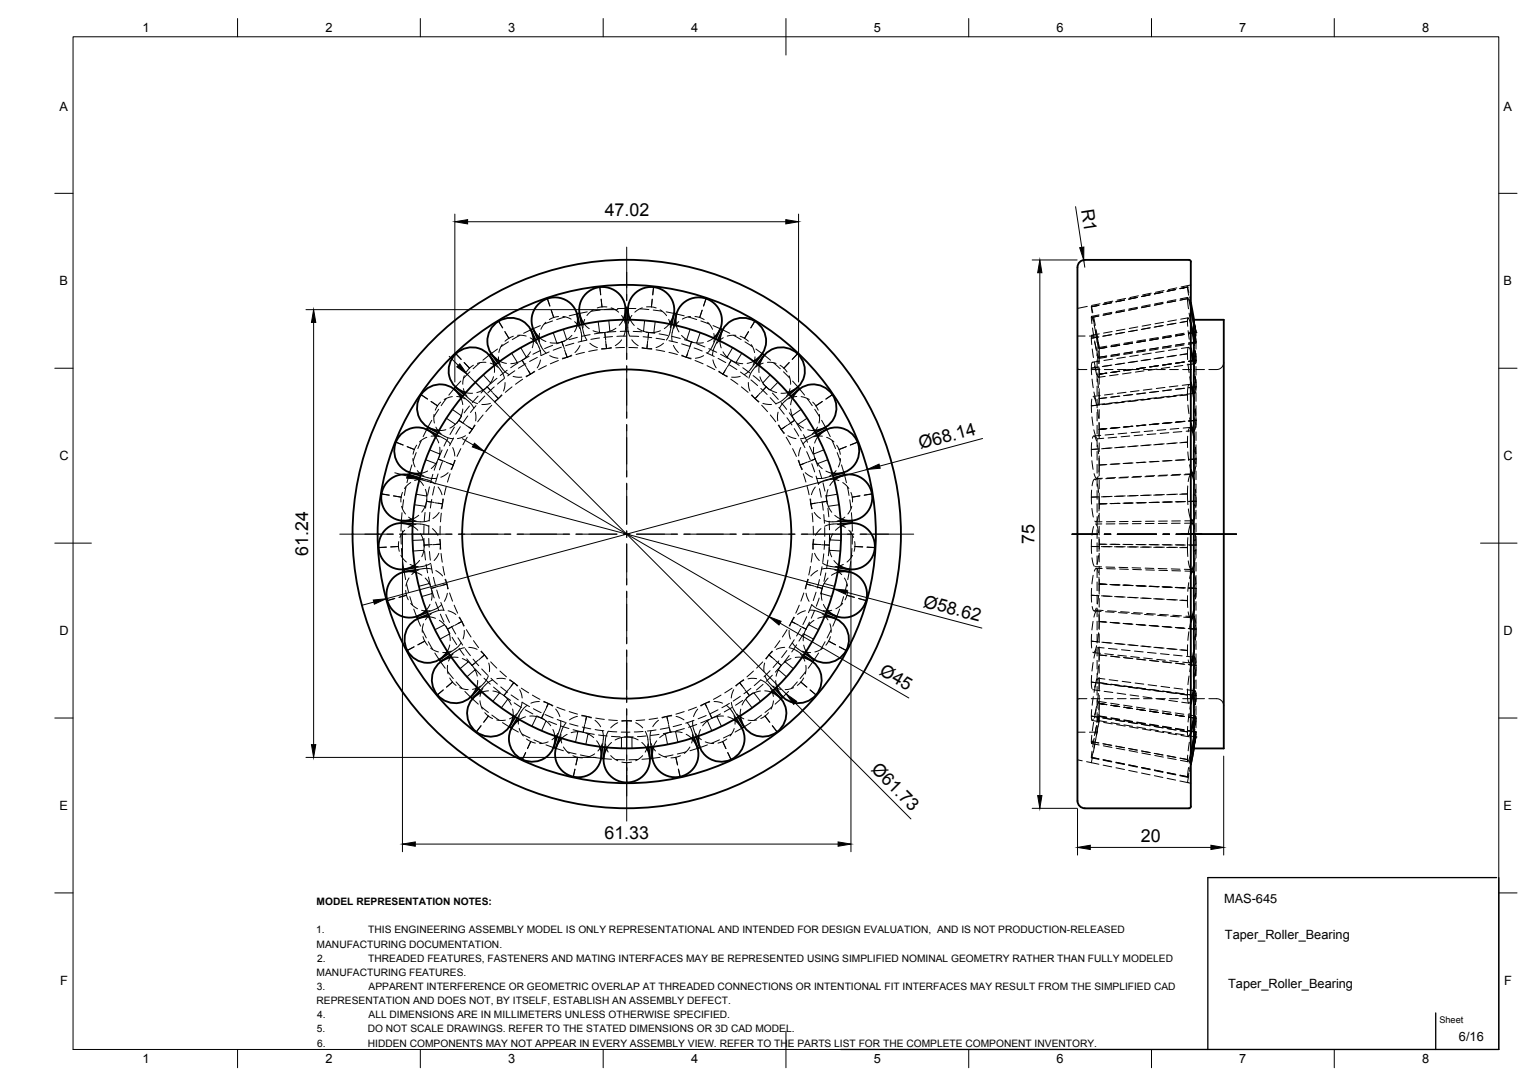
ISO-10303-21;
HEADER;
FILE_DESCRIPTION((''),'2;1');
FILE_NAME('Taper_Roller_Bearing.step','2026-10-09T10:54:55-07:00',(''),(''),'','','');
FILE_SCHEMA (('AUTOMOTIVE_DESIGN { 1 0 10303 214 3 1 1 }'));
ENDSEC;
DATA;
#10=MECHANICAL_DESIGN_GEOMETRIC_PRESENTATION_REPRESENTATION('',(#606),#63824);
#79=TOROIDAL_SURFACE('',#17489,23.5,1.) ;
#80=TOROIDAL_SURFACE('',#17493,36.5,1.) ;
#81=TOROIDAL_SURFACE('',#17497,37.25,0.25) ;
#82=TOROIDAL_SURFACE('',#17503,22.75,0.249999999999998) ;
#99=ELLIPSE('',#17336,29.1332609148258,28.6226076794831) ;
#100=ELLIPSE('',#17338,29.1332609148259,28.622607679483) ;
#101=ELLIPSE('',#17340,29.133260914826,28.6226076794829) ;
#102=ELLIPSE('',#17342,29.1332609148258,28.622607679483) ;
#103=ELLIPSE('',#17344,29.1332609148258,28.6226076794831) ;
#104=ELLIPSE('',#17346,29.1332609148257,28.6226076794832) ;
#105=ELLIPSE('',#17348,29.133260914826,28.6226076794829) ;
#106=ELLIPSE('',#17350,29.1332609148257,28.6226076794832) ;
#107=ELLIPSE('',#17353,29.1332609148258,28.622607679483) ;
#108=ELLIPSE('',#17355,29.1332609148257,28.6226076794832) ;
#109=ELLIPSE('',#17357,29.1332609148255,28.6226076794833) ;
#110=ELLIPSE('',#17359,29.1332609148258,28.6226076794831) ;
#111=ELLIPSE('',#17362,29.1332609148257,28.6226076794832) ;
#112=ELLIPSE('',#17364,29.1332609148257,28.6226076794831) ;
#113=ELLIPSE('',#17366,29.1332609148259,28.622607679483) ;
#114=ELLIPSE('',#17368,29.1332609148258,28.6226076794831) ;
#115=ELLIPSE('',#17370,29.1332609148257,28.6226076794831) ;
#116=ELLIPSE('',#17372,29.1332609148258,28.6226076794831) ;
#117=ELLIPSE('',#17374,29.1332609148258,28.6226076794831) ;
#118=ELLIPSE('',#17376,29.1332609148258,28.6226076794831) ;
#119=ELLIPSE('',#17378,29.1332609148259,28.622607679483) ;
#120=ELLIPSE('',#17380,29.1332609148258,28.622607679483) ;
#121=ELLIPSE('',#17382,29.1332609148258,28.6226076794831) ;
#122=ELLIPSE('',#17384,29.1332609148258,28.622607679483) ;
#123=ELLIPSE('',#17386,29.1332609148258,28.6226076794831) ;
#124=ELLIPSE('',#17388,29.1332609148258,28.6226076794831) ;
#125=ELLIPSE('',#17390,29.1332609148258,28.6226076794831) ;
#126=ELLIPSE('',#17392,29.1332609148258,28.6226076794831) ;
#127=ELLIPSE('',#17393,29.1332609148257,28.6226076794832) ;
#128=ELLIPSE('',#17395,29.8160190680257,29.3077933083081) ;
#129=ELLIPSE('',#17396,29.8160190680257,29.3077933083081) ;
#130=ELLIPSE('',#17397,29.8160190680257,29.3077933083081) ;
#131=ELLIPSE('',#17398,29.8160190680257,29.3077933083081) ;
#132=ELLIPSE('',#17399,29.8160190680257,29.3077933083081) ;
#133=ELLIPSE('',#17400,29.8160190680257,29.3077933083081) ;
#134=ELLIPSE('',#17401,29.8160190680257,29.3077933083081) ;
#135=ELLIPSE('',#17402,29.8160190680257,29.3077933083081) ;
#136=ELLIPSE('',#17403,29.8160190680257,29.3077933083081) ;
#137=ELLIPSE('',#17404,29.8160190680257,29.3077933083081) ;
#138=ELLIPSE('',#17405,29.8160190680257,29.3077933083081) ;
#139=ELLIPSE('',#17406,29.8160190680257,29.3077933083081) ;
#140=ELLIPSE('',#17407,29.8160190680257,29.3077933083081) ;
#141=ELLIPSE('',#17408,29.8160190680257,29.3077933083081) ;
#142=ELLIPSE('',#17409,29.8160190680257,29.3077933083081) ;
#143=ELLIPSE('',#17410,29.8160190680257,29.3077933083081) ;
#144=ELLIPSE('',#17411,29.8160190680257,29.3077933083081) ;
#145=ELLIPSE('',#17412,29.8160190680257,29.3077933083081) ;
#146=ELLIPSE('',#17413,29.8160190680257,29.3077933083081) ;
#147=ELLIPSE('',#17414,29.8160190680257,29.3077933083081) ;
#148=ELLIPSE('',#17415,29.8160190680257,29.3077933083081) ;
#149=ELLIPSE('',#17416,29.8160190680257,29.3077933083081) ;
#150=ELLIPSE('',#17417,29.8160190680257,29.3077933083081) ;
#151=ELLIPSE('',#17418,29.8160190680257,29.3077933083081) ;
#152=ELLIPSE('',#17419,29.8160190680257,29.3077933083081) ;
#153=ELLIPSE('',#17420,29.8160190680257,29.3077933083081) ;
#154=ELLIPSE('',#17421,29.8160190680257,29.3077933083082) ;
#155=ELLIPSE('',#17422,29.8160190680257,29.3077933083082) ;
#156=ELLIPSE('',#17423,29.8160190680257,29.3077933083082) ;
#157=ELLIPSE('',#17424,29.8160190680257,29.3077933083082) ;
#158=ELLIPSE('',#17425,29.8160190680257,29.3077933083081) ;
#159=ELLIPSE('',#17426,29.8160190680257,29.3077933083081) ;
#160=ELLIPSE('',#17427,29.8160190680257,29.3077933083081) ;
#161=ELLIPSE('',#17428,29.8160190680257,29.3077933083081) ;
#162=ELLIPSE('',#17429,29.8160190680257,29.3077933083081) ;
#163=ELLIPSE('',#17430,29.8160190680257,29.3077933083081) ;
#164=ELLIPSE('',#17431,29.8160190680257,29.3077933083081) ;
#165=ELLIPSE('',#17432,29.8160190680257,29.3077933083081) ;
#166=ELLIPSE('',#17433,29.8160190680257,29.3077933083081) ;
#167=ELLIPSE('',#17434,29.8160190680257,29.3077933083081) ;
#168=ELLIPSE('',#17435,29.8160190680257,29.3077933083082) ;
#169=ELLIPSE('',#17436,29.8160190680257,29.3077933083082) ;
#170=ELLIPSE('',#17437,29.8160190680257,29.3077933083081) ;
#171=ELLIPSE('',#17438,29.8160190680257,29.3077933083081) ;
#172=ELLIPSE('',#17439,29.8160190680257,29.3077933083081) ;
#173=ELLIPSE('',#17440,29.8160190680257,29.3077933083081) ;
#174=ELLIPSE('',#17441,29.8160190680257,29.3077933083081) ;
#175=ELLIPSE('',#17442,29.8160190680257,29.3077933083081) ;
#176=ELLIPSE('',#17443,29.8160190680257,29.3077933083081) ;
#177=ELLIPSE('',#17444,29.8160190680257,29.3077933083081) ;
#178=ELLIPSE('',#17445,29.8160190680257,29.3077933083081) ;
#179=ELLIPSE('',#17446,29.8160190680257,29.3077933083081) ;
#180=ELLIPSE('',#17447,29.8160190680257,29.3077933083081) ;
#181=ELLIPSE('',#17448,29.8160190680257,29.3077933083081) ;
#182=ELLIPSE('',#17449,29.8160190680257,29.3077933083082) ;
#183=ELLIPSE('',#17450,29.8160190680257,29.3077933083082) ;
#184=ELLIPSE('',#17451,29.8160190680257,29.3077933083081) ;
#185=ELLIPSE('',#17452,29.8160190680257,29.3077933083081) ;
#186=ELLIPSE('',#17457,35.9515371622909,35.3123204328217) ;
#187=ELLIPSE('',#17458,35.9515371622912,35.3123204328215) ;
#188=ELLIPSE('',#17459,35.9515371622912,35.3123204328215) ;
#189=ELLIPSE('',#17460,35.9515371622913,35.3123204328214) ;
#190=ELLIPSE('',#17461,35.951537162291,35.3123204328217) ;
#191=ELLIPSE('',#17462,35.9515371622911,35.3123204328216) ;
#192=ELLIPSE('',#17463,35.9515371622911,35.3123204328216) ;
#193=ELLIPSE('',#17464,35.9515371622911,35.3123204328216) ;
#194=ELLIPSE('',#17465,35.9515371622913,35.3123204328214) ;
#195=ELLIPSE('',#17466,35.951537162291,35.3123204328217) ;
#196=ELLIPSE('',#17467,35.9515371622912,35.3123204328215) ;
#197=ELLIPSE('',#17468,35.9515371622911,35.3123204328216) ;
#198=ELLIPSE('',#17469,35.951537162291,35.3123204328217) ;
#199=ELLIPSE('',#17470,35.9515371622913,35.3123204328214) ;
#200=ELLIPSE('',#17471,35.951537162291,35.3123204328217) ;
#201=ELLIPSE('',#17472,35.951537162291,35.3123204328217) ;
#202=ELLIPSE('',#17473,35.9515371622912,35.3123204328215) ;
#203=ELLIPSE('',#17474,35.9515371622911,35.3123204328216) ;
#204=ELLIPSE('',#17475,35.9515371622911,35.3123204328216) ;
#205=ELLIPSE('',#17476,35.951537162291,35.3123204328217) ;
#206=ELLIPSE('',#17477,35.9515371622911,35.3123204328215) ;
#207=ELLIPSE('',#17478,35.9515371622911,35.3123204328216) ;
#208=ELLIPSE('',#17479,35.9515371622913,35.3123204328214) ;
#209=ELLIPSE('',#17480,35.9515371622912,35.3123204328215) ;
#210=ELLIPSE('',#17481,35.951537162291,35.3123204328217) ;
#211=ELLIPSE('',#17482,35.9515371622911,35.3123204328216) ;
#212=ELLIPSE('',#17483,35.9515371622913,35.3123204328214) ;
#213=ELLIPSE('',#17484,35.9515371622912,35.3123204328215) ;
#214=ELLIPSE('',#17485,35.9515371622911,35.3123204328216) ;
#333=B_SPLINE_CURVE_WITH_KNOTS('',3,(#53886,#53887,#53888,#53889,#53890,
#53891,#53892,#53893,#53894,#53895,#53896,#53897,#53898,#53899,#53900,#53901,
#53902,#53903,#53904,#53905,#53906,#53907,#53908,#53909,#53910,#53911,#53912,
#53913,#53914,#53915,#53916,#53917,#53918,#53919,#53920,#53921,#53922,#53923,
#53924,#53925),.UNSPECIFIED.,.F.,.F.,(4,3,3,3,3,3,3,3,3,3,3,3,3,4),(1.39920553665769,
1.60174184009255,1.6712576734102,1.86788901812265,2.06612241242195,2.22834356454693,
2.4268269574145,2.62368336398366,2.78544130230508,2.98797174735918,3.19010175291755,
3.34253904006323,3.55341784507492,3.76429664997047),.UNSPECIFIED.) ;
#334=B_SPLINE_CURVE_WITH_KNOTS('',2,(#53927,#53928,#53929),
 .UNSPECIFIED.,.F.,.F.,(3,3),(0.,1.505093859451),.UNSPECIFIED.) ;
#335=B_SPLINE_CURVE_WITH_KNOTS('',2,(#53933,#53934,#53935),
 .UNSPECIFIED.,.F.,.F.,(3,3),(0.0815875964935672,1.58668145590164),
 .UNSPECIFIED.) ;
#336=B_SPLINE_CURVE_WITH_KNOTS('',3,(#53937,#53938,#53939,#53940,#53941,
#53942,#53943,#53944,#53945,#53946,#53947,#53948,#53949,#53950,#53951,#53952,
#53953,#53954,#53955,#53956,#53957,#53958,#53959,#53960,#53961,#53962,#53963,
#53964,#53965,#53966,#53967,#53968,#53969,#53970,#53971,#53972,#53973,#53974,
#53975,#53976),.UNSPECIFIED.,.F.,.F.,(4,3,3,3,3,3,3,3,3,3,3,3,3,4),(5.14917238118853,
5.36005118608411,5.57092999109581,5.77298643029957,5.97546031432194,6.12802772885396,
6.32462027006988,6.52281590231075,6.68512546661211,6.88364627198794,7.08054113574276,
7.24221135774884,7.44474766118475,7.51426349450141),.UNSPECIFIED.) ;
#337=B_SPLINE_CURVE_WITH_KNOTS('',3,(#53980,#53981,#53982,#53983,#53984,
#53985,#53986,#53987,#53988,#53989,#53990,#53991,#53992,#53993,#53994,#53995,
#53996,#53997,#53998,#53999,#54000,#54001,#54002,#54003,#54004,#54005,#54006,
#54007,#54008,#54009,#54010,#54011,#54012,#54013,#54014,#54015,#54016,#54017,
#54018,#54019),.UNSPECIFIED.,.F.,.F.,(4,3,3,3,3,3,3,3,3,3,3,3,3,4),(1.3992055473476,
1.60174185079187,1.6712576734102,1.86788901812146,2.06612241241944,2.22834356454693,
2.42682695741341,2.62368336398125,2.78544130230507,2.98797174735946,3.19010175291812,
3.34253904006322,3.55341784507436,3.76429664996946),.UNSPECIFIED.) ;
#338=B_SPLINE_CURVE_WITH_KNOTS('',2,(#54021,#54022,#54023),
 .UNSPECIFIED.,.F.,.F.,(3,3),(0.,1.50509385964352),.UNSPECIFIED.) ;
#339=B_SPLINE_CURVE_WITH_KNOTS('',2,(#54027,#54028,#54029),
 .UNSPECIFIED.,.F.,.F.,(3,3),(0.0815875959280614,1.58668145590161),
 .UNSPECIFIED.) ;
#340=B_SPLINE_CURVE_WITH_KNOTS('',3,(#54031,#54032,#54033,#54034,#54035,
#54036,#54037,#54038,#54039,#54040,#54041,#54042,#54043,#54044,#54045,#54046,
#54047,#54048,#54049,#54050,#54051,#54052,#54053,#54054,#54055,#54056,#54057,
#54058,#54059,#54060,#54061,#54062,#54063,#54064,#54065,#54066,#54067,#54068,
#54069,#54070),.UNSPECIFIED.,.F.,.F.,(4,3,3,3,3,3,3,3,3,3,3,3,3,4),(5.14917238118934,
5.36005118608456,5.57092999109581,5.77298643030027,5.97546031432337,6.12802772885396,
6.32462027007005,6.52281590231107,6.6851254666121,6.88364627198753,7.08054113574224,
7.24221135774884,7.44474766119323,7.51426348381142),.UNSPECIFIED.) ;
#341=B_SPLINE_CURVE_WITH_KNOTS('',3,(#54074,#54075,#54076,#54077,#54078,
#54079,#54080,#54081,#54082,#54083,#54084,#54085,#54086,#54087,#54088,#54089,
#54090,#54091,#54092,#54093,#54094,#54095,#54096,#54097,#54098,#54099,#54100,
#54101,#54102,#54103,#54104,#54105,#54106,#54107,#54108,#54109,#54110,#54111,
#54112,#54113),.UNSPECIFIED.,.F.,.F.,(4,3,3,3,3,3,3,3,3,3,3,3,3,4),(1.39920580594633,
1.60174210962102,1.6712576734102,1.86788901812167,2.06612241242011,2.22834356454693,
2.42682695741379,2.62368336398277,2.78544130230507,2.9879717473613,3.19010175292116,
3.34253904006322,3.55341784507367,3.76429664996785),.UNSPECIFIED.) ;
#342=B_SPLINE_CURVE_WITH_KNOTS('',2,(#54115,#54116,#54117),
 .UNSPECIFIED.,.F.,.F.,(3,3),(0.,1.50509385929303),.UNSPECIFIED.) ;
#343=B_SPLINE_CURVE_WITH_KNOTS('',2,(#54121,#54122,#54123),
 .UNSPECIFIED.,.F.,.F.,(3,3),(0.0815875965016897,1.5866814559016),
 .UNSPECIFIED.) ;
#344=B_SPLINE_CURVE_WITH_KNOTS('',3,(#54125,#54126,#54127,#54128,#54129,
#54130,#54131,#54132,#54133,#54134,#54135,#54136,#54137,#54138,#54139,#54140,
#54141,#54142,#54143,#54144,#54145,#54146,#54147,#54148,#54149,#54150,#54151,
#54152,#54153,#54154,#54155,#54156,#54157,#54158,#54159,#54160,#54161,#54162,
#54163,#54164),.UNSPECIFIED.,.F.,.F.,(4,3,3,3,3,3,3,3,3,3,3,3,3,4),(5.14917238119121,
5.36005118608542,5.57092999109581,5.77298643029801,5.97546031431876,6.12802772885396,
6.32462027007008,6.52281590231108,6.6851254666121,6.8836462719899,7.08054113574684,
7.24221135774884,7.44474766142535,7.51426322521267),.UNSPECIFIED.) ;
#345=B_SPLINE_CURVE_WITH_KNOTS('',3,(#54168,#54169,#54170,#54171,#54172,
#54173,#54174,#54175,#54176,#54177,#54178,#54179,#54180,#54181,#54182,#54183,
#54184,#54185,#54186,#54187,#54188,#54189,#54190,#54191,#54192,#54193,#54194,
#54195,#54196,#54197,#54198,#54199,#54200,#54201,#54202,#54203,#54204,#54205,
#54206,#54207),.UNSPECIFIED.,.F.,.F.,(4,3,3,3,3,3,3,3,3,3,3,3,3,4),(1.39920578163106,
1.60174208528522,1.67125767341019,1.86788901812004,2.06612241241701,2.22834356454693,
2.42682695741272,2.62368336398046,2.78544130230507,2.98797174735873,3.19010175291722,
3.34253904006322,3.55341784507366,3.76429664996792),.UNSPECIFIED.) ;
#346=B_SPLINE_CURVE_WITH_KNOTS('',2,(#54209,#54210,#54211),
 .UNSPECIFIED.,.F.,.F.,(3,3),(0.,1.50509385916676),.UNSPECIFIED.) ;
#347=B_SPLINE_CURVE_WITH_KNOTS('',2,(#54215,#54216,#54217),
 .UNSPECIFIED.,.F.,.F.,(3,3),(0.0815875966396183,1.58668145590158),
 .UNSPECIFIED.) ;
#348=B_SPLINE_CURVE_WITH_KNOTS('',3,(#54219,#54220,#54221,#54222,#54223,
#54224,#54225,#54226,#54227,#54228,#54229,#54230,#54231,#54232,#54233,#54234,
#54235,#54236,#54237,#54238,#54239,#54240,#54241,#54242,#54243,#54244,#54245,
#54246,#54247,#54248,#54249,#54250,#54251,#54252,#54253,#54254,#54255,#54256,
#54257,#54258),.UNSPECIFIED.,.F.,.F.,(4,3,3,3,3,3,3,3,3,3,3,3,3,4),(5.14917238119099,
5.36005118608529,5.57092999109581,5.77298643030054,5.97546031432383,6.12802772885395,
6.32462027006874,6.52281590230857,6.6851254666121,6.883646271988,7.08054113574284,
7.24221135774883,7.44474766140413,7.51426324952797),.UNSPECIFIED.) ;
#349=B_SPLINE_CURVE_WITH_KNOTS('',3,(#54262,#54263,#54264,#54265,#54266,
#54267,#54268,#54269,#54270,#54271,#54272,#54273,#54274,#54275,#54276,#54277,
#54278,#54279,#54280,#54281,#54282,#54283,#54284,#54285,#54286,#54287,#54288,
#54289,#54290,#54291,#54292,#54293,#54294,#54295,#54296,#54297,#54298,#54299,
#54300,#54301),.UNSPECIFIED.,.F.,.F.,(4,3,3,3,3,3,3,3,3,3,3,3,3,4),(1.39920580297369,
1.60174210664721,1.6712576734102,1.86788901812216,2.06612241242095,2.22834356454693,
2.42682695741258,2.62368336398087,2.78544130230508,2.98797174735879,3.19010175291683,
3.34253904006322,3.55341784507441,3.76429664996957),.UNSPECIFIED.) ;
#350=B_SPLINE_CURVE_WITH_KNOTS('',2,(#54303,#54304,#54305),
 .UNSPECIFIED.,.F.,.F.,(3,3),(0.,1.50509385957502),.UNSPECIFIED.) ;
#351=B_SPLINE_CURVE_WITH_KNOTS('',2,(#54309,#54310,#54311),
 .UNSPECIFIED.,.F.,.F.,(3,3),(0.0815875964292831,1.58668145590159),
 .UNSPECIFIED.) ;
#352=B_SPLINE_CURVE_WITH_KNOTS('',3,(#54313,#54314,#54315,#54316,#54317,
#54318,#54319,#54320,#54321,#54322,#54323,#54324,#54325,#54326,#54327,#54328,
#54329,#54330,#54331,#54332,#54333,#54334,#54335,#54336,#54337,#54338,#54339,
#54340,#54341,#54342,#54343,#54344,#54345,#54346,#54347,#54348,#54349,#54350,
#54351,#54352),.UNSPECIFIED.,.F.,.F.,(4,3,3,3,3,3,3,3,3,3,3,3,3,4),(5.14917238118972,
5.36005118608478,5.57092999109581,5.77298643029918,5.97546031432131,6.12802772885395,
6.32462027006936,6.52281590230965,6.6851254666121,6.88364627198904,7.08054113574454,
7.24221135774883,7.44474766142377,7.51426322818532),.UNSPECIFIED.) ;
#353=B_SPLINE_CURVE_WITH_KNOTS('',3,(#54356,#54357,#54358,#54359,#54360,
#54361,#54362,#54363,#54364,#54365,#54366,#54367,#54368,#54369,#54370,#54371,
#54372,#54373,#54374,#54375,#54376,#54377,#54378,#54379,#54380,#54381,#54382,
#54383,#54384,#54385,#54386,#54387,#54388,#54389,#54390,#54391,#54392,#54393,
#54394,#54395),.UNSPECIFIED.,.F.,.F.,(4,3,3,3,3,3,3,3,3,3,3,3,3,4),(1.39920556389945,
1.60174186735948,1.67125767341019,1.86788901812192,2.06612241242117,2.22834356454693,
2.426826957414,2.62368336398261,2.78544130230507,2.98797174735794,3.1901017529155,
3.34253904006322,3.55341784507408,3.76429664996891),.UNSPECIFIED.) ;
#354=B_SPLINE_CURVE_WITH_KNOTS('',2,(#54397,#54398,#54399),
 .UNSPECIFIED.,.F.,.F.,(3,3),(0.,1.50509385942592),.UNSPECIFIED.) ;
#355=B_SPLINE_CURVE_WITH_KNOTS('',2,(#54403,#54404,#54405),
 .UNSPECIFIED.,.F.,.F.,(3,3),(0.0815875963862985,1.5866814559016),
 .UNSPECIFIED.) ;
#356=B_SPLINE_CURVE_WITH_KNOTS('',3,(#54407,#54408,#54409,#54410,#54411,
#54412,#54413,#54414,#54415,#54416,#54417,#54418,#54419,#54420,#54421,#54422,
#54423,#54424,#54425,#54426,#54427,#54428,#54429,#54430,#54431,#54432,#54433,
#54434,#54435,#54436,#54437,#54438,#54439,#54440,#54441,#54442,#54443,#54444,
#54445,#54446),.UNSPECIFIED.,.F.,.F.,(4,3,3,3,3,3,3,3,3,3,3,3,3,4),(5.14917238118991,
5.36005118608483,5.57092999109581,5.77298643030024,5.97546031432328,6.12802772885395,
6.32462027006993,6.52281590231083,6.6851254666121,6.88364627199045,7.0805411357475,
7.24221135774883,7.44474766121079,7.51426346725949),.UNSPECIFIED.) ;
#357=B_SPLINE_CURVE_WITH_KNOTS('',3,(#54450,#54451,#54452,#54453,#54454,
#54455,#54456,#54457,#54458,#54459,#54460,#54461,#54462,#54463,#54464,#54465,
#54466,#54467,#54468,#54469,#54470,#54471,#54472,#54473,#54474,#54475,#54476,
#54477,#54478,#54479,#54480,#54481,#54482,#54483,#54484,#54485,#54486,#54487,
#54488,#54489),.UNSPECIFIED.,.F.,.F.,(4,3,3,3,3,3,3,3,3,3,3,3,3,4),(1.39920553665765,
1.60174184009286,1.6712576734102,1.86788901812204,2.06612241242079,2.22834356454693,
2.42682695741453,2.62368336398352,2.78544130230508,2.98797174736053,3.19010175291979,
3.34253904006323,3.55341784507441,3.76429664996951),.UNSPECIFIED.) ;
#358=B_SPLINE_CURVE_WITH_KNOTS('',2,(#54491,#54492,#54493),
 .UNSPECIFIED.,.F.,.F.,(3,3),(0.,1.50509385956687),.UNSPECIFIED.) ;
#359=B_SPLINE_CURVE_WITH_KNOTS('',2,(#54497,#54498,#54499),
 .UNSPECIFIED.,.F.,.F.,(3,3),(0.0815875965308134,1.58668145590159),
 .UNSPECIFIED.) ;
#360=B_SPLINE_CURVE_WITH_KNOTS('',3,(#54501,#54502,#54503,#54504,#54505,
#54506,#54507,#54508,#54509,#54510,#54511,#54512,#54513,#54514,#54515,#54516,
#54517,#54518,#54519,#54520,#54521,#54522,#54523,#54524,#54525,#54526,#54527,
#54528,#54529,#54530,#54531,#54532,#54533,#54534,#54535,#54536,#54537,#54538,
#54539,#54540),.UNSPECIFIED.,.F.,.F.,(4,3,3,3,3,3,3,3,3,3,3,3,3,4),(5.14917238118966,
5.36005118608471,5.57092999109581,5.77298643029994,5.9754603143227,6.12802772885396,
6.32462027006873,6.5228159023084,6.6851254666121,6.88364627198617,7.0805411357391,
7.24221135774884,7.44474766118404,7.51426349450139),.UNSPECIFIED.) ;
#361=B_SPLINE_CURVE_WITH_KNOTS('',3,(#54544,#54545,#54546,#54547,#54548,
#54549,#54550,#54551,#54552,#54553,#54554,#54555,#54556,#54557,#54558,#54559,
#54560,#54561,#54562,#54563,#54564,#54565,#54566,#54567,#54568,#54569,#54570,
#54571,#54572,#54573,#54574,#54575,#54576,#54577,#54578,#54579,#54580,#54581,
#54582,#54583),.UNSPECIFIED.,.F.,.F.,(4,3,3,3,3,3,3,3,3,3,3,3,3,4),(1.39920553665761,
1.60174184009247,1.6712576734102,1.86788901812121,2.06612241241882,2.22834356454693,
2.42682695741519,2.62368336398565,2.78544130230508,2.98797174735976,3.1901017529189,
3.34253904006323,3.55341784507426,3.76429664996931),.UNSPECIFIED.) ;
#362=B_SPLINE_CURVE_WITH_KNOTS('',2,(#54585,#54586,#54587),
 .UNSPECIFIED.,.F.,.F.,(3,3),(0.,1.50509385941839),.UNSPECIFIED.) ;
#363=B_SPLINE_CURVE_WITH_KNOTS('',2,(#54591,#54592,#54593),
 .UNSPECIFIED.,.F.,.F.,(3,3),(0.081587596231324,1.5866814559016),
 .UNSPECIFIED.) ;
#364=B_SPLINE_CURVE_WITH_KNOTS('',3,(#54595,#54596,#54597,#54598,#54599,
#54600,#54601,#54602,#54603,#54604,#54605,#54606,#54607,#54608,#54609,#54610,
#54611,#54612,#54613,#54614,#54615,#54616,#54617,#54618,#54619,#54620,#54621,
#54622,#54623,#54624,#54625,#54626,#54627,#54628,#54629,#54630,#54631,#54632,
#54633,#54634),.UNSPECIFIED.,.F.,.F.,(4,3,3,3,3,3,3,3,3,3,3,3,3,4),(5.14917238118963,
5.36005118608472,5.57092999109581,5.77298643030019,5.97546031432334,6.12802772885396,
6.32462027006835,6.52281590230765,6.68512546661211,6.88364627198795,7.08054113574254,
7.24221135774884,7.4447476611839,7.51426349450141),.UNSPECIFIED.) ;
#365=B_SPLINE_CURVE_WITH_KNOTS('',3,(#54638,#54639,#54640,#54641,#54642,
#54643,#54644,#54645,#54646,#54647,#54648,#54649,#54650,#54651,#54652,#54653,
#54654,#54655,#54656,#54657,#54658,#54659,#54660,#54661,#54662,#54663,#54664,
#54665,#54666,#54667,#54668,#54669,#54670,#54671,#54672,#54673,#54674,#54675,
#54676,#54677),.UNSPECIFIED.,.F.,.F.,(4,3,3,3,3,3,3,3,3,3,3,3,3,4),(1.39920577957092,
1.60174208322376,1.6712576734102,1.86788901812092,2.06612241241852,2.22834356454693,
2.42682695741545,2.62368336398506,2.78544130230508,2.98797174736192,3.19010175292271,
3.34253904006322,3.55341784507434,3.76429664996941),.UNSPECIFIED.) ;
#366=B_SPLINE_CURVE_WITH_KNOTS('',2,(#54679,#54680,#54681),
 .UNSPECIFIED.,.F.,.F.,(3,3),(0.,1.50509385951517),.UNSPECIFIED.) ;
#367=B_SPLINE_CURVE_WITH_KNOTS('',2,(#54685,#54686,#54687),
 .UNSPECIFIED.,.F.,.F.,(3,3),(0.0815875965974276,1.58668145590159),
 .UNSPECIFIED.) ;
#368=B_SPLINE_CURVE_WITH_KNOTS('',3,(#54689,#54690,#54691,#54692,#54693,
#54694,#54695,#54696,#54697,#54698,#54699,#54700,#54701,#54702,#54703,#54704,
#54705,#54706,#54707,#54708,#54709,#54710,#54711,#54712,#54713,#54714,#54715,
#54716,#54717,#54718,#54719,#54720,#54721,#54722,#54723,#54724,#54725,#54726,
#54727,#54728),.UNSPECIFIED.,.F.,.F.,(4,3,3,3,3,3,3,3,3,3,3,3,3,4),(5.14917238118954,
5.36005118608465,5.57092999109581,5.77298643029922,5.9754603143212,6.12802772885395,
6.32462027006964,6.52281590231008,6.6851254666121,6.88364627198796,7.0805411357427,
7.24221135774883,7.44474766140348,7.51426325158808),.UNSPECIFIED.) ;
#369=B_SPLINE_CURVE_WITH_KNOTS('',3,(#54732,#54733,#54734,#54735,#54736,
#54737,#54738,#54739,#54740,#54741,#54742,#54743,#54744,#54745,#54746,#54747,
#54748,#54749,#54750,#54751,#54752,#54753,#54754,#54755,#54756,#54757,#54758,
#54759,#54760,#54761,#54762,#54763,#54764,#54765,#54766,#54767,#54768,#54769,
#54770,#54771),.UNSPECIFIED.,.F.,.F.,(4,3,3,3,3,3,3,3,3,3,3,3,3,4),(1.39920575510034,
1.60174205873101,1.6712576734102,1.86788901812208,2.06612241242132,2.22834356454693,
2.42682695741398,2.623683363982,2.78544130230508,2.98797174735979,3.19010175291888,
3.34253904006322,3.55341784507434,3.76429664996953),.UNSPECIFIED.) ;
#370=B_SPLINE_CURVE_WITH_KNOTS('',2,(#54773,#54774,#54775),
 .UNSPECIFIED.,.F.,.F.,(3,3),(0.,1.50509385978829),.UNSPECIFIED.) ;
#371=B_SPLINE_CURVE_WITH_KNOTS('',2,(#54779,#54780,#54781),
 .UNSPECIFIED.,.F.,.F.,(3,3),(0.0815875962064005,1.58668145590161),
 .UNSPECIFIED.) ;
#372=B_SPLINE_CURVE_WITH_KNOTS('',3,(#54783,#54784,#54785,#54786,#54787,
#54788,#54789,#54790,#54791,#54792,#54793,#54794,#54795,#54796,#54797,#54798,
#54799,#54800,#54801,#54802,#54803,#54804,#54805,#54806,#54807,#54808,#54809,
#54810,#54811,#54812,#54813,#54814,#54815,#54816,#54817,#54818,#54819,#54820,
#54821,#54822),.UNSPECIFIED.,.F.,.F.,(4,3,3,3,3,3,3,3,3,3,3,3,3,4),(5.14917238118977,
5.36005118608484,5.57092999109581,5.77298643029907,5.97546031432088,6.12802772885396,
6.32462027006765,6.52281590230627,6.68512546661211,6.88364627198604,7.08054113573874,
7.24221135774884,7.44474766137677,7.51426327605873),.UNSPECIFIED.) ;
#373=B_SPLINE_CURVE_WITH_KNOTS('',3,(#54826,#54827,#54828,#54829,#54830,
#54831,#54832,#54833,#54834,#54835,#54836,#54837,#54838,#54839,#54840,#54841,
#54842,#54843,#54844,#54845,#54846,#54847,#54848,#54849,#54850,#54851,#54852,
#54853,#54854,#54855,#54856,#54857,#54858,#54859,#54860,#54861,#54862,#54863,
#54864,#54865),.UNSPECIFIED.,.F.,.F.,(4,3,3,3,3,3,3,3,3,3,3,3,3,4),(1.39920578522048,
1.60174208887688,1.6712576734102,1.86788901812355,2.06612241242382,2.22834356454693,
2.42682695741664,2.62368336398744,2.78544130230508,2.98797174736012,3.19010175291939,
3.34253904006323,3.55341784507339,3.76429664996726),.UNSPECIFIED.) ;
#374=B_SPLINE_CURVE_WITH_KNOTS('',2,(#54867,#54868,#54869),
 .UNSPECIFIED.,.F.,.F.,(3,3),(0.,1.50509385946946),.UNSPECIFIED.) ;
#375=B_SPLINE_CURVE_WITH_KNOTS('',2,(#54873,#54874,#54875),
 .UNSPECIFIED.,.F.,.F.,(3,3),(0.0815875967998225,1.58668145590156),
 .UNSPECIFIED.) ;
#376=B_SPLINE_CURVE_WITH_KNOTS('',3,(#54877,#54878,#54879,#54880,#54881,
#54882,#54883,#54884,#54885,#54886,#54887,#54888,#54889,#54890,#54891,#54892,
#54893,#54894,#54895,#54896,#54897,#54898,#54899,#54900,#54901,#54902,#54903,
#54904,#54905,#54906,#54907,#54908,#54909,#54910,#54911,#54912,#54913,#54914,
#54915,#54916),.UNSPECIFIED.,.F.,.F.,(4,3,3,3,3,3,3,3,3,3,3,3,3,4),(5.14917238119203,
5.36005118608581,5.57092999109581,5.77298643029689,5.97546031431666,6.12802772885396,
6.32462027006706,6.52281590230514,6.6851254666121,6.88364627198659,7.08054113574006,
7.24221135774884,7.44474766140431,7.51426324593851),.UNSPECIFIED.) ;
#377=B_SPLINE_CURVE_WITH_KNOTS('',3,(#54920,#54921,#54922,#54923,#54924,
#54925,#54926,#54927,#54928,#54929,#54930,#54931,#54932,#54933,#54934,#54935,
#54936,#54937,#54938,#54939,#54940,#54941,#54942,#54943,#54944,#54945,#54946,
#54947,#54948,#54949,#54950,#54951,#54952,#54953,#54954,#54955,#54956,#54957,
#54958,#54959),.UNSPECIFIED.,.F.,.F.,(4,3,3,3,3,3,3,3,3,3,3,3,3,4),(1.39920579236041,
1.6017420960232,1.6712576734102,1.86788901812226,2.06612241242125,2.22834356454693,
2.42682695741395,2.62368336398385,2.78544130230508,2.98797174735984,3.19010175291892,
3.34253904006322,3.55341784507403,3.76429664996856),.UNSPECIFIED.) ;
#378=B_SPLINE_CURVE_WITH_KNOTS('',2,(#54961,#54962,#54963),
 .UNSPECIFIED.,.F.,.F.,(3,3),(0.,1.50509385922266),.UNSPECIFIED.) ;
#379=B_SPLINE_CURVE_WITH_KNOTS('',2,(#54967,#54968,#54969),
 .UNSPECIFIED.,.F.,.F.,(3,3),(0.0815875968142298,1.58668145590157),
 .UNSPECIFIED.) ;
#380=B_SPLINE_CURVE_WITH_KNOTS('',3,(#54971,#54972,#54973,#54974,#54975,
#54976,#54977,#54978,#54979,#54980,#54981,#54982,#54983,#54984,#54985,#54986,
#54987,#54988,#54989,#54990,#54991,#54992,#54993,#54994,#54995,#54996,#54997,
#54998,#54999,#55000,#55001,#55002,#55003,#55004,#55005,#55006,#55007,#55008,
#55009,#55010),.UNSPECIFIED.,.F.,.F.,(4,3,3,3,3,3,3,3,3,3,3,3,3,4),(5.14917238119063,
5.36005118608513,5.57092999109581,5.77298643030012,5.97546031432292,6.12802772885395,
6.32462027007051,6.52281590231203,6.6851254666121,6.8836462719894,7.08054113574546,
7.24221135774883,7.44474766141017,7.51426323879855),.UNSPECIFIED.) ;
#381=B_SPLINE_CURVE_WITH_KNOTS('',3,(#55014,#55015,#55016,#55017,#55018,
#55019,#55020,#55021,#55022,#55023,#55024,#55025,#55026,#55027,#55028,#55029,
#55030,#55031,#55032,#55033,#55034,#55035,#55036,#55037,#55038,#55039,#55040,
#55041,#55042,#55043,#55044,#55045,#55046,#55047,#55048,#55049,#55050,#55051,
#55052,#55053),.UNSPECIFIED.,.F.,.F.,(4,3,3,3,3,3,3,3,3,3,3,3,3,4),(1.39920565780197,
1.6017419613437,1.6712576734102,1.86788901812192,2.06612241242043,2.22834356454693,
2.42682695741329,2.62368336398141,2.78544130230508,2.98797174735931,3.19010175291749,
3.34253904006323,3.5534178450742,3.76429664996896),.UNSPECIFIED.) ;
#382=B_SPLINE_CURVE_WITH_KNOTS('',2,(#55055,#55056,#55057),
 .UNSPECIFIED.,.F.,.F.,(3,3),(0.,1.50509385918315),.UNSPECIFIED.) ;
#383=B_SPLINE_CURVE_WITH_KNOTS('',2,(#55061,#55062,#55063),
 .UNSPECIFIED.,.F.,.F.,(3,3),(0.0815875963175643,1.58668145590161),
 .UNSPECIFIED.) ;
#384=B_SPLINE_CURVE_WITH_KNOTS('',3,(#55065,#55066,#55067,#55068,#55069,
#55070,#55071,#55072,#55073,#55074,#55075,#55076,#55077,#55078,#55079,#55080,
#55081,#55082,#55083,#55084,#55085,#55086,#55087,#55088,#55089,#55090,#55091,
#55092,#55093,#55094,#55095,#55096,#55097,#55098,#55099,#55100,#55101,#55102,
#55103,#55104),.UNSPECIFIED.,.F.,.F.,(4,3,3,3,3,3,3,3,3,3,3,3,3,4),(5.14917238118996,
5.36005118608481,5.57092999109581,5.77298643029938,5.97546031432158,6.12802772885396,
6.32462027006706,6.52281590230528,6.68512546661211,6.88364627198969,7.08054113574575,
7.24221135774884,7.44474766128961,7.51426337335708),.UNSPECIFIED.) ;
#385=B_SPLINE_CURVE_WITH_KNOTS('',3,(#55108,#55109,#55110,#55111,#55112,
#55113,#55114,#55115,#55116,#55117,#55118,#55119,#55120,#55121,#55122,#55123,
#55124,#55125,#55126,#55127,#55128,#55129,#55130,#55131,#55132,#55133,#55134,
#55135,#55136,#55137,#55138,#55139,#55140,#55141,#55142,#55143,#55144,#55145,
#55146,#55147),.UNSPECIFIED.,.F.,.F.,(4,3,3,3,3,3,3,3,3,3,3,3,3,4),(1.39920626730384,
1.60174256547371,1.6712576734102,1.86788901812253,2.06612241242136,2.22834356454693,
2.42682695741533,2.62368336398524,2.78544130230508,2.9879717473591,3.19010175291799,
3.34253904006322,3.55341784507403,3.76429664996862),.UNSPECIFIED.) ;
#386=B_SPLINE_CURVE_WITH_KNOTS('',2,(#55149,#55150,#55151),
 .UNSPECIFIED.,.F.,.F.,(3,3),(0.,1.50509385974731),.UNSPECIFIED.) ;
#387=B_SPLINE_CURVE_WITH_KNOTS('',2,(#55155,#55156,#55157),
 .UNSPECIFIED.,.F.,.F.,(3,3),(0.081587596220629,1.58668145590162),
 .UNSPECIFIED.) ;
#388=B_SPLINE_CURVE_WITH_KNOTS('',3,(#55159,#55160,#55161,#55162,#55163,
#55164,#55165,#55166,#55167,#55168,#55169,#55170,#55171,#55172,#55173,#55174,
#55175,#55176,#55177,#55178,#55179,#55180,#55181,#55182,#55183,#55184,#55185,
#55186,#55187,#55188,#55189,#55190,#55191,#55192,#55193,#55194,#55195,#55196,
#55197,#55198),.UNSPECIFIED.,.F.,.F.,(4,3,3,3,3,3,3,3,3,3,3,3,3,4),(5.14917238119046,
5.36005118608503,5.57092999109581,5.77298643030045,5.97546031432374,6.12802772885396,
6.32462027006966,6.52281590231019,6.6851254666121,6.88364627198813,7.08054113574297,
7.24221135774884,7.44474766183158,7.51426276518474),.UNSPECIFIED.) ;
#389=B_SPLINE_CURVE_WITH_KNOTS('',3,(#55202,#55203,#55204,#55205,#55206,
#55207,#55208,#55209,#55210,#55211,#55212,#55213,#55214,#55215,#55216,#55217,
#55218,#55219,#55220,#55221,#55222,#55223,#55224,#55225,#55226,#55227,#55228,
#55229,#55230,#55231,#55232,#55233,#55234,#55235,#55236,#55237,#55238,#55239,
#55240,#55241),.UNSPECIFIED.,.F.,.F.,(4,3,3,3,3,3,3,3,3,3,3,3,3,4),(1.39920553665763,
1.60174184009342,1.6712576734102,1.86788901812086,2.06612241241843,2.22834356454693,
2.42682695741443,2.62368336398377,2.78544130230508,2.98797174735924,3.19010175291802,
3.34253904006322,3.55341784507355,3.76429664996775),.UNSPECIFIED.) ;
#390=B_SPLINE_CURVE_WITH_KNOTS('',2,(#55243,#55244,#55245),
 .UNSPECIFIED.,.F.,.F.,(3,3),(0.,1.50509385940246),.UNSPECIFIED.) ;
#391=B_SPLINE_CURVE_WITH_KNOTS('',2,(#55249,#55250,#55251),
 .UNSPECIFIED.,.F.,.F.,(3,3),(0.0815875964990715,1.58668145590159),
 .UNSPECIFIED.) ;
#392=B_SPLINE_CURVE_WITH_KNOTS('',3,(#55253,#55254,#55255,#55256,#55257,
#55258,#55259,#55260,#55261,#55262,#55263,#55264,#55265,#55266,#55267,#55268,
#55269,#55270,#55271,#55272,#55273,#55274,#55275,#55276,#55277,#55278,#55279,
#55280,#55281,#55282,#55283,#55284,#55285,#55286,#55287,#55288,#55289,#55290,
#55291,#55292),.UNSPECIFIED.,.F.,.F.,(4,3,3,3,3,3,3,3,3,3,3,3,3,4),(5.14917238119122,
5.36005118608543,5.57092999109581,5.77298643029924,5.97546031432136,6.12802772885395,
6.32462027006939,6.52281590230979,6.6851254666121,6.88364627198772,7.08054113574227,
7.24221135774883,7.44474766118609,7.5142634945014),.UNSPECIFIED.) ;
#393=B_SPLINE_CURVE_WITH_KNOTS('',3,(#55296,#55297,#55298,#55299,#55300,
#55301,#55302,#55303,#55304,#55305,#55306,#55307,#55308,#55309,#55310,#55311,
#55312,#55313,#55314,#55315,#55316,#55317,#55318,#55319,#55320,#55321,#55322,
#55323,#55324,#55325,#55326,#55327,#55328,#55329,#55330,#55331,#55332,#55333,
#55334,#55335),.UNSPECIFIED.,.F.,.F.,(4,3,3,3,3,3,3,3,3,3,3,3,3,4),(1.39920626597427,
1.60174256547503,1.6712576734102,1.86788901812092,2.06612241241852,2.22834356454693,
2.4268269574154,2.62368336398519,2.78544130230508,2.98797174735909,3.19010175291677,
3.34253904006322,3.55341784507445,3.76429664996961),.UNSPECIFIED.) ;
#394=B_SPLINE_CURVE_WITH_KNOTS('',2,(#55337,#55338,#55339),
 .UNSPECIFIED.,.F.,.F.,(3,3),(0.,1.50509385919341),.UNSPECIFIED.) ;
#395=B_SPLINE_CURVE_WITH_KNOTS('',2,(#55343,#55344,#55345),
 .UNSPECIFIED.,.F.,.F.,(3,3),(0.0815875964645715,1.58668145590163),
 .UNSPECIFIED.) ;
#396=B_SPLINE_CURVE_WITH_KNOTS('',3,(#55347,#55348,#55349,#55350,#55351,
#55352,#55353,#55354,#55355,#55356,#55357,#55358,#55359,#55360,#55361,#55362,
#55363,#55364,#55365,#55366,#55367,#55368,#55369,#55370,#55371,#55372,#55373,
#55374,#55375,#55376,#55377,#55378,#55379,#55380,#55381,#55382,#55383,#55384,
#55385,#55386),.UNSPECIFIED.,.F.,.F.,(4,3,3,3,3,3,3,3,3,3,3,3,3,4),(5.14917238118938,
5.36005118608458,5.57092999109581,5.77298643029965,5.97546031432214,6.12802772885396,
6.32462027006888,6.5228159023088,6.6851254666121,6.88364627198861,7.0805411357444,
7.24221135774884,7.44474766183236,7.51426276385522),.UNSPECIFIED.) ;
#397=B_SPLINE_CURVE_WITH_KNOTS('',3,(#55390,#55391,#55392,#55393,#55394,
#55395,#55396,#55397,#55398,#55399,#55400,#55401,#55402,#55403,#55404,#55405,
#55406,#55407,#55408,#55409,#55410,#55411,#55412,#55413,#55414,#55415,#55416,
#55417,#55418,#55419,#55420,#55421,#55422,#55423,#55424,#55425,#55426,#55427,
#55428,#55429),.UNSPECIFIED.,.F.,.F.,(4,3,3,3,3,3,3,3,3,3,3,3,3,4),(1.39920565780197,
1.60174196134636,1.6712576734102,1.86788901812062,2.06612241241771,2.22834356454693,
2.42682695741333,2.62368336398205,2.78544130230508,2.98797174735987,3.19010175291831,
3.34253904006323,3.55341784507432,3.76429664996955),.UNSPECIFIED.) ;
#398=B_SPLINE_CURVE_WITH_KNOTS('',2,(#55431,#55432,#55433),
 .UNSPECIFIED.,.F.,.F.,(3,3),(0.,1.50509385959389),.UNSPECIFIED.) ;
#399=B_SPLINE_CURVE_WITH_KNOTS('',2,(#55437,#55438,#55439),
 .UNSPECIFIED.,.F.,.F.,(3,3),(0.0815875963589051,1.58668145590161),
 .UNSPECIFIED.) ;
#400=B_SPLINE_CURVE_WITH_KNOTS('',3,(#55441,#55442,#55443,#55444,#55445,
#55446,#55447,#55448,#55449,#55450,#55451,#55452,#55453,#55454,#55455,#55456,
#55457,#55458,#55459,#55460,#55461,#55462,#55463,#55464,#55465,#55466,#55467,
#55468,#55469,#55470,#55471,#55472,#55473,#55474,#55475,#55476,#55477,#55478,
#55479,#55480),.UNSPECIFIED.,.F.,.F.,(4,3,3,3,3,3,3,3,3,3,3,3,3,4),(5.1491723811898,
5.36005118608492,5.57092999109581,5.77298643029963,5.97546031432211,6.12802772885396,
6.32462027007047,6.52281590231188,6.6851254666121,6.88364627198989,7.08054113574668,
7.24221135774884,7.44474766129325,7.51426337335708),.UNSPECIFIED.) ;
#401=B_SPLINE_CURVE_WITH_KNOTS('',3,(#55484,#55485,#55486,#55487,#55488,
#55489,#55490,#55491,#55492,#55493,#55494,#55495,#55496,#55497,#55498,#55499,
#55500,#55501,#55502,#55503,#55504,#55505,#55506,#55507,#55508,#55509,#55510,
#55511,#55512,#55513,#55514,#55515,#55516,#55517,#55518,#55519,#55520,#55521,
#55522,#55523),.UNSPECIFIED.,.F.,.F.,(4,3,3,3,3,3,3,3,3,3,3,3,3,4),(1.39920579236047,
1.60174209602461,1.6712576734102,1.86788901812178,2.06612241242039,2.22834356454693,
2.42682695741637,2.6236833639871,2.78544130230507,2.98797174736062,3.1901017529202,
3.34253904006322,3.55341784507431,3.76429664996928),.UNSPECIFIED.) ;
#402=B_SPLINE_CURVE_WITH_KNOTS('',2,(#55525,#55526,#55527),
 .UNSPECIFIED.,.F.,.F.,(3,3),(0.,1.50509385958745),.UNSPECIFIED.) ;
#403=B_SPLINE_CURVE_WITH_KNOTS('',2,(#55531,#55532,#55533),
 .UNSPECIFIED.,.F.,.F.,(3,3),(0.081587596555011,1.58668145590161),
 .UNSPECIFIED.) ;
#404=B_SPLINE_CURVE_WITH_KNOTS('',3,(#55535,#55536,#55537,#55538,#55539,
#55540,#55541,#55542,#55543,#55544,#55545,#55546,#55547,#55548,#55549,#55550,
#55551,#55552,#55553,#55554,#55555,#55556,#55557,#55558,#55559,#55560,#55561,
#55562,#55563,#55564,#55565,#55566,#55567,#55568,#55569,#55570,#55571,#55572,
#55573,#55574),.UNSPECIFIED.,.F.,.F.,(4,3,3,3,3,3,3,3,3,3,3,3,3,4),(5.14917238118991,
5.36005118608479,5.5709299910958,5.77298643029917,5.9754603143211,6.12802772885395,
6.32462027006938,6.5228159023099,6.68512546661209,6.88364627198928,7.08054113574494,
7.24221135774883,7.44474766141436,7.51426323879859),.UNSPECIFIED.) ;
#405=B_SPLINE_CURVE_WITH_KNOTS('',3,(#55578,#55579,#55580,#55581,#55582,
#55583,#55584,#55585,#55586,#55587,#55588,#55589,#55590,#55591,#55592,#55593,
#55594,#55595,#55596,#55597,#55598,#55599,#55600,#55601,#55602,#55603,#55604,
#55605,#55606,#55607,#55608,#55609,#55610,#55611,#55612,#55613,#55614,#55615,
#55616,#55617),.UNSPECIFIED.,.F.,.F.,(4,3,3,3,3,3,3,3,3,3,3,3,3,4),(1.39920578522049,
1.60174208887845,1.6712576734102,1.86788901812191,2.0661224124205,2.22834356454693,
2.42682695741374,2.62368336398196,2.78544130230508,2.98797174736077,3.19010175292072,
3.34253904006322,3.55341784507369,3.76429664996809),.UNSPECIFIED.) ;
#406=B_SPLINE_CURVE_WITH_KNOTS('',2,(#55619,#55620,#55621),
 .UNSPECIFIED.,.F.,.F.,(3,3),(0.,1.50509385994802),.UNSPECIFIED.) ;
#407=B_SPLINE_CURVE_WITH_KNOTS('',2,(#55625,#55626,#55627),
 .UNSPECIFIED.,.F.,.F.,(3,3),(0.0815875960578148,1.58668145590161),
 .UNSPECIFIED.) ;
#408=B_SPLINE_CURVE_WITH_KNOTS('',3,(#55629,#55630,#55631,#55632,#55633,
#55634,#55635,#55636,#55637,#55638,#55639,#55640,#55641,#55642,#55643,#55644,
#55645,#55646,#55647,#55648,#55649,#55650,#55651,#55652,#55653,#55654,#55655,
#55656,#55657,#55658,#55659,#55660,#55661,#55662,#55663,#55664,#55665,#55666,
#55667,#55668),.UNSPECIFIED.,.F.,.F.,(4,3,3,3,3,3,3,3,3,3,3,3,3,4),(5.14917238119084,
5.36005118608529,5.57092999109581,5.7729864302989,5.97546031432077,6.12802772885396,
6.32462027007018,6.52281590231123,6.6851254666121,6.8836462719878,7.08054113574219,
7.24221135774883,7.44474766140652,7.5142632459385),.UNSPECIFIED.) ;
#409=B_SPLINE_CURVE_WITH_KNOTS('',3,(#55672,#55673,#55674,#55675,#55676,
#55677,#55678,#55679,#55680,#55681,#55682,#55683,#55684,#55685,#55686,#55687,
#55688,#55689,#55690,#55691,#55692,#55693,#55694,#55695,#55696,#55697,#55698,
#55699,#55700,#55701,#55702,#55703,#55704,#55705,#55706,#55707,#55708,#55709,
#55710,#55711),.UNSPECIFIED.,.F.,.F.,(4,3,3,3,3,3,3,3,3,3,3,3,3,4),(1.39920575510034,
1.60174205873404,1.6712576734102,1.86788901812231,2.06612241242113,2.22834356454693,
2.42682695741377,2.62368336398224,2.78544130230507,2.98797174735987,3.1901017529183,
3.34253904006322,3.5534178450742,3.76429664996902),.UNSPECIFIED.) ;
#410=B_SPLINE_CURVE_WITH_KNOTS('',2,(#55713,#55714,#55715),
 .UNSPECIFIED.,.F.,.F.,(3,3),(0.,1.50509385928664),.UNSPECIFIED.) ;
#411=B_SPLINE_CURVE_WITH_KNOTS('',2,(#55719,#55720,#55721),
 .UNSPECIFIED.,.F.,.F.,(3,3),(0.081587596588401,1.58668145590163),
 .UNSPECIFIED.) ;
#412=B_SPLINE_CURVE_WITH_KNOTS('',3,(#55723,#55724,#55725,#55726,#55727,
#55728,#55729,#55730,#55731,#55732,#55733,#55734,#55735,#55736,#55737,#55738,
#55739,#55740,#55741,#55742,#55743,#55744,#55745,#55746,#55747,#55748,#55749,
#55750,#55751,#55752,#55753,#55754,#55755,#55756,#55757,#55758,#55759,#55760,
#55761,#55762),.UNSPECIFIED.,.F.,.F.,(4,3,3,3,3,3,3,3,3,3,3,3,3,4),(5.14917238118993,
5.36005118608476,5.57092999109581,5.77298643029968,5.97546031432223,6.12802772885395,
6.32462027006896,6.52281590230873,6.6851254666121,6.88364627198979,7.08054113574599,
7.24221135774883,7.44474766138134,7.51426327605874),.UNSPECIFIED.) ;
#413=B_SPLINE_CURVE_WITH_KNOTS('',3,(#55766,#55767,#55768,#55769,#55770,
#55771,#55772,#55773,#55774,#55775,#55776,#55777,#55778,#55779,#55780,#55781,
#55782,#55783,#55784,#55785,#55786,#55787,#55788,#55789,#55790,#55791,#55792,
#55793,#55794,#55795,#55796,#55797,#55798,#55799,#55800,#55801,#55802,#55803,
#55804,#55805),.UNSPECIFIED.,.F.,.F.,(4,3,3,3,3,3,3,3,3,3,3,3,3,4),(1.39920577957096,
1.60174208322522,1.6712576734102,1.86788901812319,2.06612241242312,2.22834356454693,
2.42682695741511,2.62368336398486,2.78544130230508,2.98797174736008,3.19010175291886,
3.34253904006322,3.5534178450743,3.76429664996913),.UNSPECIFIED.) ;
#414=B_SPLINE_CURVE_WITH_KNOTS('',2,(#55807,#55808,#55809),
 .UNSPECIFIED.,.F.,.F.,(3,3),(0.,1.50509385929993),.UNSPECIFIED.) ;
#415=B_SPLINE_CURVE_WITH_KNOTS('',2,(#55813,#55814,#55815),
 .UNSPECIFIED.,.F.,.F.,(3,3),(0.0815875966725096,1.58668145590163),
 .UNSPECIFIED.) ;
#416=B_SPLINE_CURVE_WITH_KNOTS('',3,(#55817,#55818,#55819,#55820,#55821,
#55822,#55823,#55824,#55825,#55826,#55827,#55828,#55829,#55830,#55831,#55832,
#55833,#55834,#55835,#55836,#55837,#55838,#55839,#55840,#55841,#55842,#55843,
#55844,#55845,#55846,#55847,#55848,#55849,#55850,#55851,#55852,#55853,#55854,
#55855,#55856),.UNSPECIFIED.,.F.,.F.,(4,3,3,3,3,3,3,3,3,3,3,3,3,4),(5.14917238118991,
5.36005118608476,5.57092999109581,5.77298643029882,5.97546031432058,6.12802772885396,
6.32462027006761,6.52281590230618,6.6851254666121,6.88364627199035,7.08054113574733,
7.24221135774884,7.44474766140251,7.51426325158811),.UNSPECIFIED.) ;
#417=B_SPLINE_CURVE_WITH_KNOTS('',3,(#55860,#55861,#55862,#55863,#55864,
#55865,#55866,#55867,#55868,#55869,#55870,#55871,#55872,#55873,#55874,#55875,
#55876,#55877,#55878,#55879,#55880,#55881,#55882,#55883,#55884,#55885,#55886,
#55887,#55888,#55889,#55890,#55891,#55892,#55893,#55894,#55895,#55896,#55897,
#55898,#55899),.UNSPECIFIED.,.F.,.F.,(4,3,3,3,3,3,3,3,3,3,3,3,3,4),(1.39920553665765,
1.60174184009056,1.6712576734102,1.86788901812072,2.06612241241829,2.22834356454694,
2.42682695741387,2.62368336398203,2.78544130230508,2.98797174735976,3.19010175291811,
3.34253904006323,3.55341784507432,3.76429664996928),.UNSPECIFIED.) ;
#418=B_SPLINE_CURVE_WITH_KNOTS('',2,(#55901,#55902,#55903),
 .UNSPECIFIED.,.F.,.F.,(3,3),(0.,1.5050938596919),.UNSPECIFIED.) ;
#419=B_SPLINE_CURVE_WITH_KNOTS('',2,(#55907,#55908,#55909),
 .UNSPECIFIED.,.F.,.F.,(3,3),(0.0815875961098428,1.58668145590164),
 .UNSPECIFIED.) ;
#420=B_SPLINE_CURVE_WITH_KNOTS('',3,(#55911,#55912,#55913,#55914,#55915,
#55916,#55917,#55918,#55919,#55920,#55921,#55922,#55923,#55924,#55925,#55926,
#55927,#55928,#55929,#55930,#55931,#55932,#55933,#55934,#55935,#55936,#55937,
#55938,#55939,#55940,#55941,#55942,#55943,#55944,#55945,#55946,#55947,#55948,
#55949,#55950),.UNSPECIFIED.,.F.,.F.,(4,3,3,3,3,3,3,3,3,3,3,3,3,4),(5.14917238118964,
5.36005118608463,5.57092999109582,5.77298643029978,5.97546031432238,6.12802772885397,
6.32462027006883,6.52281590230841,6.68512546661211,6.88364627198785,7.0805411357423,
7.24221135774884,7.44474766118272,7.51426349450143),.UNSPECIFIED.) ;
#421=B_SPLINE_CURVE_WITH_KNOTS('',3,(#55954,#55955,#55956,#55957,#55958,
#55959,#55960,#55961,#55962,#55963,#55964,#55965,#55966,#55967,#55968,#55969,
#55970,#55971,#55972,#55973,#55974,#55975,#55976,#55977,#55978,#55979,#55980,
#55981,#55982,#55983,#55984,#55985,#55986,#55987,#55988,#55989,#55990,#55991,
#55992,#55993),.UNSPECIFIED.,.F.,.F.,(4,3,3,3,3,3,3,3,3,3,3,3,3,4),(1.39920553665765,
1.60174184009242,1.6712576734102,1.86788901812178,2.0661224124197,2.22834356454693,
2.42682695741288,2.62368336398156,2.78544130230508,2.98797174735984,3.19010175291886,
3.34253904006323,3.55341784507438,3.76429664996941),.UNSPECIFIED.) ;
#422=B_SPLINE_CURVE_WITH_KNOTS('',2,(#55995,#55996,#55997),
 .UNSPECIFIED.,.F.,.F.,(3,3),(0.,1.50509385942888),.UNSPECIFIED.) ;
#423=B_SPLINE_CURVE_WITH_KNOTS('',2,(#56001,#56002,#56003),
 .UNSPECIFIED.,.F.,.F.,(3,3),(0.0815875966181519,1.58668145590164),
 .UNSPECIFIED.) ;
#424=B_SPLINE_CURVE_WITH_KNOTS('',3,(#56005,#56006,#56007,#56008,#56009,
#56010,#56011,#56012,#56013,#56014,#56015,#56016,#56017,#56018,#56019,#56020,
#56021,#56022,#56023,#56024,#56025,#56026,#56027,#56028,#56029,#56030,#56031,
#56032,#56033,#56034,#56035,#56036,#56037,#56038,#56039,#56040,#56041,#56042,
#56043,#56044),.UNSPECIFIED.,.F.,.F.,(4,3,3,3,3,3,3,3,3,3,3,3,3,4),(5.1491723811896,
5.36005118608465,5.57092999109581,5.77298643029993,5.9754603143227,6.12802772885395,
6.32462027006869,6.52281590230835,6.6851254666121,6.88364627198907,7.08054113574468,
7.24221135774883,7.44474766118646,7.51426349450139),.UNSPECIFIED.) ;
#425=B_SPLINE_CURVE_WITH_KNOTS('',3,(#56048,#56049,#56050,#56051,#56052,
#56053,#56054,#56055,#56056,#56057,#56058,#56059,#56060,#56061,#56062,#56063,
#56064,#56065,#56066,#56067,#56068,#56069,#56070,#56071,#56072,#56073,#56074,
#56075,#56076,#56077,#56078,#56079,#56080,#56081,#56082,#56083,#56084,#56085,
#56086,#56087),.UNSPECIFIED.,.F.,.F.,(4,3,3,3,3,3,3,3,3,3,3,3,3,4),(1.39920556389953,
1.60174186736169,1.6712576734102,1.86788901812329,2.06612241242289,2.22834356454693,
2.42682695741632,2.62368336398626,2.78544130230508,2.98797174736086,3.19010175292064,
3.34253904006322,3.55341784507414,3.76429664996872),.UNSPECIFIED.) ;
#426=B_SPLINE_CURVE_WITH_KNOTS('',2,(#56089,#56090,#56091),
 .UNSPECIFIED.,.F.,.F.,(3,3),(0.,1.50509385902892),.UNSPECIFIED.) ;
#427=B_SPLINE_CURVE_WITH_KNOTS('',2,(#56095,#56096,#56097),
 .UNSPECIFIED.,.F.,.F.,(3,3),(0.0815875968459406,1.58668145590164),
 .UNSPECIFIED.) ;
#428=B_SPLINE_CURVE_WITH_KNOTS('',3,(#56099,#56100,#56101,#56102,#56103,
#56104,#56105,#56106,#56107,#56108,#56109,#56110,#56111,#56112,#56113,#56114,
#56115,#56116,#56117,#56118,#56119,#56120,#56121,#56122,#56123,#56124,#56125,
#56126,#56127,#56128,#56129,#56130,#56131,#56132,#56133,#56134,#56135,#56136,
#56137,#56138),.UNSPECIFIED.,.F.,.F.,(4,3,3,3,3,3,3,3,3,3,3,3,3,4),(5.14917238119049,
5.360051186085,5.57092999109581,5.77298643030171,5.97546031432617,6.12802772885396,
6.32462027007144,6.5228159023139,6.6851254666121,6.88364627198961,7.08054113574615,
7.24221135774884,7.44474766120728,7.51426346725953),.UNSPECIFIED.) ;
#429=B_SPLINE_CURVE_WITH_KNOTS('',3,(#56142,#56143,#56144,#56145,#56146,
#56147,#56148,#56149,#56150,#56151,#56152,#56153,#56154,#56155,#56156,#56157,
#56158,#56159,#56160,#56161,#56162,#56163,#56164,#56165,#56166,#56167,#56168,
#56169,#56170,#56171,#56172,#56173,#56174,#56175,#56176,#56177,#56178,#56179,
#56180,#56181),.UNSPECIFIED.,.F.,.F.,(4,3,3,3,3,3,3,3,3,3,3,3,3,4),(1.39920580297372,
1.60174210665031,1.6712576734102,1.86788901812242,2.06612241242141,2.22834356454693,
2.42682695741471,2.6236833639841,2.78544130230508,2.98797174736084,3.19010175292033,
3.34253904006322,3.55341784507415,3.76429664996889),.UNSPECIFIED.) ;
#430=B_SPLINE_CURVE_WITH_KNOTS('',2,(#56183,#56184,#56185),
 .UNSPECIFIED.,.F.,.F.,(3,3),(0.,1.50509385917405),.UNSPECIFIED.) ;
#431=B_SPLINE_CURVE_WITH_KNOTS('',2,(#56189,#56190,#56191),
 .UNSPECIFIED.,.F.,.F.,(3,3),(0.0815875970104741,1.58668145590163),
 .UNSPECIFIED.) ;
#432=B_SPLINE_CURVE_WITH_KNOTS('',3,(#56193,#56194,#56195,#56196,#56197,
#56198,#56199,#56200,#56201,#56202,#56203,#56204,#56205,#56206,#56207,#56208,
#56209,#56210,#56211,#56212,#56213,#56214,#56215,#56216,#56217,#56218,#56219,
#56220,#56221,#56222,#56223,#56224,#56225,#56226,#56227,#56228,#56229,#56230,
#56231,#56232),.UNSPECIFIED.,.F.,.F.,(4,3,3,3,3,3,3,3,3,3,3,3,3,4),(5.14917238118975,
5.36005118608465,5.57092999109581,5.77298643029957,5.97546031432202,6.12802772885396,
6.32462027006847,6.52281590230783,6.6851254666121,6.88364627198963,7.0805411357456,
7.24221135774883,7.44474766142264,7.51426322818531),.UNSPECIFIED.) ;
#433=B_SPLINE_CURVE_WITH_KNOTS('',3,(#56236,#56237,#56238,#56239,#56240,
#56241,#56242,#56243,#56244,#56245,#56246,#56247,#56248,#56249,#56250,#56251,
#56252,#56253,#56254,#56255,#56256,#56257,#56258,#56259,#56260,#56261,#56262,
#56263,#56264,#56265,#56266,#56267,#56268,#56269,#56270,#56271,#56272,#56273,
#56274,#56275),.UNSPECIFIED.,.F.,.F.,(4,3,3,3,3,3,3,3,3,3,3,3,3,4),(1.39920578163109,
1.60174208528961,1.67125767341019,1.86788901812345,2.06612241242393,2.22834356454692,
2.42682695741443,2.62368336398346,2.78544130230507,2.98797174735876,3.1901017529163,
3.34253904006322,3.55341784507393,3.76429664996861),.UNSPECIFIED.) ;
#434=B_SPLINE_CURVE_WITH_KNOTS('',2,(#56277,#56278,#56279),
 .UNSPECIFIED.,.F.,.F.,(3,3),(0.,1.50509385977447),.UNSPECIFIED.) ;
#435=B_SPLINE_CURVE_WITH_KNOTS('',2,(#56283,#56284,#56285),
 .UNSPECIFIED.,.F.,.F.,(3,3),(0.0815875964822538,1.58668145590165),
 .UNSPECIFIED.) ;
#436=B_SPLINE_CURVE_WITH_KNOTS('',3,(#56287,#56288,#56289,#56290,#56291,
#56292,#56293,#56294,#56295,#56296,#56297,#56298,#56299,#56300,#56301,#56302,
#56303,#56304,#56305,#56306,#56307,#56308,#56309,#56310,#56311,#56312,#56313,
#56314,#56315,#56316,#56317,#56318,#56319,#56320,#56321,#56322,#56323,#56324,
#56325,#56326),.UNSPECIFIED.,.F.,.F.,(4,3,3,3,3,3,3,3,3,3,3,3,3,4),(5.14917238119043,
5.36005118608505,5.5709299910958,5.77298643029934,5.97546031432166,6.12802772885395,
6.32462027006776,6.52281590230651,6.6851254666121,6.88364627199062,7.08054113574748,
7.24221135774883,7.44474766140304,7.51426324952791),.UNSPECIFIED.) ;
#437=B_SPLINE_CURVE_WITH_KNOTS('',3,(#56330,#56331,#56332,#56333,#56334,
#56335,#56336,#56337,#56338,#56339,#56340,#56341,#56342,#56343,#56344,#56345,
#56346,#56347,#56348,#56349,#56350,#56351,#56352,#56353,#56354,#56355,#56356,
#56357,#56358,#56359,#56360,#56361,#56362,#56363,#56364,#56365,#56366,#56367,
#56368,#56369),.UNSPECIFIED.,.F.,.F.,(4,3,3,3,3,3,3,3,3,3,3,3,3,4),(1.39920580594635,
1.60174210962213,1.67125767341019,1.86788901812036,2.06612241241732,2.22834356454693,
2.42682695741494,2.62368336398253,2.78544130230507,2.98797174736146,3.1901017529218,
3.34253904006322,3.55341784507419,3.76429664996922),.UNSPECIFIED.) ;
#438=B_SPLINE_CURVE_WITH_KNOTS('',2,(#56371,#56372,#56373),
 .UNSPECIFIED.,.F.,.F.,(3,3),(0.,1.50509385953119),.UNSPECIFIED.) ;
#439=B_SPLINE_CURVE_WITH_KNOTS('',2,(#56377,#56378,#56379),
 .UNSPECIFIED.,.F.,.F.,(3,3),(0.0815875961704467,1.58668145590162),
 .UNSPECIFIED.) ;
#440=B_SPLINE_CURVE_WITH_KNOTS('',3,(#56381,#56382,#56383,#56384,#56385,
#56386,#56387,#56388,#56389,#56390,#56391,#56392,#56393,#56394,#56395,#56396,
#56397,#56398,#56399,#56400,#56401,#56402,#56403,#56404,#56405,#56406,#56407,
#56408,#56409,#56410,#56411,#56412,#56413,#56414,#56415,#56416,#56417,#56418,
#56419,#56420),.UNSPECIFIED.,.F.,.F.,(4,3,3,3,3,3,3,3,3,3,3,3,3,4),(5.14917238118979,
5.3600511860848,5.57092999109581,5.77298643029889,5.97546031432064,6.12802772885396,
6.32462027006939,6.52281590230972,6.6851254666121,6.88364627198858,7.08054113574403,
7.24221135774883,7.44474766142492,7.51426322521266),.UNSPECIFIED.) ;
#441=B_SPLINE_CURVE_WITH_KNOTS('',3,(#56424,#56425,#56426,#56427,#56428,
#56429,#56430,#56431,#56432,#56433,#56434,#56435,#56436,#56437,#56438,#56439,
#56440,#56441,#56442,#56443,#56444,#56445,#56446,#56447,#56448,#56449,#56450,
#56451,#56452,#56453,#56454,#56455,#56456,#56457,#56458,#56459,#56460,#56461,
#56462,#56463),.UNSPECIFIED.,.F.,.F.,(4,3,3,3,3,3,3,3,3,3,3,3,3,4),(1.39920554734762,
1.60174185079261,1.6712576734102,1.86788901812075,2.06612241241815,2.22834356454693,
2.42682695741446,2.62368336398269,2.78544130230508,2.9879717473577,3.19010175291388,
3.34253904006322,3.5534178450744,3.76429664996949),.UNSPECIFIED.) ;
#442=B_SPLINE_CURVE_WITH_KNOTS('',2,(#56465,#56466,#56467),
 .UNSPECIFIED.,.F.,.F.,(3,3),(0.,1.50509385944905),.UNSPECIFIED.) ;
#443=B_SPLINE_CURVE_WITH_KNOTS('',2,(#56471,#56472,#56473),
 .UNSPECIFIED.,.F.,.F.,(3,3),(0.0815875965531534,1.58668145590162),
 .UNSPECIFIED.) ;
#444=B_SPLINE_CURVE_WITH_KNOTS('',3,(#56475,#56476,#56477,#56478,#56479,
#56480,#56481,#56482,#56483,#56484,#56485,#56486,#56487,#56488,#56489,#56490,
#56491,#56492,#56493,#56494,#56495,#56496,#56497,#56498,#56499,#56500,#56501,
#56502,#56503,#56504,#56505,#56506,#56507,#56508,#56509,#56510,#56511,#56512,
#56513,#56514),.UNSPECIFIED.,.F.,.F.,(4,3,3,3,3,3,3,3,3,3,3,3,3,4),(5.14917238118972,
5.36005118608473,5.57092999109581,5.77298643029944,5.97546031432173,6.12802772885396,
6.32462027006809,6.52281590230707,6.6851254666121,6.88364627198843,7.08054113574374,
7.24221135774884,7.44474766119369,7.51426348381143),.UNSPECIFIED.) ;
#445=B_SPLINE_CURVE_WITH_KNOTS('',3,(#56518,#56519,#56520,#56521,#56522,
#56523,#56524,#56525,#56526,#56527,#56528,#56529,#56530,#56531,#56532,#56533,
#56534,#56535,#56536,#56537,#56538,#56539,#56540,#56541,#56542,#56543,#56544,
#56545,#56546,#56547,#56548,#56549,#56550,#56551,#56552,#56553,#56554,#56555,
#56556,#56557),.UNSPECIFIED.,.F.,.F.,(4,3,3,3,3,3,3,3,3,3,3,3,3,4),(1.39920553665764,
1.60174184009116,1.6712576734102,1.86788901812116,2.06612241241911,2.22834356454693,
2.42682695741597,2.62368336398584,2.78544130230508,2.98797174735932,3.19010175291758,
3.34253904006323,3.55341784507458,3.76429664996967),.UNSPECIFIED.) ;
#446=B_SPLINE_CURVE_WITH_KNOTS('',2,(#56559,#56560,#56561),
 .UNSPECIFIED.,.F.,.F.,(3,3),(0.,1.50509385946355),.UNSPECIFIED.) ;
#447=B_SPLINE_CURVE_WITH_KNOTS('',2,(#56565,#56566,#56567),
 .UNSPECIFIED.,.F.,.F.,(3,3),(0.0815875966540559,1.58668145590163),
 .UNSPECIFIED.) ;
#448=B_SPLINE_CURVE_WITH_KNOTS('',3,(#56569,#56570,#56571,#56572,#56573,
#56574,#56575,#56576,#56577,#56578,#56579,#56580,#56581,#56582,#56583,#56584,
#56585,#56586,#56587,#56588,#56589,#56590,#56591,#56592,#56593,#56594,#56595,
#56596,#56597,#56598,#56599,#56600,#56601,#56602,#56603,#56604,#56605,#56606,
#56607,#56608),.UNSPECIFIED.,.F.,.F.,(4,3,3,3,3,3,3,3,3,3,3,3,3,4),(5.14917238118944,
5.36005118608449,5.57092999109581,5.77298643029889,5.97546031432065,6.12802772885396,
6.32462027006934,6.52281590230941,6.68512546661211,6.88364627198978,7.08054113574635,
7.24221135774884,7.4447476611834,7.51426349450135),.UNSPECIFIED.) ;
#449=B_SPLINE_CURVE_WITH_KNOTS('',3,(#56616,#56617,#56618,#56619,#56620,
#56621,#56622,#56623,#56624,#56625,#56626,#56627,#56628,#56629,#56630,#56631,
#56632,#56633,#56634,#56635,#56636,#56637),.UNSPECIFIED.,.F.,.F.,(4,2,2,
2,2,2,2,2,2,2,4),(5.27191149550306E-6,0.0527078513361115,6.45340679863479,
7.10706620105005,7.54824310354326,7.76072560346531,7.78191476646708,7.79349134258084,
7.79962401028583,7.80184798817142,7.80203371562736),.UNSPECIFIED.) ;
#450=B_SPLINE_CURVE_WITH_KNOTS('',3,(#56640,#56641,#56642,#56643,#56644,
#56645,#56646,#56647,#56648,#56649),.UNSPECIFIED.,.F.,.F.,(4,2,2,2,4),(7.80221259693202,
7.80241711061396,7.80965893536248,8.08890869992909,13.8149316250846),
 .UNSPECIFIED.) ;
#451=B_SPLINE_CURVE_WITH_KNOTS('',3,(#56653,#56654,#56655,#56656,#56657,
#56658,#56659,#56660,#56661,#56662,#56663,#56664,#56665,#56666,#56667,#56668,
#56669,#56670,#56671,#56672,#56673,#56674),.UNSPECIFIED.,.F.,.F.,(4,2,2,
2,2,2,2,2,2,2,4),(5.27191148509523E-6,0.0465537949478901,6.44830136700651,
7.10264046407999,7.54412371933544,7.75697956115347,7.7781894765911,7.78977015010294,
7.79592806966615,7.79819769958458,7.79836756459383),.UNSPECIFIED.) ;
#452=B_SPLINE_CURVE_WITH_KNOTS('',3,(#56677,#56678,#56679,#56680,#56681,
#56682,#56683,#56684,#56685,#56686,#56687,#56688),.UNSPECIFIED.,.F.,.F.,
(4,2,2,2,2,4),(7.79863737329538,7.79879895211581,7.811727333517,8.2183177167418,
17.3378811428621,58.4300224110889),.UNSPECIFIED.) ;
#453=B_SPLINE_CURVE_WITH_KNOTS('',3,(#56692,#56693,#56694,#56695,#56696,
#56697,#56698,#56699,#56700,#56701,#56702,#56703,#56704,#56705,#56706,#56707,
#56708,#56709,#56710,#56711,#56712,#56713),.UNSPECIFIED.,.F.,.F.,(4,2,2,
2,2,2,2,2,2,2,4),(5.27191158905907E-6,0.0396446874731099,6.43885097308755,
7.09357142809069,7.53514148843079,7.74829188309382,7.76951301811614,7.78108926141565,
7.78727446991383,7.78888160161461,7.78890865002446),.UNSPECIFIED.) ;
#454=B_SPLINE_CURVE_WITH_KNOTS('',3,(#56716,#56717,#56718,#56719,#56720,
#56721,#56722,#56723,#56724,#56725),.UNSPECIFIED.,.F.,.F.,(4,2,2,2,4),(7.78895653301216,
7.78900494242095,7.79222894606557,7.8726852687626,8.96203806139483),
 .UNSPECIFIED.) ;
#455=B_SPLINE_CURVE_WITH_KNOTS('',3,(#56729,#56730,#56731,#56732,#56733,
#56734,#56735,#56736,#56737,#56738,#56739,#56740,#56741,#56742,#56743,#56744,
#56745,#56746,#56747,#56748,#56749,#56750),.UNSPECIFIED.,.F.,.F.,(4,2,2,
2,2,2,2,2,2,2,4),(5.27191189062319E-6,0.0355022021223558,6.44121530656163,
7.0969892443639,7.53916678802634,7.75276318216616,7.77401784522417,7.78560516000671,
7.79181523099173,7.79344311532259,7.79346999485175),.UNSPECIFIED.) ;
#456=B_SPLINE_CURVE_WITH_KNOTS('',3,(#56753,#56754,#56755,#56756,#56757,
#56758,#56759,#56760,#56761,#56762,#56763,#56764),.UNSPECIFIED.,.F.,.F.,
(4,2,2,2,2,4),(7.79352661259234,7.79358342104345,7.80166819041049,7.90391945213033,
10.5115157415884,22.7185743110134),.UNSPECIFIED.) ;
#457=B_SPLINE_CURVE_WITH_KNOTS('',3,(#56768,#56769,#56770,#56771,#56772,
#56773,#56774,#56775,#56776,#56777,#56778,#56779,#56780,#56781,#56782,#56783,
#56784,#56785,#56786,#56787,#56788,#56789),.UNSPECIFIED.,.F.,.F.,(4,2,2,
2,2,2,2,2,2,2,4),(5.27191147638787E-6,0.0377827332366595,6.43903319305708,
7.0941366968806,7.5359188939874,7.74924020070412,7.77047347261814,7.78205309254291,
7.78824859694197,7.78986477823942,7.78989191787037),.UNSPECIFIED.) ;
#458=B_SPLINE_CURVE_WITH_KNOTS('',3,(#56792,#56793,#56794,#56795,#56796,
#56797,#56798,#56799,#56800,#56801),.UNSPECIFIED.,.F.,.F.,(4,2,2,2,4),(7.78996291674499,
7.7900243542677,7.79393765773531,7.88810518975087,9.08002513845262),
 .UNSPECIFIED.) ;
#459=B_SPLINE_CURVE_WITH_KNOTS('',3,(#56805,#56806,#56807,#56808,#56809,
#56810,#56811,#56812,#56813,#56814,#56815,#56816,#56817,#56818,#56819,#56820,
#56821,#56822,#56823,#56824,#56825,#56826),.UNSPECIFIED.,.F.,.F.,(4,2,2,
2,2,2,2,2,2,2,4),(5.27191138067076E-6,0.0449461593234226,6.44633404502776,
7.1007856663008,7.54230514096117,7.75523728757385,7.77645054559184,7.78803083691326,
7.79419520281166,7.79647958901679,7.79664367287054),.UNSPECIFIED.) ;
#460=B_SPLINE_CURVE_WITH_KNOTS('',3,(#56829,#56830,#56831,#56832,#56833,
#56834,#56835,#56836,#56837,#56838,#56839,#56840,#56841,#56842,#56843,#56844,
#56845,#56846,#56847,#56848,#56849,#56850,#56851,#56852,#56853,#56854,#56855,
#56856),.UNSPECIFIED.,.F.,.F.,(4,3,3,3,3,3,3,3,3,4),(7.79681765090147,7.79693246333981,
7.80264593101425,7.80335304330589,7.86482173740273,8.71154800799036,9.74463365376269,
10.2896549353898,22.5136531132542,24.4500364531805),.UNSPECIFIED.) ;
#461=B_SPLINE_CURVE_WITH_KNOTS('',3,(#56860,#56861,#56862,#56863,#56864,
#56865,#56866,#56867,#56868,#56869,#56870,#56871,#56872,#56873,#56874,#56875,
#56876,#56877,#56878,#56879,#56880,#56881),.UNSPECIFIED.,.F.,.F.,(4,2,2,
2,2,2,2,2,2,2,4),(5.27191147799299E-6,0.0511073819017907,6.45440150746996,
7.10847604594555,7.54989318912631,7.76255058442115,7.78375285138069,7.79533495417965,
7.80147593136055,7.80371064912123,7.80389282491498),.UNSPECIFIED.) ;
#462=B_SPLINE_CURVE_WITH_KNOTS('',3,(#56884,#56885,#56886,#56887,#56888,
#56889,#56890,#56891,#56892,#56893),.UNSPECIFIED.,.F.,.F.,(4,2,2,2,4),(7.80438554879021,
7.80496076768678,7.83948451539625,8.84807105865867,29.8486833513606),
 .UNSPECIFIED.) ;
#463=B_SPLINE_CURVE_WITH_KNOTS('',3,(#56897,#56898,#56899,#56900,#56901,
#56902,#56903,#56904,#56905,#56906,#56907,#56908,#56909,#56910,#56911,#56912,
#56913,#56914,#56915,#56916,#56917,#56918),.UNSPECIFIED.,.F.,.F.,(4,2,2,
2,2,2,2,2,2,2,4),(5.27191166391327E-6,0.0525380308481434,6.45668644422429,
7.11071566703238,7.55213750314294,7.76474488984048,7.78594601623854,7.79752901314693,
7.80366549802474,7.8058915856127,7.80609162294199),.UNSPECIFIED.) ;
#464=B_SPLINE_CURVE_WITH_KNOTS('',3,(#56921,#56922,#56923,#56924,#56925,
#56926,#56927,#56928,#56929,#56930,#56931,#56932),.UNSPECIFIED.,.F.,.F.,
(4,2,2,2,2,4),(7.80644056341581,7.80682262141797,7.85814957526539,8.49497231289726,
25.6284091705695,104.059811221683),.UNSPECIFIED.) ;
#465=B_SPLINE_CURVE_WITH_KNOTS('',3,(#56938,#56939,#56940,#56941,#56942,
#56943,#56944,#56945,#56946,#56947,#56948,#56949,#56950,#56951,#56952,#56953,
#56954,#56955,#56956,#56957,#56958,#56959),.UNSPECIFIED.,.F.,.F.,(4,2,2,
2,2,2,2,2,2,2,4),(5.27191148216978E-6,0.0414743981847573,6.44013831362117,
7.09463297986845,7.53609600585336,7.74912764611573,7.77034174576342,7.78191720208803,
7.78809369888862,7.78969224195007,7.78972443835406),.UNSPECIFIED.) ;
#466=B_SPLINE_CURVE_WITH_KNOTS('',3,(#56962,#56963,#56964,#56965,#56966,
#56967,#56968,#56969,#56970,#56971),.UNSPECIFIED.,.F.,.F.,(4,2,2,2,4),(7.78977667487699,
7.78981377673323,7.79239024212666,7.85784828520671,8.78134693044458),
 .UNSPECIFIED.) ;
#467=B_SPLINE_CURVE_WITH_KNOTS('',3,(#56975,#56976,#56977,#56978,#56979,
#56980,#56981,#56982,#56983,#56984,#56985,#56986,#56987,#56988,#56989,#56990,
#56991,#56992,#56993,#56994,#56995,#56996),.UNSPECIFIED.,.F.,.F.,(4,2,2,
2,2,2,2,2,2,2,4),(5.27191166871522E-6,0.0356514515568032,6.43942015127324,
7.0949804845643,7.53701786178047,7.75054081785537,7.77178857574933,7.78337224535537,
7.78957964075273,7.79120607196549,7.79123706466225),.UNSPECIFIED.) ;
#468=B_SPLINE_CURVE_WITH_KNOTS('',3,(#56999,#57000,#57001,#57002,#57003,
#57004,#57005,#57006,#57007,#57008,#57009,#57010,#57011,#57012,#57013,#57014),
 .UNSPECIFIED.,.F.,.F.,(4,2,2,2,2,2,2,4),(7.79128432176965,7.79131403753904,
7.79508710279556,7.83622558772195,8.30441129116172,8.8671118434176,9.28957449106967,
15.1690241021115),.UNSPECIFIED.) ;
#469=B_SPLINE_CURVE_WITH_KNOTS('',3,(#57018,#57019,#57020,#57021,#57022,
#57023,#57024,#57025,#57026,#57027,#57028,#57029,#57030,#57031,#57032,#57033,
#57034,#57035,#57036,#57037,#57038,#57039),.UNSPECIFIED.,.F.,.F.,(4,2,2,
2,2,2,2,2,2,2,4),(5.27191151498337E-6,0.0359657639257141,6.43915849273793,
7.09463043773541,7.53661602976181,7.7501023827329,7.77134728693642,7.78293006298598,
7.78913549825155,7.79076040490507,7.79078675221503),.UNSPECIFIED.) ;
#470=B_SPLINE_CURVE_WITH_KNOTS('',3,(#57042,#57043,#57044,#57045,#57046,
#57047,#57048,#57049,#57050,#57051,#57052,#57053),.UNSPECIFIED.,.F.,.F.,
(4,2,2,2,2,4),(7.79083814663995,7.79089463150174,7.79821119965064,7.89001115859904,
10.2475238105046,21.2881958971545),.UNSPECIFIED.) ;
#471=B_SPLINE_CURVE_WITH_KNOTS('',3,(#57057,#57058,#57059,#57060,#57061,
#57062,#57063,#57064,#57065,#57066,#57067,#57068,#57069,#57070,#57071,#57072,
#57073,#57074,#57075,#57076,#57077,#57078),.UNSPECIFIED.,.F.,.F.,(4,2,2,
2,2,2,2,2,2,2,4),(5.2719118637948E-6,0.0432725905166975,6.44833055008626,
7.10331460056981,7.54515147355067,7.75829865105336,7.77952893588274,7.79111596175757,
7.79729100354606,7.79959341946853,7.79979287868427),.UNSPECIFIED.) ;
#472=B_SPLINE_CURVE_WITH_KNOTS('',3,(#57081,#57082,#57083,#57084,#57085,
#57086,#57087,#57088,#57089,#57090),.UNSPECIFIED.,.F.,.F.,(4,2,2,2,4),(7.80028431507407,
7.80069015909249,7.83056852627773,8.69977922056581,21.3113858823424),
 .UNSPECIFIED.) ;
#473=B_SPLINE_CURVE_WITH_KNOTS('',3,(#57096,#57097,#57098,#57099,#57100,
#57101,#57102,#57103,#57104,#57105,#57106,#57107,#57108,#57109,#57110,#57111,
#57112,#57113,#57114,#57115,#57116,#57117),.UNSPECIFIED.,.F.,.F.,(4,2,2,
2,2,2,2,2,2,2,4),(5.27191168534313E-6,0.0523927874971037,6.45501410063101,
7.10890009251696,7.55022187180551,7.7627860844029,7.78398255234983,7.79556279674482,
7.80169848168718,7.80392514223319,7.8041092694236),.UNSPECIFIED.) ;
#474=B_SPLINE_CURVE_WITH_KNOTS('',3,(#57120,#57121,#57122,#57123,#57124,
#57125,#57126,#57127,#57128,#57129,#57130,#57131),.UNSPECIFIED.,.F.,.F.,
(4,2,2,2,2,4),(7.80477126540197,7.80558521468643,7.91497253507506,9.27554144510681,
45.7162452587849,212.471335771752),.UNSPECIFIED.) ;
#475=B_SPLINE_CURVE_WITH_KNOTS('',3,(#57135,#57136,#57137,#57138,#57139,
#57140,#57141,#57142,#57143,#57144,#57145,#57146,#57147,#57148,#57149,#57150,
#57151,#57152,#57153,#57154,#57155,#57156,#57157,#57158,#57159,#57160),
 .UNSPECIFIED.,.F.,.F.,(4,2,2,2,2,2,2,2,2,2,2,2,4),(5.27191148861508E-6,
1.47097891395074,5.75978232176541,6.40361086116478,6.48988083888239,7.03787277637638,
7.49650945099211,7.54247660519179,7.67353711320395,7.75556392091874,7.78274835154569,
7.79406144395684,7.80522308440679),.UNSPECIFIED.) ;
#476=B_SPLINE_CURVE_WITH_KNOTS('',3,(#57163,#57164,#57165,#57166,#57167,
#57168,#57169,#57170,#57171,#57172,#57173,#57174,#57175,#57176,#57177,#57178,
#57179,#57180,#57181,#57182),.UNSPECIFIED.,.F.,.F.,(4,2,2,2,2,2,2,2,2,4),
(7.80522308440679,7.80979087307447,8.2018949531721,9.24780316434757,9.79842768307673,
10.2918952776785,43.49970799473,58.02812605844,60.3284654325973,275.954206920472),
 .UNSPECIFIED.) ;
#477=B_SPLINE_CURVE_WITH_KNOTS('',3,(#57186,#57187,#57188,#57189,#57190,
#57191,#57192,#57193,#57194,#57195,#57196,#57197,#57198,#57199,#57200,#57201,
#57202,#57203,#57204,#57205,#57206,#57207),.UNSPECIFIED.,.F.,.F.,(4,2,2,
2,2,2,2,2,2,2,4),(5.27191187477842E-6,0.0432725252097352,6.44831604470414,
7.1032986187713,7.54513449628265,7.75828119283847,7.77951138720516,7.79109852155536,
7.79727326708117,7.79957524268641,7.79974556459194),.UNSPECIFIED.) ;
#478=B_SPLINE_CURVE_WITH_KNOTS('',3,(#57210,#57211,#57212,#57213,#57214,
#57215,#57216,#57217,#57218,#57219),.UNSPECIFIED.,.F.,.F.,(4,2,2,2,4),(7.79995524677398,
7.80010024939709,7.81075911559854,8.12013970698806,12.6093269820519),
 .UNSPECIFIED.) ;
#479=B_SPLINE_CURVE_WITH_KNOTS('',3,(#57223,#57224,#57225,#57226,#57227,
#57228,#57229,#57230,#57231,#57232,#57233,#57234,#57235,#57236,#57237,#57238,
#57239,#57240,#57241,#57242,#57243,#57244),.UNSPECIFIED.,.F.,.F.,(4,2,2,
2,2,2,2,2,2,2,4),(5.271912279136E-6,0.0359879560292855,6.44510187443905,
7.10117994822179,7.54357425347277,7.75725802200454,7.77852259826938,7.79011608262715,
7.7963274350803,7.79795412309629,7.79798119670788),.UNSPECIFIED.) ;
#480=B_SPLINE_CURVE_WITH_KNOTS('',3,(#57247,#57248,#57249,#57250,#57251,
#57252,#57253,#57254,#57255,#57256,#57257,#57258),.UNSPECIFIED.,.F.,.F.,
(4,2,2,2,2,4),(7.79803620397162,7.79809114082297,7.80515926793939,7.89384206027351,
10.1712995690942,20.8370576609684),.UNSPECIFIED.) ;
#481=B_SPLINE_CURVE_WITH_KNOTS('',3,(#57262,#57263,#57264,#57265,#57266,
#57267,#57268,#57269,#57270,#57271,#57272,#57273,#57274,#57275,#57276,#57277,
#57278,#57279,#57280,#57281,#57282,#57283),.UNSPECIFIED.,.F.,.F.,(4,2,2,
2,2,2,2,2,2,2,4),(5.27191168080902E-6,0.0356505571059927,6.43917854529716,
7.0947142369843,7.5367349984191,7.75024992867144,7.77149687789579,7.78308023607464,
7.78928745150985,7.79091398242415,7.79094393251091),.UNSPECIFIED.) ;
#482=B_SPLINE_CURVE_WITH_KNOTS('',3,(#57286,#57287,#57288,#57289,#57290,
#57291,#57292,#57293,#57294,#57295,#57296,#57297),.UNSPECIFIED.,.F.,.F.,
(4,2,2,2,2,4),(7.79100926174046,7.79108071178542,7.80013022621495,7.91427990087799,
10.8320810124655,24.4930959714559),.UNSPECIFIED.) ;
#483=B_SPLINE_CURVE_WITH_KNOTS('',3,(#57301,#57302,#57303,#57304,#57305,
#57306,#57307,#57308,#57309,#57310,#57311,#57312,#57313,#57314,#57315,#57316,
#57317,#57318,#57319,#57320,#57321,#57322),.UNSPECIFIED.,.F.,.F.,(4,2,2,
2,2,2,2,2,2,2,4),(5.27191187344555E-6,0.0415033517824493,6.44685814573985,
7.10203719509694,7.54395170849138,7.75721624445404,7.77845257041729,7.79004012437634,
7.79622326565104,7.79782372936473,7.79785623932904),.UNSPECIFIED.) ;
#484=B_SPLINE_CURVE_WITH_KNOTS('',3,(#57325,#57326,#57327,#57328,#57329,
#57330,#57331,#57332,#57333,#57334,#57335,#57336,#57337,#57338,#57339,#57340,
#57341,#57342),.UNSPECIFIED.,.F.,.F.,(4,2,2,2,2,2,2,2,4),(7.79793150207117,
7.79814723346125,7.79870043059623,7.80649383530305,7.89256327609095,7.99478803002891,
8.06034762858735,9.28573631573981,9.36839839072109),.UNSPECIFIED.) ;
#485=B_SPLINE_CURVE_WITH_KNOTS('',3,(#57346,#57347,#57348,#57349,#57350,
#57351,#57352,#57353,#57354,#57355,#57356,#57357,#57358,#57359,#57360,#57361,
#57362,#57363,#57364,#57365,#57366,#57367,#57368,#57369,#57370,#57371,#57372,
#57373),.UNSPECIFIED.,.F.,.F.,(4,2,2,2,1,2,2,2,2,2,2,2,2,1,4),(5.27191159103619E-6,
1.04820808125431,4.7657172239378,5.66605146943146,6.11270166153183,6.41832688046243,
6.4954431947857,7.09297306404379,7.38226395613211,7.6384860640954,7.75703692454204,
7.78060543766242,7.79405002558409,7.79920996916132,7.80436991273856),
 .UNSPECIFIED.) ;
#486=B_SPLINE_CURVE_WITH_KNOTS('',3,(#57376,#57377,#57378,#57379,#57380,
#57381,#57382,#57383,#57384,#57385,#57386,#57387,#57388,#57389,#57390,#57391,
#57392,#57393),.UNSPECIFIED.,.F.,.F.,(4,2,2,2,2,2,2,2,4),(7.80436991273856,
7.80474232030115,7.88242710709233,8.75841205662384,8.96393995438549,22.8445100409781,
28.9172594538623,29.9482351239262,120.00842073875),.UNSPECIFIED.) ;
#487=B_SPLINE_CURVE_WITH_KNOTS('',3,(#57397,#57398,#57399,#57400,#57401,
#57402,#57403,#57404,#57405,#57406,#57407,#57408,#57409,#57410,#57411,#57412,
#57413,#57414,#57415,#57416,#57417,#57418),.UNSPECIFIED.,.F.,.F.,(4,2,2,
2,2,2,2,2,2,2,4),(5.2719118122293E-6,0.0525432957185552,6.45765275965806,
7.11178013090022,7.55326821002014,7.76590750214238,7.78711180679313,7.79869646853999,
7.80483393332087,7.80706039962179,7.80724567724711),.UNSPECIFIED.) ;
#488=B_SPLINE_CURVE_WITH_KNOTS('',3,(#57421,#57422,#57423,#57424,#57425,
#57426,#57427,#57428,#57429,#57430,#57431,#57432),.UNSPECIFIED.,.F.,.F.,
(4,2,2,2,2,4),(7.80754124133301,7.80785818194975,7.8504276541488,8.37868320530173,
22.5834113324897,87.6053326518759),.UNSPECIFIED.) ;
#489=B_SPLINE_CURVE_WITH_KNOTS('',3,(#57436,#57437,#57438,#57439,#57440,
#57441,#57442,#57443,#57444,#57445,#57446,#57447,#57448,#57449,#57450,#57451,
#57452,#57453,#57454,#57455,#57456,#57457),.UNSPECIFIED.,.F.,.F.,(4,2,2,
2,2,2,2,2,2,2,4),(5.27191176710306E-6,0.0511111946987736,6.45512057751185,
7.10926817712045,7.55073462661806,7.76341577672905,7.78462040594282,7.79620374455683,
7.80234564099213,7.80458100357878,7.80476406937864),.UNSPECIFIED.) ;
#490=B_SPLINE_CURVE_WITH_KNOTS('',3,(#57460,#57461,#57462,#57463,#57464,
#57465,#57466,#57467,#57468,#57469),.UNSPECIFIED.,.F.,.F.,(4,2,2,2,4),(7.80523453137563,
7.80581761661808,7.84080868875818,8.86305145409338,30.1478164970341),
 .UNSPECIFIED.) ;
#491=B_SPLINE_CURVE_WITH_KNOTS('',3,(#57473,#57474,#57475,#57476,#57477,
#57478,#57479,#57480,#57481,#57482,#57483,#57484,#57485,#57486,#57487,#57488,
#57489,#57490,#57491,#57492,#57493,#57494),.UNSPECIFIED.,.F.,.F.,(4,2,2,
2,2,2,2,2,2,2,4),(5.27191169017701E-6,0.0449566642310049,6.44858512306242,
7.10326581171296,7.54493982518336,7.7579465003635,7.77916725766819,7.7907515857637,
7.79691817502006,7.79920352721897,7.7993673461476),.UNSPECIFIED.) ;
#492=B_SPLINE_CURVE_WITH_KNOTS('',3,(#57497,#57498,#57499,#57500,#57501,
#57502,#57503,#57504,#57505,#57506,#57507,#57508),.UNSPECIFIED.,.F.,.F.,
(4,2,2,2,2,4),(7.79964068154672,7.79984266942381,7.81523993495469,8.180553028938,
16.1414183538315,51.9114717465994),.UNSPECIFIED.) ;
#493=B_SPLINE_CURVE_WITH_KNOTS('',3,(#57512,#57513,#57514,#57515,#57516,
#57517,#57518,#57519,#57520,#57521,#57522,#57523,#57524,#57525,#57526,#57527,
#57528,#57529,#57530,#57531,#57532,#57533),.UNSPECIFIED.,.F.,.F.,(4,2,2,
2,2,2,2,2,2,2,4),(5.27191157823416E-6,0.0377812881750992,6.43866511053677,
7.09373109278456,7.53548798669349,7.74879707503235,7.77002911215379,7.78160814123601,
7.78780327656431,7.78941938430865,7.78944792551213),.UNSPECIFIED.) ;
#494=B_SPLINE_CURVE_WITH_KNOTS('',3,(#57536,#57537,#57538,#57539,#57540,
#57541,#57542,#57543,#57544,#57545),.UNSPECIFIED.,.F.,.F.,(4,2,2,2,4),(7.78950417221257,
7.78954999296874,7.79247137180975,7.86278869254345,8.75285890777793),
 .UNSPECIFIED.) ;
#495=B_SPLINE_CURVE_WITH_KNOTS('',3,(#57549,#57550,#57551,#57552,#57553,
#57554,#57555,#57556,#57557,#57558,#57559,#57560,#57561,#57562,#57563,#57564,
#57565,#57566,#57567,#57568,#57569,#57570),.UNSPECIFIED.,.F.,.F.,(4,2,2,
2,2,2,2,2,2,2,4),(5.27191169046416E-6,0.0354948744565003,6.43922713707928,
7.09479828954679,7.53683909853423,7.7503694420143,7.77161751967803,7.78320124737355,
7.78940924098477,7.79103637023299,7.7910624807489),.UNSPECIFIED.) ;
#496=B_SPLINE_CURVE_WITH_KNOTS('',3,(#57573,#57574,#57575,#57576,#57577,
#57578,#57579,#57580,#57581,#57582,#57583,#57584),.UNSPECIFIED.,.F.,.F.,
(4,2,2,2,2,4),(7.79111289413845,7.79116616933223,7.79788554663789,7.88286765791431,
10.0499826184928,20.1949747619141),.UNSPECIFIED.) ;
#497=B_SPLINE_CURVE_WITH_KNOTS('',3,(#57588,#57589,#57590,#57591,#57592,
#57593,#57594,#57595,#57596,#57597,#57598,#57599,#57600,#57601,#57602,#57603,
#57604,#57605,#57606,#57607,#57608,#57609),.UNSPECIFIED.,.F.,.F.,(4,2,2,
2,2,2,2,2,2,2,4),(5.27191168177523E-6,0.0396625350310654,6.443183559499,
7.09834546596198,7.54021325882577,7.75350737242496,7.77474277060722,7.78632676826843,
7.79251614782254,7.7941243263727,7.79415422696317),.UNSPECIFIED.) ;
#498=B_SPLINE_CURVE_WITH_KNOTS('',3,(#57612,#57613,#57614,#57615,#57616,
#57617,#57618,#57619,#57620,#57621),.UNSPECIFIED.,.F.,.F.,(4,2,2,2,4),(7.794199587327,
7.7942340932038,7.79653236739817,7.85378276088928,8.62896774962984),
 .UNSPECIFIED.) ;
#499=B_SPLINE_CURVE_WITH_KNOTS('',3,(#57625,#57626,#57627,#57628,#57629,
#57630,#57631,#57632,#57633,#57634,#57635,#57636,#57637,#57638,#57639,#57640,
#57641,#57642,#57643,#57644,#57645,#57646),.UNSPECIFIED.,.F.,.F.,(4,2,2,
2,2,2,2,2,2,2,4),(5.2719115819804E-6,0.0465604352314907,6.44967554861822,
7.10415442622451,7.54573199163219,7.75863330383081,7.7798478022043,7.79143103500224,
7.79759014313736,7.79986010495208,7.80003908106863),.UNSPECIFIED.) ;
#500=B_SPLINE_CURVE_WITH_KNOTS('',3,(#57649,#57650,#57651,#57652,#57653,
#57654,#57655,#57656,#57657,#57658,#57659,#57660),.UNSPECIFIED.,.F.,.F.,
(4,2,2,2,2,4),(7.80029559813691,7.80047746006334,7.81505666974208,8.27340780924998,
18.5539386231002,64.8773239617285),.UNSPECIFIED.) ;
#501=B_SPLINE_CURVE_WITH_KNOTS('',3,(#57664,#57665,#57666,#57667,#57668,
#57669,#57670,#57671,#57672,#57673,#57674,#57675,#57676,#57677,#57678,#57679,
#57680,#57681,#57682,#57683,#57684,#57685),.UNSPECIFIED.,.F.,.F.,(4,2,2,
2,2,2,2,2,2,2,4),(5.27191148200324E-6,0.0527129873805481,6.45434578160439,
7.10810055256914,7.54934182256476,7.76185532353388,7.78304756105929,7.79462588360834,
7.8007593731596,7.8029837332684,7.80317840349864),.UNSPECIFIED.) ;
#502=B_SPLINE_CURVE_WITH_KNOTS('',3,(#57688,#57689,#57690,#57691,#57692,
#57693,#57694,#57695,#57696,#57697,#57698,#57699),.UNSPECIFIED.,.F.,.F.,
(4,2,2,2,2,4),(7.80373274627093,7.80444564896149,7.9001288190428,9.08312630466139,
41.1183452310278,187.839302386062),.UNSPECIFIED.) ;
#503=B_SPLINE_CURVE_WITH_KNOTS('',3,(#57702,#57703,#57704,#57705,#57706,
#57707,#57708,#57709,#57710,#57711,#57712,#57713,#57714,#57715,#57716,#57717,
#57718,#57719,#57720,#57721,#57722,#57723,#57724,#57725,#57726,#57727),
 .UNSPECIFIED.,.F.,.F.,(4,2,2,2,2,2,2,2,2,2,2,2,4),(5.27191147116053E-6,
1.14584468705305,5.27595614080581,6.27621750851155,6.42842423170021,6.49296697752034,
7.05675108509317,7.48372044806425,7.72947375032807,7.77323441341815,7.79046163520876,
7.79956239767949,7.80160940374884),.UNSPECIFIED.) ;
#504=B_SPLINE_CURVE_WITH_KNOTS('',3,(#57730,#57731,#57732,#57733,#57734,
#57735,#57736,#57737,#57738,#57739,#57740,#57741,#57742,#57743,#57744,#57745,
#57746,#57747,#57748,#57749),.UNSPECIFIED.,.F.,.F.,(4,2,2,2,2,2,2,2,2,4),
(7.80160940758295,7.8089379799619,7.99849136645798,8.48798714708565,8.85467142169077,
9.05313731358241,24.5851715502772,31.3804365288312,32.5696272011659,133.309321825113),
 .UNSPECIFIED.) ;
#505=B_SPLINE_CURVE_WITH_KNOTS('',3,(#57751,#57752,#57753,#57754,#57755,
#57756,#57757,#57758,#57759,#57760,#57761,#57762,#57763,#57764,#57765,#57766,
#57767,#57768,#57769,#57770,#57771,#57772,#57773,#57774,#57775,#57776,#57777,
#57778),.UNSPECIFIED.,.F.,.F.,(4,2,2,2,2,2,2,2,2,2,2,2,2,4),(5.27191147341303E-6,
1.28771119835054,3.98796378162772,5.31699434995946,5.97631810846778,6.42862113427837,
6.4934258850079,7.14815420783244,7.47423960298919,7.64928235471921,7.73777852432768,
7.78772679076623,7.79646451937251,7.80216111214384),.UNSPECIFIED.) ;
#506=B_SPLINE_CURVE_WITH_KNOTS('',3,(#57781,#57782,#57783,#57784,#57785,
#57786,#57787,#57788,#57789,#57790,#57791,#57792,#57793,#57794,#57795,#57796,
#57797,#57798,#57799,#57800),.UNSPECIFIED.,.F.,.F.,(4,2,2,2,2,2,2,2,2,4),
(7.80216111214384,7.81235512109906,8.05788043165933,8.70649760391101,9.05150172288028,
9.31799764820168,29.9162325081877,38.9279602594316,40.3746267938085,174.103758636969),
 .UNSPECIFIED.) ;
#507=B_SPLINE_CURVE_WITH_KNOTS('',3,(#57987,#57988,#57989,#57990,#57991,
#57992,#57993,#57994,#57995,#57996,#57997,#57998,#57999,#58000,#58001,#58002,
#58003,#58004,#58005,#58006,#58007,#58008,#58009,#58010,#58011,#58012,#58013,
#58014,#58015,#58016,#58017,#58018,#58019,#58020,#58021,#58022,#58023,#58024,
#58025,#58026,#58027,#58028,#58029,#58030,#58031,#58032,#58033,#58034,#58035,
#58036,#58037,#58038,#58039,#58040,#58041,#58042,#58043,#58044,#58045,#58046,
#58047,#58048,#58049,#58050,#58051,#58052,#58053,#58054,#58055,#58056,#58057,
#58058,#58059,#58060,#58061,#58062,#58063,#58064,#58065,#58066,#58067,#58068,
#58069,#58070,#58071,#58072,#58073,#58074,#58075,#58076),.UNSPECIFIED.,
 .F.,.F.,(4,2,2,2,2,2,2,2,2,2,2,2,2,2,2,2,2,2,2,2,2,2,2,2,2,2,2,2,2,2,2,
2,2,2,2,2,2,2,2,2,2,2,2,2,4),(1.42697216485095,1.642313125249,3.28462625049799,
4.92693937574699,6.56925250099599,7.39040906362048,8.21156562624498,9.03272218886948,
9.85387875149398,10.2644570328062,10.6750353141185,11.0856135954307,11.496191876743,
11.9067701580552,12.3173484393675,12.5226375800236,12.7279267206797,12.9332158613358,
13.138505001992,13.3261120329266,13.4199155483939,13.5137190638612,13.6075225793285,
13.6544243370621,13.7013260947958,13.7482278525294,13.7951296102631,13.8185804891299,
13.8420313679967,13.8654822468635,13.877207686297,13.8889331257304,13.9006742956463,
13.9124154655623,13.9182860505203,13.9241566354783,13.9270919279573,13.9300272204363,
13.9329625129153,13.9344301591548,13.9358978053943,13.9366528001863,13.9374077949783,
13.9381627897703,13.9385402871663),.UNSPECIFIED.) ;
#508=B_SPLINE_CURVE_WITH_KNOTS('',3,(#58079,#58080,#58081,#58082,#58083,
#58084,#58085,#58086,#58087,#58088,#58089,#58090,#58091,#58092,#58093,#58094,
#58095,#58096,#58097,#58098,#58099,#58100,#58101,#58102,#58103,#58104,#58105,
#58106,#58107,#58108,#58109,#58110,#58111,#58112,#58113,#58114,#58115,#58116,
#58117,#58118,#58119,#58120,#58121,#58122,#58123,#58124,#58125,#58126,#58127,
#58128,#58129,#58130,#58131,#58132,#58133,#58134,#58135,#58136,#58137,#58138,
#58139,#58140,#58141,#58142,#58143,#58144,#58145,#58146,#58147,#58148,#58149,
#58150,#58151,#58152,#58153,#58154,#58155,#58156,#58157,#58158,#58159,#58160,
#58161,#58162,#58163,#58164,#58165,#58166,#58167,#58168),.UNSPECIFIED.,
 .F.,.F.,(4,2,2,2,2,2,2,2,2,2,2,2,2,2,2,2,2,2,2,2,2,2,2,2,2,2,2,2,2,2,2,
2,2,2,2,2,2,2,2,2,2,2,2,2,4),(13.9397809911914,13.9401584882633,13.9409134824073,
13.9416684765512,13.9424234706951,13.9438911167666,13.9453587628381,13.9482940549812,
13.9512293471242,13.9541646392672,13.9600352235533,13.9659058078393,13.9776469764114,
13.9893881449835,14.0011135844584,14.0128390239333,14.0362899028832,14.059740781833,
14.0831916607828,14.1300934186824,14.176995176582,14.2238969344817,14.2707986923813,
14.3646022081806,14.4584057239798,14.5522092397791,14.7398162713776,14.9451054120337,
15.1503945526898,15.355683693346,15.5609728340021,15.9715511153143,16.3821293966266,
16.7927076779388,17.2032859592511,17.6138642405633,18.0244425218756,18.8455990845001,
19.6667556471246,20.4879122097491,21.3090687723736,22.9513818976226,24.5936950228716,
26.2360081481206,26.4513491085187),.UNSPECIFIED.) ;
#509=B_SPLINE_CURVE_WITH_KNOTS('',3,(#58173,#58174,#58175,#58176,#58177,
#58178,#58179,#58180,#58181,#58182,#58183,#58184,#58185,#58186,#58187,#58188,
#58189,#58190,#58191,#58192,#58193,#58194,#58195,#58196,#58197,#58198,#58199,
#58200,#58201,#58202,#58203,#58204,#58205,#58206,#58207,#58208,#58209,#58210,
#58211,#58212,#58213,#58214,#58215,#58216,#58217,#58218,#58219,#58220,#58221,
#58222,#58223,#58224,#58225,#58226,#58227,#58228,#58229,#58230,#58231,#58232,
#58233,#58234,#58235,#58236,#58237,#58238,#58239,#58240,#58241,#58242,#58243,
#58244,#58245,#58246,#58247,#58248,#58249,#58250,#58251,#58252,#58253,#58254,
#58255,#58256,#58257,#58258,#58259,#58260),.UNSPECIFIED.,.F.,.F.,(4,2,2,
2,2,2,2,2,2,2,2,2,2,2,2,2,2,2,2,2,2,2,2,2,2,2,2,2,2,2,2,2,2,2,2,2,2,2,2,
2,2,2,2,4),(14.1204637881216,14.1208456566844,14.1216093938099,14.1223731309355,
14.123136868061,14.1246217770385,14.1261066860159,14.1290765039707,14.1320463219256,
14.1350161398804,14.1409557757901,14.1468954116998,14.1587746835192,14.1706539553386,
14.182518573564,14.1943831917895,14.2181124282403,14.2418416646912,14.2655709011421,
14.3130293740439,14.3604878469457,14.4079463198475,14.4554047927492,14.5503217385528,
14.6452386843564,14.7401556301599,14.929989521767,15.1379533273813,15.3459171329956,
15.5538809386098,15.7618447442241,16.1777723554526,16.5936999666812,17.0096275779097,
17.4255551891382,17.8414828003668,18.2574104115953,19.0892656340524,19.9211208565095,
20.7529760789665,21.5848313014236,23.2485417463377,24.9122521912519,26.627144761),
 .UNSPECIFIED.) ;
#510=B_SPLINE_CURVE_WITH_KNOTS('',3,(#58261,#58262,#58263,#58264,#58265,
#58266,#58267,#58268,#58269,#58270,#58271,#58272,#58273,#58274,#58275,#58276,
#58277,#58278,#58279,#58280,#58281,#58282,#58283,#58284,#58285,#58286,#58287,
#58288,#58289,#58290,#58291,#58292,#58293,#58294,#58295,#58296,#58297,#58298,
#58299,#58300,#58301,#58302,#58303,#58304,#58305,#58306,#58307,#58308,#58309,
#58310,#58311,#58312,#58313,#58314,#58315,#58316,#58317,#58318,#58319,#58320,
#58321,#58322,#58323,#58324,#58325,#58326,#58327,#58328,#58329,#58330,#58331,
#58332,#58333,#58334,#58335,#58336,#58337,#58338,#58339,#58340,#58341,#58342,
#58343,#58344,#58345,#58346,#58347,#58348,#58349,#58350),.UNSPECIFIED.,
 .F.,.F.,(4,2,2,2,2,2,2,2,2,2,2,2,2,2,2,2,2,2,2,2,2,2,2,2,2,2,2,2,2,2,2,
2,2,2,2,2,2,2,2,2,2,2,2,2,4),(1.61252832007444,1.66371044461233,3.32742088922465,
4.99113133383698,6.6548417784493,7.48669700075546,8.31855222306163,9.15040744536779,
9.98226266767395,10.398190278827,10.8141178899801,11.2300455011332,11.6459731122863,
12.0619007234394,12.4778283345924,12.685792140169,12.8937559457455,13.1017197513221,
13.3096835568986,13.4995174488634,13.5944343948458,13.6893513408282,13.7842682868105,
13.8317267598017,13.8791852327929,13.9266437057841,13.9741021787753,13.9978314152709,
14.0215606517665,14.0452898882621,14.0571545065099,14.0690191247577,14.0808983967437,
14.0927776687297,14.0987173047227,14.1046569407157,14.1076267587122,14.1105965767087,
14.1135663947052,14.1150513037034,14.1165362127017,14.1172999492339,14.1180636857662,
14.1188274222985,14.1192092905646),.UNSPECIFIED.) ;
#511=B_SPLINE_CURVE_WITH_KNOTS('',3,(#58355,#58356,#58357,#58358,#58359,
#58360,#58361,#58362,#58363,#58364,#58365,#58366,#58367,#58368,#58369,#58370,
#58371,#58372,#58373,#58374,#58375,#58376,#58377,#58378,#58379,#58380,#58381,
#58382,#58383,#58384,#58385,#58386,#58387,#58388,#58389,#58390,#58391,#58392,
#58393,#58394,#58395,#58396,#58397,#58398,#58399,#58400,#58401,#58402,#58403,
#58404,#58405,#58406,#58407,#58408,#58409,#58410,#58411,#58412,#58413,#58414,
#58415,#58416,#58417,#58418,#58419,#58420,#58421,#58422,#58423,#58424,#58425,
#58426,#58427,#58428,#58429,#58430,#58431,#58432,#58433,#58434,#58435,#58436,
#58437,#58438,#58439,#58440,#58441,#58442),.UNSPECIFIED.,.F.,.F.,(4,2,2,
2,2,2,2,2,2,2,2,2,2,2,2,2,2,2,2,2,2,2,2,2,2,2,2,2,2,2,2,2,2,2,2,2,2,2,2,
2,2,2,2,4),(14.1663480266505,14.1667310032561,14.1674969564673,14.1682629096785,
14.1690288628896,14.1705181494738,14.1720074360579,14.1749860092261,14.1779645823943,
14.1809431555625,14.1869003018989,14.1928574482354,14.2047717409082,14.2166860335811,
14.2285859486937,14.2404858638063,14.2642856940314,14.2880855242566,14.3118853544817,
14.359485014932,14.4070846753823,14.4546843358327,14.502283996283,14.5974833171836,
14.6926826380842,14.7878819589848,14.9782806007861,15.1869236860124,15.3955667712387,
15.604209856465,15.8128529416912,16.2301391121438,16.6474252825964,17.064711453049,
17.4819976235016,17.8992837939541,18.3165699644067,19.1511423053119,19.985714646217,
20.8202869871222,21.6548593280273,23.3240040098377,24.993148691648,26.671883998059),
 .UNSPECIFIED.) ;
#512=B_SPLINE_CURVE_WITH_KNOTS('',3,(#58443,#58444,#58445,#58446,#58447,
#58448,#58449,#58450,#58451,#58452,#58453,#58454,#58455,#58456,#58457,#58458,
#58459,#58460,#58461,#58462,#58463,#58464,#58465,#58466,#58467,#58468,#58469,
#58470,#58471,#58472,#58473,#58474,#58475,#58476,#58477,#58478,#58479,#58480,
#58481,#58482,#58483,#58484,#58485,#58486,#58487,#58488,#58489,#58490,#58491,
#58492,#58493,#58494,#58495,#58496,#58497,#58498,#58499,#58500,#58501,#58502,
#58503,#58504,#58505,#58506,#58507,#58508,#58509,#58510,#58511,#58512,#58513,
#58514,#58515,#58516,#58517,#58518,#58519,#58520,#58521,#58522,#58523,#58524,
#58525,#58526,#58527,#58528,#58529,#58530,#58531,#58532),.UNSPECIFIED.,
 .F.,.F.,(4,2,2,2,2,2,2,2,2,2,2,2,2,2,2,2,2,2,2,2,2,2,2,2,2,2,2,2,2,2,2,
2,2,2,2,2,2,2,2,2,2,2,2,2,4),(1.65955405720668,1.66914468166147,3.33828936332295,
5.00743404498442,6.6765787266459,7.51115106747663,8.34572340830737,9.18029574913811,
10.0148680899688,10.4321542603842,10.8494404307996,11.266726601215,11.6840127716303,
12.1012989420457,12.5185851124611,12.7272281976687,12.9358712828764,13.1445143680841,
13.3531574532918,13.5435560957881,13.6387554170363,13.7339547382844,13.8291540595326,
13.8767537201567,13.9243533807807,13.9719530414048,14.0195527020289,14.0433525323409,
14.067152362653,14.090952192965,14.102852108121,14.1147520232771,14.1266663151852,
14.1385806070933,14.1445377530473,14.1504948990014,14.1534734719784,14.1564520449554,
14.1594306179325,14.160919904421,14.1624091909095,14.1631751442385,14.1639410975676,
14.1647070508966,14.1650900275612),.UNSPECIFIED.) ;
#513=B_SPLINE_CURVE_WITH_KNOTS('',3,(#58537,#58538,#58539,#58540,#58541,
#58542,#58543,#58544,#58545,#58546,#58547,#58548,#58549,#58550,#58551,#58552,
#58553,#58554,#58555,#58556,#58557,#58558,#58559,#58560,#58561,#58562,#58563,
#58564,#58565,#58566,#58567,#58568,#58569,#58570,#58571,#58572,#58573,#58574,
#58575,#58576,#58577,#58578,#58579,#58580,#58581,#58582,#58583,#58584,#58585,
#58586,#58587,#58588,#58589,#58590,#58591,#58592,#58593,#58594,#58595,#58596,
#58597,#58598,#58599,#58600,#58601,#58602,#58603,#58604,#58605,#58606,#58607,
#58608,#58609,#58610,#58611,#58612,#58613,#58614,#58615,#58616,#58617,#58618,
#58619,#58620,#58621,#58622,#58623,#58624,#58625),.UNSPECIFIED.,.F.,.F.,
(4,2,2,2,2,2,2,2,2,2,2,2,2,2,2,2,2,2,2,2,2,2,2,2,2,2,2,2,2,2,2,2,2,2,2,
2,2,2,2,2,2,2,2,1,4),(14.0669078671381,14.0672884413977,14.0680495899169,
14.0688107384361,14.0695718869553,14.0710516830252,14.0725314790952,14.075491071235,
14.0784506633748,14.0814102555147,14.0873294397944,14.093248624074,14.1050869926334,
14.1169253611927,14.1287487567706,14.1405721523484,14.164218943504,14.1878657346596,
14.2115125258153,14.2588061081265,14.3060996904378,14.3533932727491,14.4006868550603,
14.4952740196829,14.5898611843054,14.684448348928,14.873622678173,15.0807936569189,
15.2879646356648,15.4951356144107,15.7023065931566,16.1166485506484,16.5309905081402,
16.945332465632,17.3596744231238,17.7740163806156,18.1883583381074,19.0170422530911,
19.8457261680747,20.6744100830583,21.5030939980419,23.1604618280091,24.8178296579763,
26.4751974879435,26.5749735502974),.UNSPECIFIED.) ;
#514=B_SPLINE_CURVE_WITH_KNOTS('',3,(#58626,#58627,#58628,#58629,#58630,
#58631,#58632,#58633,#58634,#58635,#58636,#58637,#58638,#58639,#58640,#58641,
#58642,#58643,#58644,#58645,#58646,#58647,#58648,#58649,#58650,#58651,#58652,
#58653,#58654,#58655,#58656,#58657,#58658,#58659,#58660,#58661,#58662,#58663,
#58664,#58665,#58666,#58667,#58668,#58669,#58670,#58671,#58672,#58673,#58674,
#58675,#58676,#58677,#58678,#58679,#58680,#58681,#58682,#58683,#58684,#58685,
#58686,#58687,#58688,#58689,#58690,#58691,#58692,#58693,#58694,#58695,#58696,
#58697,#58698,#58699,#58700,#58701,#58702,#58703,#58704,#58705,#58706,#58707,
#58708,#58709,#58710,#58711,#58712,#58713,#58714,#58715),.UNSPECIFIED.,
 .F.,.F.,(4,2,2,2,2,2,2,2,2,2,2,2,2,2,2,2,2,2,2,2,2,2,2,2,2,2,2,2,2,2,2,
2,2,2,2,2,2,2,2,2,2,2,2,2,4),(1.55759176761474,1.65736783004784,3.31473566009569,
4.97210349014353,6.62947132019138,7.4581552352153,8.28683915023922,9.11552306526314,
9.94420698028706,10.358548937799,10.772890895311,11.1872328528229,11.6015748103349,
12.0159167678469,12.4302587253588,12.6374297041148,12.8446006828708,13.0517716616268,
13.2589426403828,13.4481169692896,13.542704133743,13.6372912981964,13.7318784626498,
13.7791720448765,13.8264656271032,13.8737592093299,13.9210527915566,13.94469958267,
13.9683463737833,13.9919931648967,14.0038165604533,14.01563995601,14.0274783250456,
14.0393166940813,14.0452358785991,14.0511550631169,14.0541146553758,14.0570742476347,
14.0600338398936,14.0615136360231,14.0629934321526,14.0637545805585,14.0645157289644,
14.0652768773704,14.0656574515733),.UNSPECIFIED.) ;
#515=B_SPLINE_CURVE_WITH_KNOTS('',3,(#58720,#58721,#58722,#58723,#58724,
#58725,#58726,#58727,#58728,#58729,#58730,#58731,#58732,#58733,#58734,#58735,
#58736,#58737,#58738,#58739,#58740,#58741,#58742,#58743,#58744,#58745,#58746,
#58747,#58748,#58749,#58750,#58751,#58752,#58753,#58754,#58755,#58756,#58757,
#58758,#58759,#58760,#58761,#58762,#58763,#58764,#58765,#58766,#58767,#58768,
#58769,#58770,#58771,#58772,#58773,#58774,#58775,#58776,#58777,#58778,#58779,
#58780,#58781,#58782,#58783,#58784,#58785,#58786,#58787,#58788,#58789,#58790,
#58791,#58792,#58793,#58794,#58795,#58796,#58797,#58798,#58799,#58800,#58801,
#58802,#58803,#58804,#58805,#58806,#58807,#58808,#58809),.UNSPECIFIED.,
 .F.,.F.,(4,2,2,2,2,2,2,2,2,2,2,2,2,2,2,2,2,2,2,2,2,2,2,2,2,2,2,2,2,2,2,
2,2,2,2,2,2,2,2,2,2,2,2,2,4),(14.021342562188,14.021722034217,14.022480978275,
14.023239922333,14.023998866391,14.0254743099342,14.0269497534774,14.0299006405638,
14.0328515276501,14.0358024147365,14.0417041889092,14.0476059630819,14.0594095114273,
14.0712130597728,14.0830013624884,14.0947896652041,14.1183662706354,14.1419428760667,
14.165519481498,14.2126726923606,14.2598259032232,14.3069791140858,14.3541323249484,
14.4484387466737,14.5427451683989,14.6370515901241,14.8256644335745,15.032160898502,
15.2386573634295,15.445153828357,15.6516502932844,16.0646432231394,16.4776361529944,
16.8906290828493,17.3036220127043,17.7166149425593,18.1296078724142,18.9555937321241,
19.7815795918341,20.607565451544,21.4335513112539,23.0855230306737,24.7374947500936,
26.3894664695134,26.5306282055506),.UNSPECIFIED.) ;
#516=B_SPLINE_CURVE_WITH_KNOTS('',3,(#58810,#58811,#58812,#58813,#58814,
#58815,#58816,#58817,#58818,#58819,#58820,#58821,#58822,#58823,#58824,#58825,
#58826,#58827,#58828,#58829,#58830,#58831,#58832,#58833,#58834,#58835,#58836,
#58837,#58838,#58839,#58840,#58841,#58842,#58843,#58844,#58845,#58846,#58847,
#58848,#58849,#58850,#58851,#58852,#58853,#58854,#58855,#58856,#58857,#58858,
#58859,#58860,#58861,#58862,#58863,#58864,#58865,#58866,#58867,#58868,#58869,
#58870,#58871,#58872,#58873,#58874,#58875,#58876,#58877,#58878,#58879,#58880,
#58881,#58882,#58883,#58884,#58885,#58886,#58887,#58888,#58889,#58890,#58891,
#58892,#58893,#58894,#58895,#58896,#58897,#58898,#58899),.UNSPECIFIED.,
 .F.,.F.,(4,2,2,2,2,2,2,2,2,2,2,2,2,2,2,2,2,2,2,2,2,2,2,2,2,2,2,2,2,2,2,
2,2,2,2,2,2,2,2,2,2,2,2,2,4),(1.51080998338119,1.65197171933602,3.30394343867204,
4.95591515800806,6.60788687734408,7.43387273701209,8.2598585966801,9.08584445634811,
9.91183031601612,10.3248232458501,10.7378161756841,11.1508091055181,11.5638020353521,
11.9767949651861,12.3897878950202,12.5962843599372,12.8027808248542,13.0092772897712,
13.2157737546882,13.4043865989579,13.4986930210928,13.5929994432276,13.6873058653625,
13.7344590764299,13.7816122874974,13.8287654985648,13.8759187096322,13.8994953151659,
13.9230719206997,13.9466485262334,13.9584368290002,13.9702251317671,13.9820286804365,
13.9938322291059,13.9997340034405,14.0056357777752,14.0085866649426,14.0115375521099,
14.0144884392773,14.0159638828609,14.0174393264446,14.0181982693009,14.0189572121572,
14.0197161550135,14.0200956264417),.UNSPECIFIED.) ;
#517=B_SPLINE_CURVE_WITH_KNOTS('',3,(#58904,#58905,#58906,#58907,#58908,
#58909,#58910,#58911,#58912,#58913,#58914,#58915,#58916,#58917,#58918,#58919,
#58920,#58921,#58922,#58923,#58924,#58925,#58926,#58927,#58928,#58929,#58930,
#58931,#58932,#58933,#58934,#58935,#58936,#58937,#58938,#58939,#58940,#58941,
#58942,#58943,#58944,#58945,#58946,#58947,#58948,#58949,#58950,#58951,#58952,
#58953,#58954,#58955,#58956,#58957,#58958,#58959,#58960,#58961,#58962,#58963,
#58964,#58965,#58966,#58967,#58968,#58969,#58970,#58971,#58972,#58973,#58974,
#58975,#58976,#58977,#58978,#58979,#58980,#58981,#58982,#58983,#58984,#58985,
#58986,#58987,#58988,#58989,#58990,#58991),.UNSPECIFIED.,.F.,.F.,(4,2,2,
2,2,2,2,2,2,2,2,2,2,2,2,2,2,2,2,2,2,2,2,2,2,2,2,2,2,2,2,2,2,2,2,2,2,2,2,
2,2,2,2,4),(14.1547675259996,14.1551502230512,14.1559156171545,14.1566810112577,
14.1574464053609,14.1589345873031,14.1604227692453,14.1633991331296,14.1663754970139,
14.1693518608982,14.1753045886669,14.1812573164355,14.1931627719728,14.2050682275101,
14.2169592360564,14.2288502446028,14.2526322616954,14.2764142787881,14.3001962958808,
14.3477603300661,14.3953243642515,14.4428883984368,14.4904524326222,14.5855805009929,
14.6807085693636,14.7758366377343,14.9660927744757,15.1745644176806,15.3830360608854,
15.5915077040903,15.7999793472952,16.216922633705,16.6338659201147,17.0508092065245,
17.4677524929342,17.884695779344,18.3016390657537,19.1355256385732,19.9694122113928,
20.8032987842123,21.6371853570318,23.3049585026708,24.9727316483098,26.6605889239056),
 .UNSPECIFIED.) ;
#518=B_SPLINE_CURVE_WITH_KNOTS('',3,(#58992,#58993,#58994,#58995,#58996,
#58997,#58998,#58999,#59000,#59001,#59002,#59003,#59004,#59005,#59006,#59007,
#59008,#59009,#59010,#59011,#59012,#59013,#59014,#59015,#59016,#59017,#59018,
#59019,#59020,#59021,#59022,#59023,#59024,#59025,#59026,#59027,#59028,#59029,
#59030,#59031,#59032,#59033,#59034,#59035,#59036,#59037,#59038,#59039,#59040,
#59041,#59042,#59043,#59044,#59045,#59046,#59047,#59048,#59049,#59050,#59051,
#59052,#59053,#59054,#59055,#59056,#59057,#59058,#59059,#59060,#59061,#59062,
#59063,#59064,#59065,#59066,#59067,#59068,#59069,#59070,#59071,#59072,#59073,
#59074,#59075,#59076,#59077,#59078,#59079,#59080,#59081),.UNSPECIFIED.,
 .F.,.F.,(4,2,2,2,2,2,2,2,2,2,2,2,2,2,2,2,2,2,2,2,2,2,2,2,2,2,2,2,2,2,2,
2,2,2,2,2,2,2,2,2,2,2,2,2,4),(1.647689015682,1.66777314561885,3.33554629123771,
5.00331943685656,6.67109258247542,7.50497915528485,8.33886572809427,9.1727523009037,
10.0066388737131,10.4235821601178,10.8405254465226,11.2574687329273,11.674412019332,
12.0913553057367,12.5082985921414,12.7167702353438,12.9252418785461,13.1337135217485,
13.3421851649508,13.5324413017259,13.6275693701134,13.7226974385009,13.8178255068884,
13.8653895410822,13.912953575276,13.9605176094697,14.0080816436635,14.0318636607604,
14.0556456778572,14.0794276949541,14.0913187035026,14.103209712051,14.1151151676442,
14.1270206232375,14.1329733510341,14.1389260788307,14.141902442729,14.1448788066273,
14.1478551705256,14.1493433524748,14.1508315344239,14.151596927938,14.1523623214521,
14.1531277149662,14.1535104117233),.UNSPECIFIED.) ;
#519=B_SPLINE_CURVE_WITH_KNOTS('',3,(#59086,#59087,#59088,#59089,#59090,
#59091,#59092,#59093,#59094,#59095,#59096,#59097,#59098,#59099,#59100,#59101,
#59102,#59103,#59104,#59105,#59106,#59107,#59108,#59109,#59110,#59111,#59112,
#59113,#59114,#59115,#59116,#59117,#59118,#59119,#59120,#59121,#59122,#59123,
#59124,#59125,#59126,#59127,#59128,#59129,#59130,#59131,#59132,#59133,#59134,
#59135,#59136,#59137,#59138,#59139,#59140,#59141,#59142,#59143,#59144,#59145,
#59146,#59147,#59148,#59149,#59150,#59151,#59152,#59153,#59154,#59155,#59156,
#59157,#59158,#59159,#59160,#59161,#59162,#59163,#59164,#59165,#59166,#59167,
#59168,#59169,#59170,#59171,#59172,#59173),.UNSPECIFIED.,.F.,.F.,(4,2,2,
2,2,2,2,2,2,2,2,2,2,2,2,2,2,2,2,2,2,2,2,2,2,2,2,2,2,2,2,2,2,2,2,2,2,2,2,
2,2,2,2,4),(14.1455560200775,14.1459384944968,14.1467034433353,14.1474683921739,
14.1482333410125,14.149720644208,14.1512079474035,14.1541825537946,14.1571571601856,
14.1601317665767,14.1660809793588,14.1720301921409,14.1839286177052,14.1958270432694,
14.2077109663326,14.2195948893957,14.2433627355219,14.2671305816482,14.2908984277745,
14.338434120027,14.3859698122795,14.433505504532,14.4810411967845,14.5761125812896,
14.6711839657946,14.7662553502996,14.9563981193097,15.1647333928276,15.3730686663455,
15.5814039398634,15.7897392133813,16.206409760417,16.6230803074528,17.0397508544886,
17.4564214015244,17.8730919485602,18.2897624955959,19.1231035896675,19.9564446837391,
20.7897857778106,21.6231268718822,23.2898090600253,24.9564912481684,26.6516061658473),
 .UNSPECIFIED.) ;
#520=B_SPLINE_CURVE_WITH_KNOTS('',3,(#59174,#59175,#59176,#59177,#59178,
#59179,#59180,#59181,#59182,#59183,#59184,#59185,#59186,#59187,#59188,#59189,
#59190,#59191,#59192,#59193,#59194,#59195,#59196,#59197,#59198,#59199,#59200,
#59201,#59202,#59203,#59204,#59205,#59206,#59207,#59208,#59209,#59210,#59211,
#59212,#59213,#59214,#59215,#59216,#59217,#59218,#59219,#59220,#59221,#59222,
#59223,#59224,#59225,#59226,#59227,#59228,#59229,#59230,#59231,#59232,#59233,
#59234,#59235,#59236,#59237,#59238,#59239,#59240,#59241,#59242,#59243,#59244,
#59245,#59246,#59247,#59248,#59249,#59250,#59251,#59252,#59253,#59254,#59255,
#59256,#59257,#59258,#59259,#59260,#59261,#59262,#59263),.UNSPECIFIED.,
 .F.,.F.,(4,2,2,2,2,2,2,2,2,2,2,2,2,2,2,2,2,2,2,2,2,2,2,2,2,2,2,2,2,2,2,
2,2,2,2,2,2,2,2,2,2,2,2,2,4),(1.63824945860653,1.66668218810681,3.33336437621363,
5.00004656432044,6.66672875242725,7.50006984648066,8.33341094053407,9.16675203458747,
10.0000931286409,10.4167636756676,10.8334342226943,11.250104769721,11.6667753167477,
12.0834458637744,12.5001164108011,12.7084516843145,12.9167869578278,13.1251222313412,
13.3334575048545,13.5236002737055,13.618671658131,13.7137430425566,13.8088144269821,
13.8563501191948,13.9038858114076,13.9514215036203,13.9989571958331,14.0227250419395,
14.0464928880459,14.0702607341522,14.0821446572054,14.0940285802586,14.105927006162,
14.1178254320655,14.1237746450172,14.1297238579689,14.1326984644448,14.1356730709206,
14.1386476773965,14.1401349806344,14.1416222838723,14.1423872326495,14.1431521814267,
14.1439171302038,14.1442996045924),.UNSPECIFIED.) ;
#521=B_SPLINE_CURVE_WITH_KNOTS('',3,(#59268,#59269,#59270,#59271,#59272,
#59273,#59274,#59275,#59276,#59277,#59278,#59279,#59280,#59281,#59282,#59283,
#59284,#59285,#59286,#59287,#59288,#59289,#59290,#59291,#59292,#59293,#59294,
#59295,#59296,#59297,#59298,#59299,#59300,#59301,#59302,#59303,#59304,#59305,
#59306,#59307,#59308,#59309,#59310,#59311,#59312,#59313,#59314,#59315,#59316,
#59317,#59318,#59319,#59320,#59321,#59322,#59323,#59324,#59325,#59326,#59327,
#59328,#59329,#59330,#59331,#59332,#59333,#59334,#59335,#59336,#59337,#59338,
#59339,#59340,#59341,#59342,#59343,#59344,#59345,#59346,#59347,#59348,#59349,
#59350,#59351,#59352,#59353,#59354,#59355,#59356,#59357),.UNSPECIFIED.,
 .F.,.F.,(4,2,2,2,2,2,2,2,2,2,2,2,2,2,2,2,2,2,2,2,2,2,2,2,2,2,2,2,2,2,2,
2,2,2,2,2,2,2,2,2,2,2,2,2,4),(13.9958308278144,13.9962096816943,13.9969673894541,
13.997725097214,13.9984828049738,13.9999558104743,14.0014288159747,14.0043748269757,
14.0073208379766,14.0102668489776,14.0161588709794,14.0220508929813,14.0338349369851,
14.0456189809888,14.0573876272289,14.069156273469,14.0926935659491,14.1162308584293,
14.1397681509095,14.1868427358698,14.2339173208301,14.2809919057904,14.3280664907508,
14.4222156606714,14.5163648305921,14.6105140005127,14.798812340354,15.00493115794,
15.2110499755261,15.4171687931121,15.6232876106981,16.0355252458701,16.4477628810421,
16.8600005162142,17.2722381513862,17.6844757865582,18.0967134217303,18.9211886920743,
19.7456639624184,20.5701392327624,21.3946145031065,23.0435650437946,24.6925155844827,
26.3414661251708,26.5058166413175),.UNSPECIFIED.) ;
#522=B_SPLINE_CURVE_WITH_KNOTS('',3,(#59358,#59359,#59360,#59361,#59362,
#59363,#59364,#59365,#59366,#59367,#59368,#59369,#59370,#59371,#59372,#59373,
#59374,#59375,#59376,#59377,#59378,#59379,#59380,#59381,#59382,#59383,#59384,
#59385,#59386,#59387,#59388,#59389,#59390,#59391,#59392,#59393,#59394,#59395,
#59396,#59397,#59398,#59399,#59400,#59401,#59402,#59403,#59404,#59405,#59406,
#59407,#59408,#59409,#59410,#59411,#59412,#59413,#59414,#59415,#59416,#59417,
#59418,#59419,#59420,#59421,#59422,#59423,#59424,#59425,#59426,#59427,#59428,
#59429,#59430,#59431,#59432,#59433,#59434,#59435,#59436,#59437,#59438,#59439,
#59440,#59441,#59442,#59443,#59444,#59445,#59446,#59447),.UNSPECIFIED.,
 .F.,.F.,(4,2,2,2,2,2,2,2,2,2,2,2,2,2,2,2,2,2,2,2,2,2,2,2,2,2,2,2,2,2,2,
2,2,2,2,2,2,2,2,2,2,2,2,2,4),(1.48460002454081,1.64895054064786,3.29790108129571,
4.94685162194357,6.59580216259142,7.42027743291535,8.24475270323928,9.06922797356321,
9.89370324388713,10.3059408790491,10.7181785142111,11.130416149373,11.542653784535,
11.954891419697,12.3671290548589,12.5732478724399,12.7793666900209,12.9854855076019,
13.1916043251828,13.3799026649428,13.4740518348228,13.5682010047028,13.6623501745829,
13.7094247595229,13.7564993444629,13.8035739294029,13.8506485143429,13.8741858068129,
13.8977230992829,13.9212603917529,13.9330290379879,13.9447976842229,13.9565817286828,
13.9683657731427,13.9742577953726,13.9801498176026,13.9830958287176,13.9860418398326,
13.9889878509475,13.990460856505,13.9919338620625,13.9926915691657,13.9934492762689,
13.9942069833721,13.9945858369238),.UNSPECIFIED.) ;
#523=B_SPLINE_CURVE_WITH_KNOTS('',3,(#59452,#59453,#59454,#59455,#59456,
#59457,#59458,#59459,#59460,#59461,#59462,#59463,#59464,#59465,#59466,#59467,
#59468,#59469,#59470,#59471,#59472,#59473,#59474,#59475,#59476,#59477,#59478,
#59479,#59480,#59481,#59482,#59483,#59484,#59485,#59486,#59487,#59488,#59489,
#59490,#59491,#59492,#59493,#59494,#59495,#59496,#59497,#59498,#59499,#59500,
#59501,#59502,#59503,#59504,#59505,#59506,#59507,#59508,#59509,#59510,#59511,
#59512,#59513,#59514,#59515,#59516,#59517,#59518,#59519,#59520,#59521,#59522,
#59523,#59524,#59525,#59526,#59527,#59528,#59529,#59530,#59531,#59532,#59533,
#59534,#59535,#59536,#59537,#59538,#59539,#59540),.UNSPECIFIED.,.F.,.F.,
(4,2,2,2,2,2,2,2,2,2,2,2,2,2,2,2,2,2,2,2,2,2,2,2,2,2,2,2,2,2,2,2,2,2,2,
2,2,2,2,2,2,2,2,1,4),(14.0868029194625,14.0871839745037,14.087946084586,
14.0887081946684,14.0894703047507,14.0909520006773,14.0924336966038,14.095397088457,
14.0983604803101,14.1013238721633,14.1072506558696,14.1131774395758,14.1250310069884,
14.136884574401,14.148723286499,14.160561998597,14.184239422793,14.207916846989,
14.231594271185,14.2789491195771,14.3263039679691,14.3736588163611,14.4210136647531,
14.5157233615372,14.6104330583212,14.7051427551052,14.8945621486733,15.1020276449097,
15.3094931411461,15.5169586373825,15.7244241336189,16.1393551260918,16.5542861185646,
16.9692171110374,17.3841481035102,17.799079095983,18.2140100884559,19.0438720734015,
19.8737340583471,20.7035960432928,21.5334580282384,23.1931819981297,24.852905968021,
26.5126299379123,26.5943480659534),.UNSPECIFIED.) ;
#524=B_SPLINE_CURVE_WITH_KNOTS('',3,(#59541,#59542,#59543,#59544,#59545,
#59546,#59547,#59548,#59549,#59550,#59551,#59552,#59553,#59554,#59555,#59556,
#59557,#59558,#59559,#59560,#59561,#59562,#59563,#59564,#59565,#59566,#59567,
#59568,#59569,#59570,#59571,#59572,#59573,#59574,#59575,#59576,#59577,#59578,
#59579,#59580,#59581,#59582,#59583,#59584,#59585,#59586,#59587,#59588,#59589,
#59590,#59591,#59592,#59593,#59594,#59595,#59596,#59597,#59598,#59599,#59600,
#59601,#59602,#59603,#59604,#59605,#59606,#59607,#59608,#59609,#59610,#59611,
#59612,#59613,#59614,#59615,#59616,#59617,#59618,#59619,#59620,#59621,#59622,
#59623,#59624,#59625,#59626,#59627,#59628,#59629,#59630),.UNSPECIFIED.,
 .F.,.F.,(4,2,2,2,2,2,2,2,2,2,2,2,2,2,2,2,2,2,2,2,2,2,2,2,2,2,2,2,2,2,2,
2,2,2,2,2,2,2,2,2,2,2,2,2,4),(1.57800584185108,1.65972396994431,3.31944793988862,
4.97917190983293,6.63889587977724,7.4687578647494,8.29861984972155,9.12848183469371,
9.95834381966586,10.3732748121519,10.788205804638,11.2031367971241,11.6180677896102,
12.0329987820963,12.4479297745823,12.6553952708254,12.8628607670684,13.0703262633114,
13.2777917595545,13.4672111529754,13.5619208496858,13.6566305463962,13.7513402431067,
13.7986950914619,13.8460499398171,13.8934047881723,13.9407596365275,13.9644370607051,
13.9881144848827,14.0117919090603,14.0236306211492,14.035469333238,14.0473229006196,
14.0591764680012,14.065103251692,14.0710300353828,14.0739934272282,14.0769568190737,
14.0799202109191,14.0814019068418,14.0828836027645,14.0836457122491,14.0844078217337,
14.0851699312182,14.0855509859605),.UNSPECIFIED.) ;
#525=B_SPLINE_CURVE_WITH_KNOTS('',3,(#59635,#59636,#59637,#59638,#59639,
#59640,#59641,#59642,#59643,#59644,#59645,#59646,#59647,#59648,#59649,#59650,
#59651,#59652,#59653,#59654,#59655,#59656,#59657,#59658,#59659,#59660,#59661,
#59662,#59663,#59664,#59665,#59666,#59667,#59668,#59669,#59670,#59671,#59672,
#59673,#59674,#59675,#59676,#59677,#59678,#59679,#59680,#59681,#59682,#59683,
#59684,#59685,#59686,#59687,#59688,#59689,#59690,#59691,#59692,#59693,#59694,
#59695,#59696,#59697,#59698,#59699,#59700,#59701,#59702,#59703,#59704,#59705,
#59706,#59707,#59708,#59709,#59710,#59711,#59712,#59713,#59714,#59715,#59716,
#59717,#59718,#59719,#59720,#59721,#59722),.UNSPECIFIED.,.F.,.F.,(4,2,2,
2,2,2,2,2,2,2,2,2,2,2,2,2,2,2,2,2,2,2,2,2,2,2,2,2,2,2,2,2,2,2,2,2,2,2,2,
2,2,2,2,4),(14.1686729967438,14.1690560293449,14.1698220945472,14.1705881597495,
14.1713542249518,14.1728437331919,14.1743332414321,14.1773122579123,14.1802912743926,
14.1832702908729,14.1892283238334,14.1951863567939,14.207102422715,14.219018488636,
14.2309201917689,14.2428218949018,14.2666253011676,14.2904287074334,14.3142321136991,
14.3618389262307,14.4094457387622,14.4570525512938,14.5046593638254,14.5998729888885,
14.6950866139516,14.7903002390147,14.980727489141,15.1894049942478,15.3980824993547,
15.6067600044615,15.8154375095683,16.232792519782,16.6501475299957,17.0675025402094,
17.4848575504231,17.9022125606368,18.3195675708505,19.1542775912779,19.9889876117052,
20.8236976321326,21.65840765256,23.3278276934148,24.9972477342695,26.6741519513281),
 .UNSPECIFIED.) ;
#526=B_SPLINE_CURVE_WITH_KNOTS('',3,(#59723,#59724,#59725,#59726,#59727,
#59728,#59729,#59730,#59731,#59732,#59733,#59734,#59735,#59736,#59737,#59738,
#59739,#59740,#59741,#59742,#59743,#59744,#59745,#59746,#59747,#59748,#59749,
#59750,#59751,#59752,#59753,#59754,#59755,#59756,#59757,#59758,#59759,#59760,
#59761,#59762,#59763,#59764,#59765,#59766,#59767,#59768,#59769,#59770,#59771,
#59772,#59773,#59774,#59775,#59776,#59777,#59778,#59779,#59780,#59781,#59782,
#59783,#59784,#59785,#59786,#59787,#59788,#59789,#59790,#59791,#59792,#59793,
#59794,#59795,#59796,#59797,#59798,#59799,#59800,#59801,#59802,#59803,#59804,
#59805,#59806,#59807,#59808,#59809,#59810,#59811,#59812),.UNSPECIFIED.,
 .F.,.F.,(4,2,2,2,2,2,2,2,2,2,2,2,2,2,2,2,2,2,2,2,2,2,2,2,2,2,2,2,2,2,2,
2,2,2,2,2,2,2,2,2,2,2,2,2,4),(1.66193586464827,1.66942004071743,3.33884008143485,
5.00826012215228,6.6776801628697,7.51239018322842,8.34710020358713,9.18181022394584,
10.0165202443046,10.4338752544839,10.8512302646633,11.2685852748426,11.685940285022,
12.1032952952013,12.5206503053807,12.7293278104704,12.93800531556,13.1466828206497,
13.3553603257394,13.5457875760677,13.6410012012319,13.736214826396,13.8314284515602,
13.8790352641423,13.9266420767244,13.9742488893064,14.0218557018885,14.0456591081796,
14.0694625144706,14.0932659207616,14.1051676239072,14.1170693270527,14.1289853931201,
14.1409014591876,14.1468594922213,14.152817525255,14.1557965417719,14.1587755582887,
14.1617545748056,14.163244083064,14.1647335913224,14.1654996565209,14.1662657217195,
14.167031786918,14.1674148195172),.UNSPECIFIED.) ;
#527=B_SPLINE_CURVE_WITH_KNOTS('',3,(#59817,#59818,#59819,#59820,#59821,
#59822,#59823,#59824,#59825,#59826,#59827,#59828,#59829,#59830,#59831,#59832,
#59833,#59834,#59835,#59836,#59837,#59838,#59839,#59840,#59841,#59842,#59843,
#59844,#59845,#59846,#59847,#59848,#59849,#59850,#59851,#59852,#59853,#59854,
#59855,#59856,#59857,#59858,#59859,#59860,#59861,#59862,#59863,#59864,#59865,
#59866,#59867,#59868,#59869,#59870,#59871,#59872,#59873,#59874,#59875,#59876,
#59877,#59878,#59879,#59880,#59881,#59882,#59883,#59884,#59885,#59886,#59887,
#59888,#59889,#59890,#59891,#59892,#59893,#59894,#59895,#59896,#59897,#59898,
#59899,#59900,#59901,#59902,#59903,#59904,#59905),.UNSPECIFIED.,.F.,.F.,
(4,2,2,2,2,2,2,2,2,2,2,2,2,2,2,2,2,2,2,2,2,2,2,2,2,2,2,2,2,2,2,2,2,2,2,
2,2,2,2,2,2,2,2,1,4),(14.1046764419688,14.1050579284097,14.1058209012915,
14.1065838741732,14.107346847055,14.1088302492569,14.1103136514588,14.1132804558627,
14.1162472602665,14.1192140646704,14.1251476734781,14.1310812822858,14.1429484999011,
14.1548157175165,14.1666681867437,14.1785206559708,14.2022255944251,14.2259305328793,
14.2496354713336,14.2970453482421,14.3444552251506,14.3918651020592,14.4392749789677,
14.5340947327848,14.6289144866018,14.7237342404189,14.913373748053,15.1211038392599,
15.3288339304668,15.5365640216737,15.7442941128806,16.1597542952945,16.5752144777083,
16.9906746601222,17.406134842536,17.8215950249498,18.2370552073637,19.0679755721913,
19.898895937019,20.7298163018467,21.5607366666744,23.2225773963297,24.884418125985,
26.5462588556404,26.6117601500675),.UNSPECIFIED.) ;
#528=B_SPLINE_CURVE_WITH_KNOTS('',3,(#59906,#59907,#59908,#59909,#59910,
#59911,#59912,#59913,#59914,#59915,#59916,#59917,#59918,#59919,#59920,#59921,
#59922,#59923,#59924,#59925,#59926,#59927,#59928,#59929,#59930,#59931,#59932,
#59933,#59934,#59935,#59936,#59937,#59938,#59939,#59940,#59941,#59942,#59943,
#59944,#59945,#59946,#59947,#59948,#59949,#59950,#59951,#59952,#59953,#59954,
#59955,#59956,#59957,#59958,#59959,#59960,#59961,#59962,#59963,#59964,#59965,
#59966,#59967,#59968,#59969,#59970,#59971,#59972,#59973,#59974,#59975,#59976,
#59977,#59978,#59979,#59980,#59981,#59982,#59983,#59984,#59985,#59986,#59987,
#59988,#59989,#59990,#59991,#59992,#59993,#59994,#59995),.UNSPECIFIED.,
 .F.,.F.,(4,2,2,2,2,2,2,2,2,2,2,2,2,2,2,2,2,2,2,2,2,2,2,2,2,2,2,2,2,2,2,
2,2,2,2,2,2,2,2,2,2,2,2,2,4),(1.59633943522071,1.66184072925037,3.32368145850075,
4.98552218775112,6.6473629170015,7.47828328162668,8.30920364625187,9.14012401087706,
9.97104437550225,10.3865045578148,10.8019647401274,11.21742492244,11.6328851047526,
12.0483452870652,12.4638054693778,12.6715355605341,12.8792656516904,13.0869957428467,
13.294725834003,13.4843653426121,13.5791850969167,13.6740048512212,13.7688246055258,
13.8162344826781,13.8636443598303,13.9110542369826,13.9584641141349,13.982169052711,
14.0058739912872,14.0295789298633,14.0414313991514,14.0532838684395,14.0651510853518,
14.0770183022642,14.0829519107204,14.0888855191766,14.0918523234047,14.0948191276328,
14.0977859318609,14.0992693339749,14.100752736089,14.1015157095784,14.1022786830678,
14.1030416565573,14.103423143302),.UNSPECIFIED.) ;
#529=B_SPLINE_CURVE_WITH_KNOTS('',3,(#60000,#60001,#60002,#60003,#60004,
#60005,#60006,#60007,#60008,#60009,#60010,#60011,#60012,#60013,#60014,#60015,
#60016,#60017,#60018,#60019,#60020,#60021,#60022,#60023,#60024,#60025,#60026,
#60027,#60028,#60029,#60030,#60031,#60032,#60033,#60034,#60035,#60036,#60037,
#60038,#60039,#60040,#60041,#60042,#60043,#60044,#60045,#60046,#60047,#60048,
#60049,#60050,#60051,#60052,#60053,#60054,#60055,#60056,#60057,#60058,#60059,
#60060,#60061,#60062,#60063,#60064,#60065,#60066,#60067,#60068,#60069,#60070,
#60071,#60072,#60073,#60074,#60075,#60076,#60077,#60078,#60079,#60080,#60081,
#60082,#60083,#60084,#60085,#60086,#60087,#60088,#60089),.UNSPECIFIED.,
 .F.,.F.,(4,2,2,2,2,2,2,2,2,2,2,2,2,2,2,2,2,2,2,2,2,2,2,2,2,2,2,2,2,2,2,
2,2,2,2,2,2,2,2,2,2,2,2,2,4),(13.9686134554172,13.9689916509333,13.9697480419656,
13.9705044329979,13.9712608240301,13.9727312275229,13.9742016310156,13.9771424380011,
13.9800832449866,13.9830240519721,13.9889056659431,13.994787279914,14.006550507856,
14.0183137357979,14.0300614047906,14.0418090737832,14.0653044117685,14.0887997497538,
14.1122950877391,14.1592857637096,14.2062764396802,14.2532671156508,14.3002577916213,
14.3942391435625,14.4882204955036,14.5822018474448,14.770164551327,14.9758804803237,
15.1815964093203,15.3873123383169,15.5930282673136,16.0044601253068,16.4158919833001,
16.8273238412934,17.2387556992867,17.65018755728,18.0616194152732,18.8844831312598,
19.7073468472463,20.5302105632329,21.3530742792195,22.9988017111926,24.6445291431657,
26.2902565751388,26.4793600117376),.UNSPECIFIED.) ;
#530=B_SPLINE_CURVE_WITH_KNOTS('',3,(#60090,#60091,#60092,#60093,#60094,
#60095,#60096,#60097,#60098,#60099,#60100,#60101,#60102,#60103,#60104,#60105,
#60106,#60107,#60108,#60109,#60110,#60111,#60112,#60113,#60114,#60115,#60116,
#60117,#60118,#60119,#60120,#60121,#60122,#60123,#60124,#60125,#60126,#60127,
#60128,#60129,#60130,#60131,#60132,#60133,#60134,#60135,#60136,#60137,#60138,
#60139,#60140,#60141,#60142,#60143,#60144,#60145,#60146,#60147,#60148,#60149,
#60150,#60151,#60152,#60153,#60154,#60155,#60156,#60157,#60158,#60159,#60160,
#60161,#60162,#60163,#60164,#60165,#60166,#60167,#60168,#60169,#60170,#60171,
#60172,#60173,#60174,#60175,#60176,#60177,#60178,#60179),.UNSPECIFIED.,
 .F.,.F.,(4,2,2,2,2,2,2,2,2,2,2,2,2,2,2,2,2,2,2,2,2,2,2,2,2,2,2,2,2,2,2,
2,2,2,2,2,2,2,2,2,2,2,2,2,4),(1.45662399537573,1.64572743206755,3.29145486413511,
4.93718229620266,6.58290972827021,7.40577344430399,8.22863716033777,9.05150087637154,
9.87436459240532,10.2857964504222,10.6972283084391,11.108660166456,11.5200920244729,
11.9315238824898,12.3429557405066,12.5486716695151,12.7543875985235,12.960103527532,
13.1658194565404,13.3537821600959,13.4477635118736,13.5417448636514,13.6357262154291,
13.682716891318,13.7297075672069,13.7766982430957,13.8236889189846,13.847184256929,
13.8706795948735,13.8941749328179,13.9059226017901,13.9176702707623,13.9294334980288,
13.9411967252953,13.9470783389286,13.9529599525619,13.9559007593785,13.9588415661951,
13.9617823730117,13.9632527764201,13.9647231798284,13.9654795709265,13.9662359620246,
13.9669923531227,13.9673705486717),.UNSPECIFIED.) ;
#531=B_SPLINE_CURVE_WITH_KNOTS('',3,(#60184,#60185,#60186,#60187,#60188,
#60189,#60190,#60191,#60192,#60193,#60194,#60195,#60196,#60197,#60198,#60199,
#60200,#60201,#60202,#60203,#60204,#60205,#60206,#60207,#60208,#60209,#60210,
#60211,#60212,#60213,#60214,#60215,#60216,#60217,#60218,#60219,#60220,#60221,
#60222,#60223,#60224,#60225,#60226,#60227,#60228,#60229,#60230,#60231,#60232,
#60233,#60234,#60235,#60236,#60237,#60238,#60239,#60240,#60241,#60242,#60243,
#60244,#60245,#60246,#60247,#60248,#60249,#60250,#60251,#60252,#60253,#60254,
#60255,#60256,#60257,#60258,#60259,#60260,#60261,#60262,#60263,#60264,#60265,
#60266,#60267,#60268,#60269,#60270,#60271),.UNSPECIFIED.,.F.,.F.,(4,2,2,
2,2,2,2,2,2,2,2,2,2,2,2,2,2,2,2,2,2,2,2,2,2,2,2,2,2,2,2,2,2,2,2,2,2,2,2,
2,2,2,2,4),(14.1341071652671,14.1344893630051,14.1352537584812,14.1360181539573,
14.1367825494334,14.1382687602835,14.1397549711335,14.1427273928336,14.1456998145336,
14.1486722362337,14.1546170796338,14.160561923034,14.1724516098342,14.1843412966345,
14.1962164121656,14.2080915276967,14.2318417587589,14.2555919898211,14.2793422208833,
14.3268426830077,14.3743431451322,14.4218436072566,14.469344069381,14.5643449936298,
14.6593459178787,14.7543468421275,14.9443486906252,15.1525144733886,15.3606802561521,
15.5688460389155,15.777011821679,16.1933433872059,16.6096749527328,17.0260065182597,
17.4423380837866,17.8586696493135,18.2750012148404,19.1076643458942,19.940327476948,
20.7729906080018,21.6056537390555,23.2709800011631,24.9363062632707,26.6404437310253),
 .UNSPECIFIED.) ;
#532=B_SPLINE_CURVE_WITH_KNOTS('',3,(#60272,#60273,#60274,#60275,#60276,
#60277,#60278,#60279,#60280,#60281,#60282,#60283,#60284,#60285,#60286,#60287,
#60288,#60289,#60290,#60291,#60292,#60293,#60294,#60295,#60296,#60297,#60298,
#60299,#60300,#60301,#60302,#60303,#60304,#60305,#60306,#60307,#60308,#60309,
#60310,#60311,#60312,#60313,#60314,#60315,#60316,#60317,#60318,#60319,#60320,
#60321,#60322,#60323,#60324,#60325,#60326,#60327,#60328,#60329,#60330,#60331,
#60332,#60333,#60334,#60335,#60336,#60337,#60338,#60339,#60340,#60341,#60342,
#60343,#60344,#60345,#60346,#60347,#60348,#60349,#60350,#60351,#60352,#60353,
#60354,#60355,#60356,#60357,#60358,#60359,#60360,#60361),.UNSPECIFIED.,
 .F.,.F.,(4,2,2,2,2,2,2,2,2,2,2,2,2,2,2,2,2,2,2,2,2,2,2,2,2,2,2,2,2,2,2,
2,2,2,2,2,2,2,2,2,2,2,2,2,4),(1.62651505645876,1.66532626201344,3.33065252402689,
4.99597878604033,6.66130504805378,7.4939681790605,8.32663131006722,9.15929444107394,
9.99195757208066,10.408289137584,10.8246207030874,11.2409522685907,11.6572838340941,
12.0736153995975,12.4899469651008,12.6981127478525,12.9062785306042,13.1144443133559,
13.3226100961076,13.512611944883,13.6076128692707,13.7026137936585,13.7976147180462,
13.84511518024,13.8926156424339,13.9401161046278,13.9876165668216,14.0113667979186,
14.0351170290155,14.0588672601124,14.0707423756609,14.0826174912093,14.0945071774897,
14.10639686377,14.1123417069102,14.1182865500503,14.1212589716204,14.1242313931905,
14.1272038147606,14.1286900255456,14.1301762363306,14.1309406319289,14.1317050275272,
14.1324694231255,14.1328516209246),.UNSPECIFIED.) ;
#533=B_SPLINE_CURVE_WITH_KNOTS('',3,(#60366,#60367,#60368,#60369,#60370,
#60371,#60372,#60373,#60374,#60375,#60376,#60377,#60378,#60379,#60380,#60381,
#60382,#60383,#60384,#60385,#60386,#60387,#60388,#60389,#60390,#60391,#60392,
#60393,#60394,#60395,#60396,#60397,#60398,#60399,#60400,#60401,#60402,#60403,
#60404,#60405,#60406,#60407,#60408,#60409,#60410,#60411,#60412,#60413,#60414,
#60415,#60416,#60417,#60418,#60419,#60420,#60421,#60422,#60423,#60424,#60425,
#60426,#60427,#60428,#60429,#60430,#60431,#60432,#60433,#60434,#60435,#60436,
#60437,#60438,#60439,#60440,#60441,#60442,#60443,#60444,#60445,#60446,#60447,
#60448,#60449,#60450,#60451,#60452,#60453),.UNSPECIFIED.,.F.,.F.,(4,2,2,
2,2,2,2,2,2,2,2,2,2,2,2,2,2,2,2,2,2,2,2,2,2,2,2,2,2,2,2,2,2,2,2,2,2,2,2,
2,2,2,2,4),(14.16170696931,14.1620898339262,14.1628555631585,14.1636212923909,
14.1643870216232,14.1658758654799,14.1673647093366,14.17034239705,14.1733200847634,
14.1762977724768,14.1822531479036,14.1882085233304,14.200119274184,14.2120300250377,
14.2239263708663,14.2358227166949,14.2596154083521,14.2834081000093,14.3072007916665,
14.354786174981,14.4023715582954,14.4499569416099,14.4975423249243,14.5927130915532,
14.6878838581821,14.7830546248109,14.9733961580687,15.1819705352013,15.390544912334,
15.5991192894666,15.8076936665992,16.2248424208645,16.6419911751297,17.059139929395,
17.4762886836602,17.8934374379255,18.3105861921908,19.1448837007213,19.9791812092518,
20.8134787177823,21.6477762263128,23.3163712433738,24.9849662604349,26.6673570370797),
 .UNSPECIFIED.) ;
#534=B_SPLINE_CURVE_WITH_KNOTS('',3,(#60454,#60455,#60456,#60457,#60458,
#60459,#60460,#60461,#60462,#60463,#60464,#60465,#60466,#60467,#60468,#60469,
#60470,#60471,#60472,#60473,#60474,#60475,#60476,#60477,#60478,#60479,#60480,
#60481,#60482,#60483,#60484,#60485,#60486,#60487,#60488,#60489,#60490,#60491,
#60492,#60493,#60494,#60495,#60496,#60497,#60498,#60499,#60500,#60501,#60502,
#60503,#60504,#60505,#60506,#60507,#60508,#60509,#60510,#60511,#60512,#60513,
#60514,#60515,#60516,#60517,#60518,#60519,#60520,#60521,#60522,#60523,#60524,
#60525,#60526,#60527,#60528,#60529,#60530,#60531,#60532,#60533,#60534,#60535,
#60536,#60537,#60538,#60539,#60540,#60541,#60542,#60543),.UNSPECIFIED.,
 .F.,.F.,(4,2,2,2,2,2,2,2,2,2,2,2,2,2,2,2,2,2,2,2,2,2,2,2,2,2,2,2,2,2,2,
2,2,2,2,2,2,2,2,2,2,2,2,2,4),(1.65479925748035,1.6685950172178,3.3371900344356,
5.00578505165339,6.67438006887119,7.50867757748009,8.34297508608899,9.17727259469789,
10.0115701033068,10.4287188576112,10.8458676119157,11.2630163662201,11.6801651205246,
12.097313874829,12.5144626291335,12.7230370062857,12.9316113834379,13.1401857605902,
13.3487601377424,13.5391016710958,13.6342724377725,13.7294432044492,13.8246139711259,
13.8721993544642,13.9197847378026,13.9673701211409,14.0149555044792,14.0387481961484,
14.0625408878176,14.0863335794868,14.0982299253214,14.1101262711559,14.1220370214148,
14.1339477716737,14.1399031468032,14.1458585219326,14.1488362094973,14.1518138970621,
14.1547915846268,14.1562804284091,14.1577692721915,14.1585350011919,14.1593007301924,
14.1600664591929,14.1604493236931),.UNSPECIFIED.) ;
#535=B_SPLINE_CURVE_WITH_KNOTS('',3,(#60548,#60549,#60550,#60551,#60552,
#60553,#60554,#60555,#60556,#60557,#60558,#60559,#60560,#60561,#60562,#60563,
#60564,#60565,#60566,#60567,#60568,#60569,#60570,#60571,#60572,#60573,#60574,
#60575,#60576,#60577,#60578,#60579,#60580,#60581,#60582,#60583,#60584,#60585,
#60586,#60587,#60588,#60589,#60590,#60591,#60592,#60593,#60594,#60595,#60596,
#60597,#60598,#60599,#60600,#60601,#60602,#60603,#60604,#60605,#60606,#60607,
#60608,#60609,#60610,#60611,#60612,#60613,#60614,#60615,#60616,#60617,#60618,
#60619,#60620,#60621,#60622,#60623,#60624,#60625,#60626,#60627,#60628,#60629,
#60630,#60631,#60632,#60633,#60634,#60635,#60636,#60637),.UNSPECIFIED.,
 .F.,.F.,(4,2,2,2,2,2,2,2,2,2,2,2,2,2,2,2,2,2,2,2,2,2,2,2,2,2,2,2,2,2,2,
2,2,2,2,2,2,2,2,2,2,2,2,2,4),(14.0450621945841,14.0454422402384,14.0462023315469,
14.0469624228554,14.0477225141639,14.0492002238686,14.0506779335734,14.0536333529828,
14.0565887723922,14.0595441918017,14.0654550306206,14.0713658694395,14.0831875470772,
14.095009224715,14.1068157979037,14.1186223710924,14.1422355174697,14.1658486638471,
14.1894618102245,14.2366881029792,14.2839143957339,14.3311406884886,14.3783669812434,
14.4728195667528,14.5672721522623,14.6617247377717,14.8506299087907,15.0574774983924,
15.2643250879942,15.4711726775959,15.6780202671977,16.0917154464012,16.5054106256047,
16.9191058048082,17.3328009840117,17.7464961632152,18.1601913424187,18.9875817008258,
19.8149720592328,20.6423624176398,21.4697527760468,23.1245334928609,24.7793142096749,
26.434094926489,26.553707918216),.UNSPECIFIED.) ;
#536=B_SPLINE_CURVE_WITH_KNOTS('',3,(#60638,#60639,#60640,#60641,#60642,
#60643,#60644,#60645,#60646,#60647,#60648,#60649,#60650,#60651,#60652,#60653,
#60654,#60655,#60656,#60657,#60658,#60659,#60660,#60661,#60662,#60663,#60664,
#60665,#60666,#60667,#60668,#60669,#60670,#60671,#60672,#60673,#60674,#60675,
#60676,#60677,#60678,#60679,#60680,#60681,#60682,#60683,#60684,#60685,#60686,
#60687,#60688,#60689,#60690,#60691,#60692,#60693,#60694,#60695,#60696,#60697,
#60698,#60699,#60700,#60701,#60702,#60703,#60704,#60705,#60706,#60707,#60708,
#60709,#60710,#60711,#60712,#60713,#60714,#60715,#60716,#60717,#60718,#60719,
#60720,#60721,#60722,#60723,#60724,#60725,#60726,#60727),.UNSPECIFIED.,
 .F.,.F.,(4,2,2,2,2,2,2,2,2,2,2,2,2,2,2,2,2,2,2,2,2,2,2,2,2,2,2,2,2,2,2,
2,2,2,2,2,2,2,2,2,2,2,2,2,4),(1.53516772508572,1.65478071673876,3.30956143347751,
4.96434215021627,6.61912286695503,7.44651322532441,8.27390358369379,9.10129394206317,
9.92868430043254,10.3423794796172,10.7560746588019,11.1697698379866,11.5834650171713,
11.997160196356,12.4108553755407,12.617702965133,12.8245505547254,13.0313981443177,
13.2382457339101,13.4271509046269,13.5216034899854,13.6160560753438,13.7105086607022,
13.7577349533814,13.8049612460606,13.8521875387399,13.8994138314191,13.9230269777587,
13.9466401240983,13.9702532704379,13.9820598436077,13.9938664167775,14.0056880947879,
14.0175097727983,14.0234206118035,14.0293314508087,14.0322868703113,14.0352422898138,
14.0381977093164,14.0396754190677,14.041153128819,14.0419132202693,14.0426733117196,
14.04343340317,14.0438134488951),.UNSPECIFIED.) ;
#537=B_SPLINE_CURVE_WITH_KNOTS('',3,(#60732,#60733,#60734,#60735,#60736,
#60737,#60738,#60739,#60740,#60741,#60742,#60743,#60744,#60745,#60746,#60747,
#60748,#60749,#60750,#60751,#60752,#60753,#60754,#60755,#60756,#60757,#60758,
#60759,#60760,#60761,#60762,#60763,#60764,#60765,#60766,#60767,#60768,#60769,
#60770,#60771,#60772,#60773,#60774,#60775,#60776,#60777,#60778,#60779,#60780,
#60781,#60782,#60783,#60784,#60785,#60786,#60787,#60788,#60789,#60790,#60791,
#60792,#60793,#60794,#60795,#60796,#60797,#60798,#60799,#60800,#60801,#60802,
#60803,#60804,#60805,#60806,#60807,#60808,#60809,#60810,#60811,#60812,#60813,
#60814,#60815,#60816,#60817,#60818,#60819),.UNSPECIFIED.,.F.,.F.,(4,2,2,
2,2,2,2,2,2,2,2,2,2,2,2,2,2,2,2,2,2,2,2,2,2,2,2,2,2,2,2,2,2,2,2,2,2,2,2,
2,2,2,2,4),(14.1204637958664,14.1208456641181,14.1216094006214,14.1223731371248,
14.1231368736281,14.1246217824304,14.1261066912327,14.1290765088373,14.1320463264419,
14.1350161440465,14.1409557792558,14.146895414465,14.1587746848834,14.1706539553018,
14.1825185736228,14.1943831919437,14.2181124285857,14.2418416652276,14.2655709018695,
14.3130293751534,14.3604878484372,14.4079463217211,14.4554047950049,14.5503217415727,
14.6452386881404,14.7401556347081,14.9299895278435,15.1379533334243,15.345917139005,
15.5538809445858,15.7618447501665,16.1777723613281,16.5936999724896,17.0096275836511,
17.4255551948126,17.8414828059741,18.2574104171357,19.0892656394587,19.9211208617817,
20.7529760841048,21.5848313064278,23.2485417510739,24.91225219572,26.6271447649371),
 .UNSPECIFIED.) ;
#538=B_SPLINE_CURVE_WITH_KNOTS('',3,(#60820,#60821,#60822,#60823,#60824,
#60825,#60826,#60827,#60828,#60829,#60830,#60831,#60832,#60833,#60834,#60835,
#60836,#60837,#60838,#60839,#60840,#60841,#60842,#60843,#60844,#60845,#60846,
#60847,#60848,#60849,#60850,#60851,#60852,#60853,#60854,#60855,#60856,#60857,
#60858,#60859,#60860,#60861,#60862,#60863,#60864,#60865,#60866,#60867,#60868,
#60869,#60870,#60871,#60872,#60873,#60874,#60875,#60876,#60877,#60878,#60879,
#60880,#60881,#60882,#60883,#60884,#60885,#60886,#60887,#60888,#60889,#60890,
#60891,#60892,#60893,#60894,#60895,#60896,#60897,#60898,#60899,#60900,#60901,
#60902,#60903,#60904,#60905,#60906,#60907,#60908,#60909),.UNSPECIFIED.,
 .F.,.F.,(4,2,2,2,2,2,2,2,2,2,2,2,2,2,2,2,2,2,2,2,2,2,2,2,2,2,2,2,2,2,2,
2,2,2,2,2,2,2,2,2,2,2,2,2,4),(1.61252832008002,1.66371044490681,3.32742088981362,
4.99113133472043,6.65484177962724,7.48669700208064,8.31855222453405,9.15040744698745,
9.98226266944086,10.3981902806676,10.8141178918943,11.230045503121,11.6459731143477,
12.0619007255744,12.4778283368011,12.6857921424144,12.8937559480278,13.1017197536411,
13.3096835592545,13.4995174511513,13.5944343970998,13.6893513430482,13.7842682889966,
13.8317267619709,13.8791852349451,13.9266437079193,13.9741021808935,13.9978314173806,
14.0215606538677,14.0452898903548,14.0571545085984,14.0690191268419,14.0808983984921,
14.0927776701422,14.0987173059673,14.1046569417923,14.1076267597049,14.1105965776174,
14.1135663955299,14.1150513044862,14.1165362134425,14.1172999498782,14.1180636863139,
14.1188274227496,14.1192092909675),.UNSPECIFIED.) ;
#539=B_SPLINE_CURVE_WITH_KNOTS('',3,(#60914,#60915,#60916,#60917,#60918,
#60919,#60920,#60921,#60922,#60923,#60924,#60925,#60926,#60927,#60928,#60929,
#60930,#60931,#60932,#60933,#60934,#60935,#60936,#60937,#60938,#60939,#60940,
#60941,#60942,#60943,#60944,#60945,#60946,#60947,#60948,#60949,#60950,#60951,
#60952,#60953,#60954,#60955,#60956,#60957,#60958,#60959,#60960,#60961,#60962,
#60963,#60964,#60965,#60966,#60967,#60968,#60969,#60970,#60971,#60972,#60973,
#60974,#60975,#60976,#60977,#60978,#60979,#60980,#60981,#60982,#60983,#60984,
#60985,#60986,#60987,#60988,#60989,#60990,#60991,#60992,#60993,#60994,#60995,
#60996,#60997,#60998,#60999,#61000,#61001),.UNSPECIFIED.,.F.,.F.,(4,2,2,
2,2,2,2,2,2,2,2,2,2,2,2,2,2,2,2,2,2,2,2,2,2,2,2,2,2,2,2,2,2,2,2,2,2,2,2,
2,2,2,2,4),(14.1663480270654,14.1667310037945,14.1674969572525,14.1682629107106,
14.1690288641686,14.1705181505994,14.1720074370301,14.1749860098916,14.1779645827531,
14.1809431556146,14.1869003013375,14.1928574470605,14.2047717385064,14.2166860299524,
14.2285859450541,14.2404858601559,14.2642856903595,14.2880855205631,14.3118853507666,
14.3594850111738,14.4070846715809,14.4546843319881,14.5022839923952,14.5974833132095,
14.6926826340238,14.787881954838,14.9782805964666,15.1869236817316,15.3955667669967,
15.6042098522617,15.8128529375267,16.2301391080568,16.6474252785868,17.0647114491168,
17.4819976196469,17.8992837901769,18.316569960707,19.1511423017671,19.9857146428272,
20.8202869838873,21.6548593249474,23.3240040070676,24.9931486891877,26.6718839962123),
 .UNSPECIFIED.) ;
#540=B_SPLINE_CURVE_WITH_KNOTS('',3,(#61002,#61003,#61004,#61005,#61006,
#61007,#61008,#61009,#61010,#61011,#61012,#61013,#61014,#61015,#61016,#61017,
#61018,#61019,#61020,#61021,#61022,#61023,#61024,#61025,#61026,#61027,#61028,
#61029,#61030,#61031,#61032,#61033,#61034,#61035,#61036,#61037,#61038,#61039,
#61040,#61041,#61042,#61043,#61044,#61045,#61046,#61047,#61048,#61049,#61050,
#61051,#61052,#61053,#61054,#61055,#61056,#61057,#61058,#61059,#61060,#61061,
#61062,#61063,#61064,#61065,#61066,#61067,#61068,#61069,#61070,#61071,#61072,
#61073,#61074,#61075,#61076,#61077,#61078,#61079,#61080,#61081,#61082,#61083,
#61084,#61085,#61086,#61087,#61088,#61089,#61090,#61091),.UNSPECIFIED.,
 .F.,.F.,(4,2,2,2,2,2,2,2,2,2,2,2,2,2,2,2,2,2,2,2,2,2,2,2,2,2,2,2,2,2,2,
2,2,2,2,2,2,2,2,2,2,2,2,2,4),(1.65955405721383,1.66914468202407,3.33828936404814,
5.0074340460722,6.67657872809627,7.5111510691083,8.34572341012034,9.18029575113237,
10.0148680921444,10.4321542626504,10.8494404331564,11.2667266036625,11.6840127741685,
12.1012989446745,12.5185851151805,12.7272282004335,12.9358712856865,13.1445143709395,
13.3531574561925,13.5435560981363,13.6387554191082,13.7339547400801,13.829154061052,
13.8767537215379,13.9243533820239,13.9719530425098,14.0195527029958,14.0433525332387,
14.0671523634817,14.0909521937247,14.1028521088462,14.1147520239677,14.1266663162782,
14.1385806085888,14.1445377547441,14.1504949008994,14.1534734739771,14.1564520470547,
14.1594306201324,14.1609199066712,14.16240919321,14.1631751463293,14.1639410994486,
14.1647070525679,14.1650900291276),.UNSPECIFIED.) ;
#541=B_SPLINE_CURVE_WITH_KNOTS('',3,(#61096,#61097,#61098,#61099,#61100,
#61101,#61102,#61103,#61104,#61105,#61106,#61107,#61108,#61109,#61110,#61111,
#61112,#61113,#61114,#61115,#61116,#61117,#61118,#61119,#61120,#61121,#61122,
#61123,#61124,#61125,#61126,#61127,#61128,#61129,#61130,#61131,#61132,#61133,
#61134,#61135,#61136,#61137,#61138,#61139,#61140,#61141,#61142,#61143,#61144,
#61145,#61146,#61147,#61148,#61149,#61150,#61151,#61152,#61153,#61154,#61155,
#61156,#61157,#61158,#61159,#61160,#61161,#61162,#61163,#61164,#61165,#61166,
#61167,#61168,#61169,#61170,#61171,#61172,#61173,#61174,#61175,#61176,#61177,
#61178,#61179,#61180,#61181,#61182,#61183,#61184),.UNSPECIFIED.,.F.,.F.,
(4,2,2,2,2,2,2,2,2,2,2,2,2,2,2,2,2,2,2,2,2,2,2,2,2,2,2,2,2,2,2,2,2,2,2,
2,2,2,2,2,2,2,2,1,4),(14.0669078689612,14.0672884427976,14.0680495904704,
14.0688107381431,14.0695718858159,14.0710516820229,14.0725314782298,14.0754910706438,
14.0784506630577,14.0814102554717,14.0873294402996,14.0932486251275,14.1050869947833,
14.1169253644391,14.1287487599683,14.1405721554975,14.164218946556,14.1878657376145,
14.2115125286729,14.2588061107899,14.3060996929068,14.3533932750237,14.4006868571406,
14.4952740213745,14.5898611856084,14.6844483498422,14.8736226783099,15.0807936570773,
15.2879646358446,15.4951356146119,15.7023065933792,16.1166485509138,16.5309905084485,
16.9453324659831,17.3596744235177,17.7740163810524,18.188358338587,19.0170422536563,
19.8457261687255,20.6744100837948,21.5030939988641,23.1604618290026,24.8178296591411,
26.4751974892797,26.5749735518018),.UNSPECIFIED.) ;
#542=B_SPLINE_CURVE_WITH_KNOTS('',3,(#61185,#61186,#61187,#61188,#61189,
#61190,#61191,#61192,#61193,#61194,#61195,#61196,#61197,#61198,#61199,#61200,
#61201,#61202,#61203,#61204,#61205,#61206,#61207,#61208,#61209,#61210,#61211,
#61212,#61213,#61214,#61215,#61216,#61217,#61218,#61219,#61220,#61221,#61222,
#61223,#61224,#61225,#61226,#61227,#61228,#61229,#61230,#61231,#61232,#61233,
#61234,#61235,#61236,#61237,#61238,#61239,#61240,#61241,#61242,#61243,#61244,
#61245,#61246,#61247,#61248,#61249,#61250,#61251,#61252,#61253,#61254,#61255,
#61256,#61257,#61258,#61259,#61260,#61261,#61262,#61263,#61264,#61265,#61266,
#61267,#61268,#61269,#61270,#61271,#61272,#61273,#61274),.UNSPECIFIED.,
 .F.,.F.,(4,2,2,2,2,2,2,2,2,2,2,2,2,2,2,2,2,2,2,2,2,2,2,2,2,2,2,2,2,2,2,
2,2,2,2,2,2,2,2,2,2,2,2,2,4),(1.5575917676117,1.65736782987813,3.31473565975626,
4.97210348963439,6.62947131951252,7.45815523445158,8.28683914939064,9.11552306432971,
9.94420697926877,10.3585489367383,10.7728908942078,11.1872328516774,11.6015748091469,
12.0159167666164,12.430258724086,12.6374297028207,12.8446006815555,13.0517716602903,
13.258942639025,13.4481169687325,13.5427041335862,13.63729129844,13.7318784632937,
13.7791720457206,13.8264656281474,13.8737592105743,13.9210527930012,13.9446995842146,
13.9683463754281,13.9919931666415,14.0038165622482,14.0156399578549,14.0274783271072,
14.0393166963594,14.0452358809855,14.0511550656117,14.0541146579247,14.0570742502378,
14.0600338425508,14.0615136387074,14.0629934348639,14.0637545820743,14.0645157292847,
14.0652768764951,14.0656574501003),.UNSPECIFIED.) ;
#543=B_SPLINE_CURVE_WITH_KNOTS('',3,(#61279,#61280,#61281,#61282,#61283,
#61284,#61285,#61286,#61287,#61288,#61289,#61290,#61291,#61292,#61293,#61294,
#61295,#61296,#61297,#61298,#61299,#61300,#61301,#61302,#61303,#61304,#61305,
#61306,#61307,#61308,#61309,#61310,#61311,#61312,#61313,#61314,#61315,#61316,
#61317,#61318,#61319,#61320,#61321,#61322,#61323,#61324,#61325,#61326,#61327,
#61328,#61329,#61330,#61331,#61332,#61333,#61334,#61335,#61336,#61337,#61338,
#61339,#61340,#61341,#61342,#61343,#61344,#61345,#61346,#61347,#61348,#61349,
#61350,#61351,#61352,#61353,#61354,#61355,#61356,#61357,#61358,#61359,#61360,
#61361,#61362,#61363,#61364,#61365,#61366,#61367,#61368),.UNSPECIFIED.,
 .F.,.F.,(4,2,2,2,2,2,2,2,2,2,2,2,2,2,2,2,2,2,2,2,2,2,2,2,2,2,2,2,2,2,2,
2,2,2,2,2,2,2,2,2,2,2,2,2,4),(14.0213425633806,14.0217220346764,14.0224809772678,
14.0232399198593,14.0239988624507,14.0254743060156,14.0269497495804,14.0299006367101,
14.0328515238398,14.0358024109695,14.041704185229,14.0476059594884,14.0594095080072,
14.0712130565261,14.0830013593196,14.0947896621131,14.1183662677001,14.1419428732872,
14.1655194788742,14.2126726900482,14.2598259012223,14.3069791123964,14.3541323235704,
14.4484387459185,14.5427451682666,14.6370515906147,14.8256644353109,15.0321609002033,
15.2386573650956,15.4451538299879,15.6516502948803,16.0646432246649,16.4776361544496,
16.8906290842342,17.3036220140189,17.7166149438035,18.1296078735882,18.9555937331575,
19.7815795927268,20.6075654522961,21.4335513118655,23.0855230310041,24.7374947501427,
26.3894664692814,26.5306282050422),.UNSPECIFIED.) ;
#544=B_SPLINE_CURVE_WITH_KNOTS('',3,(#61369,#61370,#61371,#61372,#61373,
#61374,#61375,#61376,#61377,#61378,#61379,#61380,#61381,#61382,#61383,#61384,
#61385,#61386,#61387,#61388,#61389,#61390,#61391,#61392,#61393,#61394,#61395,
#61396,#61397,#61398,#61399,#61400,#61401,#61402,#61403,#61404,#61405,#61406,
#61407,#61408,#61409,#61410,#61411,#61412,#61413,#61414,#61415,#61416,#61417,
#61418,#61419,#61420,#61421,#61422,#61423,#61424,#61425,#61426,#61427,#61428,
#61429,#61430,#61431,#61432,#61433,#61434,#61435,#61436,#61437,#61438,#61439,
#61440,#61441,#61442,#61443,#61444,#61445,#61446,#61447,#61448,#61449,#61450,
#61451,#61452,#61453,#61454,#61455,#61456,#61457,#61458),.UNSPECIFIED.,
 .F.,.F.,(4,2,2,2,2,2,2,2,2,2,2,2,2,2,2,2,2,2,2,2,2,2,2,2,2,2,2,2,2,2,2,
2,2,2,2,2,2,2,2,2,2,2,2,2,4),(1.51080998338537,1.65197171958198,3.30394343916396,
4.95591515874594,6.60788687832792,7.4338727381189,8.25985859790989,9.08584445770088,
9.91183031749187,10.3248232473874,10.7378161772829,11.1508091071784,11.5638020370739,
11.9767949669693,12.3897878968648,12.5962843618126,12.8027808267603,13.0092772917081,
13.2157737566558,13.4043865999103,13.4986930215375,13.5929994431648,13.687305864792,
13.7344590756056,13.7816122864192,13.8287654972328,13.8759187080464,13.8994953134532,
13.9230719188601,13.9466485242669,13.9584368269703,13.9702251296737,13.9820286784839,
13.9938322272942,13.9997340016993,14.0056357761044,14.008586663307,14.0115375505096,
14.0144884377121,14.0159638813134,14.0174393249147,14.0181982678899,14.0189572108651,
14.0197161538403,14.020095625328),.UNSPECIFIED.) ;
#545=B_SPLINE_CURVE_WITH_KNOTS('',3,(#61463,#61464,#61465,#61466,#61467,
#61468,#61469,#61470,#61471,#61472,#61473,#61474,#61475,#61476,#61477,#61478,
#61479,#61480,#61481,#61482,#61483,#61484,#61485,#61486,#61487,#61488,#61489,
#61490,#61491,#61492,#61493,#61494,#61495,#61496,#61497,#61498,#61499,#61500,
#61501,#61502,#61503,#61504,#61505,#61506,#61507,#61508,#61509,#61510,#61511,
#61512,#61513,#61514,#61515,#61516,#61517,#61518,#61519,#61520,#61521,#61522,
#61523,#61524,#61525,#61526,#61527,#61528,#61529,#61530,#61531,#61532,#61533,
#61534,#61535,#61536,#61537,#61538,#61539,#61540,#61541,#61542,#61543,#61544,
#61545,#61546,#61547,#61548,#61549,#61550),.UNSPECIFIED.,.F.,.F.,(4,2,2,
2,2,2,2,2,2,2,2,2,2,2,2,2,2,2,2,2,2,2,2,2,2,2,2,2,2,2,2,2,2,2,2,2,2,2,2,
2,2,2,2,4),(14.1547675290755,14.1551502263592,14.1559156209268,14.1566810154943,
14.1574464100618,14.158934591997,14.1604227739322,14.1633991378025,14.1663755016729,
14.1693518655432,14.1753045932839,14.1812573210246,14.193162776506,14.2050682319874,
14.2169592405274,14.2288502490674,14.2526322661473,14.2764142832273,14.3001963003072,
14.3477603344671,14.395324368627,14.4428884027869,14.4904524369468,14.5855805052665,
14.6807085735863,14.7758366419061,14.9660927785457,15.174564421742,15.3830360649383,
15.5915077081346,15.7999793513309,16.2169226377236,16.6338659241162,17.0508092105088,
17.4677524969015,17.8846957832941,18.3016390696867,19.135525642472,19.9694122152573,
20.8032987880425,21.6371853608278,23.3049585063983,24.9727316519689,26.6605889274289),
 .UNSPECIFIED.) ;
#546=B_SPLINE_CURVE_WITH_KNOTS('',3,(#61551,#61552,#61553,#61554,#61555,
#61556,#61557,#61558,#61559,#61560,#61561,#61562,#61563,#61564,#61565,#61566,
#61567,#61568,#61569,#61570,#61571,#61572,#61573,#61574,#61575,#61576,#61577,
#61578,#61579,#61580,#61581,#61582,#61583,#61584,#61585,#61586,#61587,#61588,
#61589,#61590,#61591,#61592,#61593,#61594,#61595,#61596,#61597,#61598,#61599,
#61600,#61601,#61602,#61603,#61604,#61605,#61606,#61607,#61608,#61609,#61610,
#61611,#61612,#61613,#61614,#61615,#61616,#61617,#61618,#61619,#61620,#61621,
#61622,#61623,#61624,#61625,#61626,#61627,#61628,#61629,#61630,#61631,#61632,
#61633,#61634,#61635,#61636,#61637,#61638,#61639,#61640),.UNSPECIFIED.,
 .F.,.F.,(4,2,2,2,2,2,2,2,2,2,2,2,2,2,2,2,2,2,2,2,2,2,2,2,2,2,2,2,2,2,2,
2,2,2,2,2,2,2,2,2,2,2,2,2,4),(1.64768901568821,1.66777314593728,3.33554629187456,
5.00331943781184,6.67109258374912,7.50497915671776,8.3388657296864,9.17275230265505,
10.0066388756237,10.423582162108,10.8405254485923,11.2574687350766,11.674412021561,
12.0913553080453,12.5082985945296,12.7167702377718,12.9252418810139,13.1337135242561,
13.3421851674982,13.5324413032841,13.627569371177,13.72269743907,13.8178255069629,
13.8653895409093,13.9129535748558,13.9605176088023,14.0080816427487,14.031863659722,
14.0556456766952,14.0794276936684,14.091318702155,14.1032097106417,14.1151151666865,
14.1270206227314,14.1329733507539,14.1389260787763,14.1419024427876,14.1448788067988,
14.14785517081,14.1493433528156,14.1508315348212,14.1515969290159,14.1523623232106,
14.1531277174053,14.1535104145027),.UNSPECIFIED.) ;
#547=B_SPLINE_CURVE_WITH_KNOTS('',3,(#61645,#61646,#61647,#61648,#61649,
#61650,#61651,#61652,#61653,#61654,#61655,#61656,#61657,#61658,#61659,#61660,
#61661,#61662,#61663,#61664,#61665,#61666,#61667,#61668,#61669,#61670,#61671,
#61672,#61673,#61674,#61675,#61676,#61677,#61678,#61679,#61680,#61681,#61682,
#61683,#61684,#61685,#61686,#61687,#61688,#61689,#61690,#61691,#61692,#61693,
#61694,#61695,#61696,#61697,#61698,#61699,#61700,#61701,#61702,#61703,#61704,
#61705,#61706,#61707,#61708,#61709,#61710,#61711,#61712,#61713,#61714,#61715,
#61716,#61717,#61718,#61719,#61720,#61721,#61722,#61723,#61724,#61725,#61726,
#61727,#61728,#61729,#61730,#61731,#61732),.UNSPECIFIED.,.F.,.F.,(4,2,2,
2,2,2,2,2,2,2,2,2,2,2,2,2,2,2,2,2,2,2,2,2,2,2,2,2,2,2,2,2,2,2,2,2,2,2,2,
2,2,2,2,4),(14.1455560202463,14.1459384946887,14.1467034435733,14.147468392458,
14.1482333413426,14.1497206445499,14.1512079477573,14.154182554172,14.1571571605867,
14.1601317670014,14.1660809798308,14.1720301926602,14.183928618319,14.1958270439778,
14.2077109670005,14.2195948900231,14.2433627360685,14.2671305821138,14.2908984281591,
14.3384341202498,14.3859698123404,14.4335055044311,14.4810411965218,14.5761125807031,
14.6711839648844,14.7662553490657,14.9563981174284,15.1647333909699,15.3730686645115,
15.581403938053,15.7897392115945,16.2064097586776,16.6230803057607,17.0397508528437,
17.4564213999268,17.8730919470099,18.2897624940929,19.1231035882591,19.9564446824252,
20.7897857765913,21.6231268707575,23.2898090590897,24.956491247422,26.6516061654756),
 .UNSPECIFIED.) ;
#548=B_SPLINE_CURVE_WITH_KNOTS('',3,(#61733,#61734,#61735,#61736,#61737,
#61738,#61739,#61740,#61741,#61742,#61743,#61744,#61745,#61746,#61747,#61748,
#61749,#61750,#61751,#61752,#61753,#61754,#61755,#61756,#61757,#61758,#61759,
#61760,#61761,#61762,#61763,#61764,#61765,#61766,#61767,#61768,#61769,#61770,
#61771,#61772,#61773,#61774,#61775,#61776,#61777,#61778,#61779,#61780,#61781,
#61782,#61783,#61784,#61785,#61786,#61787,#61788,#61789,#61790,#61791,#61792,
#61793,#61794,#61795,#61796,#61797,#61798,#61799,#61800,#61801,#61802,#61803,
#61804,#61805,#61806,#61807,#61808,#61809,#61810,#61811,#61812,#61813,#61814,
#61815,#61816,#61817,#61818,#61819,#61820,#61821,#61822),.UNSPECIFIED.,
 .F.,.F.,(4,2,2,2,2,2,2,2,2,2,2,2,2,2,2,2,2,2,2,2,2,2,2,2,2,2,2,2,2,2,2,
2,2,2,2,2,2,2,2,2,2,2,2,2,4),(1.63824945861164,1.66668218836848,3.33336437673695,
5.00004656510543,6.6667287534739,7.50006984765814,8.33341094184238,9.16675203602662,
10.0000931302109,10.416763677303,10.8334342243951,11.2501047714872,11.6667753185793,
12.0834458656714,12.5001164127636,12.7084516863096,12.9167869598557,13.1251222334017,
13.3334575069478,13.523600275367,13.6186716595767,13.7137430437863,13.8088144279959,
13.8563501201007,13.9038858122055,13.9514215043103,13.9989571964151,14.0227250424676,
14.04649288852,14.0702607345724,14.0821446575986,14.0940285806248,14.1059270062631,
14.1178254319013,14.1237746447205,14.1297238575396,14.1326984639492,14.1356730703588,
14.1386476767684,14.1401349799731,14.1416222831779,14.1423872317731,14.1431521803684,
14.1439171289636,14.1442996032612),.UNSPECIFIED.) ;
#549=B_SPLINE_CURVE_WITH_KNOTS('',3,(#61827,#61828,#61829,#61830,#61831,
#61832,#61833,#61834,#61835,#61836,#61837,#61838,#61839,#61840,#61841,#61842,
#61843,#61844,#61845,#61846,#61847,#61848,#61849,#61850,#61851,#61852,#61853,
#61854,#61855,#61856,#61857,#61858,#61859,#61860,#61861,#61862,#61863,#61864,
#61865,#61866,#61867,#61868,#61869,#61870,#61871,#61872,#61873,#61874,#61875,
#61876,#61877,#61878,#61879,#61880,#61881,#61882,#61883,#61884,#61885,#61886,
#61887,#61888,#61889,#61890,#61891,#61892,#61893,#61894,#61895,#61896,#61897,
#61898,#61899,#61900,#61901,#61902,#61903,#61904,#61905,#61906,#61907,#61908,
#61909,#61910,#61911,#61912,#61913,#61914,#61915,#61916),.UNSPECIFIED.,
 .F.,.F.,(4,2,2,2,2,2,2,2,2,2,2,2,2,2,2,2,2,2,2,2,2,2,2,2,2,2,2,2,2,2,2,
2,2,2,2,2,2,2,2,2,2,2,2,2,4),(13.9958308278975,13.9962096819733,13.9969673901248,
13.9977250982764,13.9984828064279,13.9999558119132,14.0014288173985,14.0043748283691,
14.0073208393397,14.0102668503103,14.0161588722515,14.0220508941927,14.0338349380751,
14.0456189819575,14.0573876282138,14.0691562744701,14.0926935669827,14.1162308594952,
14.1397681520078,14.1868427370329,14.233917322058,14.2809919070831,14.3280664921082,
14.4222156621585,14.5163648322087,14.6105140022589,14.7988123423594,15.0049311599118,
15.2110499774642,15.4171687950166,15.6232876125691,16.0355252476739,16.4477628827787,
16.8600005178836,17.2722381529884,17.6844757880933,18.0967134231981,18.9211886934078,
19.7456639636175,20.5701392338272,21.3946145040369,23.0435650444562,24.6925155848756,
26.341466125295,26.5058166411774),.UNSPECIFIED.) ;
#550=B_SPLINE_CURVE_WITH_KNOTS('',3,(#61917,#61918,#61919,#61920,#61921,
#61922,#61923,#61924,#61925,#61926,#61927,#61928,#61929,#61930,#61931,#61932,
#61933,#61934,#61935,#61936,#61937,#61938,#61939,#61940,#61941,#61942,#61943,
#61944,#61945,#61946,#61947,#61948,#61949,#61950,#61951,#61952,#61953,#61954,
#61955,#61956,#61957,#61958,#61959,#61960,#61961,#61962,#61963,#61964,#61965,
#61966,#61967,#61968,#61969,#61970,#61971,#61972,#61973,#61974,#61975,#61976,
#61977,#61978,#61979,#61980,#61981,#61982,#61983,#61984,#61985,#61986,#61987,
#61988,#61989,#61990,#61991,#61992,#61993,#61994,#61995,#61996,#61997,#61998,
#61999,#62000,#62001,#62002,#62003,#62004,#62005,#62006),.UNSPECIFIED.,
 .F.,.F.,(4,2,2,2,2,2,2,2,2,2,2,2,2,2,2,2,2,2,2,2,2,2,2,2,2,2,2,2,2,2,2,
2,2,2,2,2,2,2,2,2,2,2,2,2,4),(1.48460002454131,1.64895054067987,3.29790108135973,
4.9468516220396,6.59580216271946,7.42027743305939,8.24475270339932,9.06922797373926,
9.89370324407919,10.3059408792492,10.7181785144191,11.1304161495891,11.5426537847591,
11.954891419929,12.367129055099,12.573247872684,12.779366690269,12.9854855078539,
13.1916043254389,13.3799026654271,13.4740518354212,13.5682010054153,13.6623501754094,
13.7094247604064,13.7564993454035,13.8035739304005,13.8506485153976,13.8741858078961,
13.8977231003946,13.9212603928931,13.9330290391424,13.9447976853916,13.9565817297195,
13.9683657740474,13.9742577962114,13.9801498183753,13.9830958294573,13.9860418405393,
13.9889878516212,13.9904608571622,13.9919338627032,13.9926915708602,13.9934492790172,
13.9942069871742,13.9945858412527),.UNSPECIFIED.) ;
#551=B_SPLINE_CURVE_WITH_KNOTS('',3,(#62011,#62012,#62013,#62014,#62015,
#62016,#62017,#62018,#62019,#62020,#62021,#62022,#62023,#62024,#62025,#62026,
#62027,#62028,#62029,#62030,#62031,#62032,#62033,#62034,#62035,#62036,#62037,
#62038,#62039,#62040,#62041,#62042,#62043,#62044,#62045,#62046,#62047,#62048,
#62049,#62050,#62051,#62052,#62053,#62054,#62055,#62056,#62057,#62058,#62059,
#62060,#62061,#62062,#62063,#62064,#62065,#62066,#62067,#62068,#62069,#62070,
#62071,#62072,#62073,#62074,#62075,#62076,#62077,#62078,#62079,#62080,#62081,
#62082,#62083,#62084,#62085,#62086,#62087,#62088,#62089,#62090,#62091,#62092,
#62093,#62094,#62095,#62096,#62097,#62098,#62099),.UNSPECIFIED.,.F.,.F.,
(4,2,2,2,2,2,2,2,2,2,2,2,2,2,2,2,2,2,2,2,2,2,2,2,2,2,2,2,2,2,2,2,2,2,2,
2,2,2,2,2,2,2,2,1,4),(14.0868029211861,14.0871839758337,14.0879460851289,
14.0887081944242,14.0894703037194,14.0909519997192,14.092433695719,14.0953970877186,
14.0983604797182,14.1013238717178,14.107250655717,14.1131774397162,14.1250310077145,
14.1368845757129,14.1487232877793,14.1605619998456,14.1842394239783,14.2079168481109,
14.2315942722436,14.2789491205089,14.3263039687743,14.3736588170396,14.421013665305,
14.5157233618356,14.6104330583663,14.705142754897,14.8945621479584,15.1020276442232,
15.309493140488,15.5169586367529,15.7244241330177,16.1393551255474,16.5542861180771,
16.9692171106068,17.3841481031365,17.7990790956662,18.2140100881959,19.0438720732552,
19.8737340583146,20.703596043374,21.5334580284334,23.1931819985521,24.8529059686708,
26.5126299387896,26.594348067054),.UNSPECIFIED.) ;
#552=B_SPLINE_CURVE_WITH_KNOTS('',3,(#62100,#62101,#62102,#62103,#62104,
#62105,#62106,#62107,#62108,#62109,#62110,#62111,#62112,#62113,#62114,#62115,
#62116,#62117,#62118,#62119,#62120,#62121,#62122,#62123,#62124,#62125,#62126,
#62127,#62128,#62129,#62130,#62131,#62132,#62133,#62134,#62135,#62136,#62137,
#62138,#62139,#62140,#62141,#62142,#62143,#62144,#62145,#62146,#62147,#62148,
#62149,#62150,#62151,#62152,#62153,#62154,#62155,#62156,#62157,#62158,#62159,
#62160,#62161,#62162,#62163,#62164,#62165,#62166,#62167,#62168,#62169,#62170,
#62171,#62172,#62173,#62174,#62175,#62176,#62177,#62178,#62179,#62180,#62181,
#62182,#62183,#62184,#62185,#62186,#62187,#62188,#62189),.UNSPECIFIED.,
 .F.,.F.,(4,2,2,2,2,2,2,2,2,2,2,2,2,2,2,2,2,2,2,2,2,2,2,2,2,2,2,2,2,2,2,
2,2,2,2,2,2,2,2,2,2,2,2,2,4),(1.57800584185246,1.65972397001552,3.31944794003104,
4.97917191004656,6.63889588006208,7.46875786506984,8.2986198500776,9.12848183508536,
9.95834382009312,10.373274812597,10.7882058051009,11.2031367976048,11.6180677901086,
12.0329987826125,12.4479297751164,12.6553952713683,12.8628607676203,13.0703262638722,
13.2777917601242,13.4672111537424,13.5619208505516,13.6566305473607,13.7513402441698,
13.7986950925744,13.846049940979,13.8934047893835,13.9407596377881,13.9644370619904,
13.9881144861927,14.0117919103949,14.0236306224961,14.0354693345972,14.0473229019233,
14.0591764692495,14.0651032529125,14.0710300365756,14.0739934284071,14.0769568202386,
14.0799202120702,14.0814019079859,14.0828836039017,14.0836457139642,14.0844078240268,
14.0851699340893,14.0855509891206),.UNSPECIFIED.) ;
#553=B_SPLINE_CURVE_WITH_KNOTS('',3,(#62194,#62195,#62196,#62197,#62198,
#62199,#62200,#62201,#62202,#62203,#62204,#62205,#62206,#62207,#62208,#62209,
#62210,#62211,#62212,#62213,#62214,#62215,#62216,#62217,#62218,#62219,#62220,
#62221,#62222,#62223,#62224,#62225,#62226,#62227,#62228,#62229,#62230,#62231,
#62232,#62233,#62234,#62235,#62236,#62237,#62238,#62239,#62240,#62241,#62242,
#62243,#62244,#62245,#62246,#62247,#62248,#62249,#62250,#62251,#62252,#62253,
#62254,#62255,#62256,#62257,#62258,#62259,#62260,#62261,#62262,#62263,#62264,
#62265,#62266,#62267,#62268,#62269,#62270,#62271,#62272,#62273,#62274,#62275,
#62276,#62277,#62278,#62279,#62280,#62281),.UNSPECIFIED.,.F.,.F.,(4,2,2,
2,2,2,2,2,2,2,2,2,2,2,2,2,2,2,2,2,2,2,2,2,2,2,2,2,2,2,2,2,2,2,2,2,2,2,2,
2,2,2,2,4),(14.1686729957178,14.1690560284224,14.1698220938314,14.1705881592404,
14.1713542246494,14.1728437329402,14.1743332412309,14.1773122578124,14.1802912743938,
14.1832702909753,14.1892283241382,14.1951863573012,14.2071024236271,14.2190184899529,
14.2309201930728,14.2428218961926,14.2666253024322,14.2904287086718,14.3142321149114,
14.3618389273906,14.4094457398698,14.457052552349,14.5046593648282,14.5998729897866,
14.695086614745,14.7903002397034,14.9807274896203,15.1894049946999,15.3980824997795,
15.6067600048591,15.8154375099388,16.232792520098,16.6501475302573,17.0675025404165,
17.4848575505757,17.902212560735,18.3195675708942,19.1542775912127,19.9889876115312,
20.8236976318497,21.6584076521682,23.3278276928052,24.9972477334421,26.6741519500694),
 .UNSPECIFIED.) ;
#554=B_SPLINE_CURVE_WITH_KNOTS('',3,(#62282,#62283,#62284,#62285,#62286,
#62287,#62288,#62289,#62290,#62291,#62292,#62293,#62294,#62295,#62296,#62297,
#62298,#62299,#62300,#62301,#62302,#62303,#62304,#62305,#62306,#62307,#62308,
#62309,#62310,#62311,#62312,#62313,#62314,#62315,#62316,#62317,#62318,#62319,
#62320,#62321,#62322,#62323,#62324,#62325,#62326,#62327,#62328,#62329,#62330,
#62331,#62332,#62333,#62334,#62335,#62336,#62337,#62338,#62339,#62340,#62341,
#62342,#62343,#62344,#62345,#62346,#62347,#62348,#62349,#62350,#62351,#62352,
#62353,#62354,#62355,#62356,#62357,#62358,#62359,#62360,#62361,#62362,#62363,
#62364,#62365,#62366,#62367,#62368,#62369,#62370,#62371),.UNSPECIFIED.,
 .F.,.F.,(4,2,2,2,2,2,2,2,2,2,2,2,2,2,2,2,2,2,2,2,2,2,2,2,2,2,2,2,2,2,2,
2,2,2,2,2,2,2,2,2,2,2,2,2,4),(1.66193586464491,1.66942004054979,3.33884008109958,
5.00826012164937,6.67768016219916,7.51239018247405,8.34710020274895,9.18181022302385,
10.0165202432987,10.4338752534362,10.8512302635736,11.2685852737111,11.6859402838485,
12.103295293986,12.5206503041234,12.7293278091921,12.9380053142609,13.1466828193296,
13.3553603243983,13.545787573842,13.6410011985639,13.7362148232857,13.8314284480076,
13.8790352603685,13.9266420727294,13.9742488850903,14.0218556974513,14.0456591036317,
14.0694625098122,14.0932659159926,14.1051676190829,14.1170693221731,14.1289853886477,
14.1409014551223,14.1468594883595,14.1528175215968,14.1557965382155,14.1587755548341,
14.1617545714527,14.1632440797621,14.1647335880714,14.1654996538429,14.1662657196144,
14.1670317853859,14.1674148182716),.UNSPECIFIED.) ;
#555=B_SPLINE_CURVE_WITH_KNOTS('',3,(#62376,#62377,#62378,#62379,#62380,
#62381,#62382,#62383,#62384,#62385,#62386,#62387,#62388,#62389,#62390,#62391,
#62392,#62393,#62394,#62395,#62396,#62397,#62398,#62399,#62400,#62401,#62402,
#62403,#62404,#62405,#62406,#62407,#62408,#62409,#62410,#62411,#62412,#62413,
#62414,#62415,#62416,#62417,#62418,#62419,#62420,#62421,#62422,#62423,#62424,
#62425,#62426,#62427,#62428,#62429,#62430,#62431,#62432,#62433,#62434,#62435,
#62436,#62437,#62438,#62439,#62440,#62441,#62442,#62443,#62444,#62445,#62446,
#62447,#62448,#62449,#62450,#62451,#62452,#62453,#62454,#62455,#62456,#62457,
#62458,#62459,#62460,#62461,#62462,#62463,#62464),.UNSPECIFIED.,.F.,.F.,
(4,2,2,2,2,2,2,2,2,2,2,2,2,2,2,2,2,2,2,2,2,2,2,2,2,2,2,2,2,2,2,2,2,2,2,
2,2,2,2,2,2,2,2,1,4),(14.1046764400768,14.1050579266305,14.1058208997379,
14.1065838728453,14.1073468459527,14.1088302481455,14.1103136503384,14.113280454724,
14.1162472591097,14.1192140634954,14.1251476722667,14.1310812810381,14.1429484985808,
14.1548157161235,14.1666681853681,14.1785206546127,14.202225593102,14.2259305315912,
14.2496354700804,14.2970453470589,14.3444552240374,14.3918651010159,14.4392749779944,
14.5340947319514,14.6289144859084,14.7237342398654,14.9133737477793,15.1211038389457,
15.3288339301121,15.5365640212784,15.7442941124448,16.1597542947775,16.5752144771102,
16.990674659443,17.4061348417757,17.8215950241084,18.2370552064411,19.0679755711066,
19.8988959357721,20.7298163004375,21.560736665103,23.2225773944339,24.8844181237648,
26.5462588530957,26.6117601472044),.UNSPECIFIED.) ;
#556=B_SPLINE_CURVE_WITH_KNOTS('',3,(#62465,#62466,#62467,#62468,#62469,
#62470,#62471,#62472,#62473,#62474,#62475,#62476,#62477,#62478,#62479,#62480,
#62481,#62482,#62483,#62484,#62485,#62486,#62487,#62488,#62489,#62490,#62491,
#62492,#62493,#62494,#62495,#62496,#62497,#62498,#62499,#62500,#62501,#62502,
#62503,#62504,#62505,#62506,#62507,#62508,#62509,#62510,#62511,#62512,#62513,
#62514,#62515,#62516,#62517,#62518,#62519,#62520,#62521,#62522,#62523,#62524,
#62525,#62526,#62527,#62528,#62529,#62530,#62531,#62532,#62533,#62534,#62535,
#62536,#62537,#62538,#62539,#62540,#62541,#62542,#62543,#62544,#62545,#62546,
#62547,#62548,#62549,#62550,#62551,#62552,#62553,#62554),.UNSPECIFIED.,
 .F.,.F.,(4,2,2,2,2,2,2,2,2,2,2,2,2,2,2,2,2,2,2,2,2,2,2,2,2,2,2,2,2,2,2,
2,2,2,2,2,2,2,2,2,2,2,2,2,4),(1.59633943522304,1.66184072937422,3.32368145874844,
4.98552218812266,6.64736291749688,7.47828328218399,8.3092036468711,9.14012401155821,
9.97104437624532,10.3865045585889,10.8019647409324,11.217424923276,11.6328851056195,
12.0483452879631,12.4638054703066,12.6715355614784,12.8792656526502,13.086995743822,
13.2947258349938,13.4843653425812,13.5791850963749,13.6740048501686,13.7688246039623,
13.8162344808592,13.8636443577561,13.9110542346529,13.9584641115498,13.9821690499982,
14.0058739884466,14.0295789268951,14.0414313961193,14.0532838653435,14.0651510830035,
14.0770183006634,14.0829519094934,14.0888855183234,14.0918523227384,14.0948191271534,
14.0977859315684,14.0992693337759,14.1007527359834,14.1015157096051,14.1022786832268,
14.1030416568486,14.1034231436594),.UNSPECIFIED.) ;
#557=B_SPLINE_CURVE_WITH_KNOTS('',3,(#62559,#62560,#62561,#62562,#62563,
#62564,#62565,#62566,#62567,#62568,#62569,#62570,#62571,#62572,#62573,#62574,
#62575,#62576,#62577,#62578,#62579,#62580,#62581,#62582,#62583,#62584,#62585,
#62586,#62587,#62588,#62589,#62590,#62591,#62592,#62593,#62594,#62595,#62596,
#62597,#62598,#62599,#62600,#62601,#62602,#62603,#62604,#62605,#62606,#62607,
#62608,#62609,#62610,#62611,#62612,#62613,#62614,#62615,#62616,#62617,#62618,
#62619,#62620,#62621,#62622,#62623,#62624,#62625,#62626,#62627,#62628,#62629,
#62630,#62631,#62632,#62633,#62634,#62635,#62636,#62637,#62638,#62639,#62640,
#62641,#62642,#62643,#62644,#62645,#62646,#62647,#62648),.UNSPECIFIED.,
 .F.,.F.,(4,2,2,2,2,2,2,2,2,2,2,2,2,2,2,2,2,2,2,2,2,2,2,2,2,2,2,2,2,2,2,
2,2,2,2,2,2,2,2,2,2,2,2,2,4),(13.9686134586717,13.9689916543654,13.9697480457528,
13.9705044371402,13.9712608285275,13.9727312318299,13.9742016351324,13.9771424417372,
13.980083248342,13.9830240549468,13.9889056681565,13.9947872813661,14.0065505077854,
14.0183137342047,14.0300614031915,14.0418090721782,14.0653044101518,14.0887997481254,
14.112295086099,14.1592857620462,14.2062764379934,14.2532671139406,14.3002577898878,
14.3942391417821,14.4882204936765,14.5822018455709,14.7701645493596,14.9758804783754,
15.1815964073912,15.3873123364069,15.5930282654227,16.0044601234543,16.4158919814858,
16.8273238395174,17.2387556975489,17.6501875555805,18.061619413612,18.8844831296751,
19.7073468457382,20.5302105618013,21.3530742778644,22.9988017099906,24.6445291421168,
26.290256574243,26.4793600109925),.UNSPECIFIED.) ;
#558=B_SPLINE_CURVE_WITH_KNOTS('',3,(#62649,#62650,#62651,#62652,#62653,
#62654,#62655,#62656,#62657,#62658,#62659,#62660,#62661,#62662,#62663,#62664,
#62665,#62666,#62667,#62668,#62669,#62670,#62671,#62672,#62673,#62674,#62675,
#62676,#62677,#62678,#62679,#62680,#62681,#62682,#62683,#62684,#62685,#62686,
#62687,#62688,#62689,#62690,#62691,#62692,#62693,#62694,#62695,#62696,#62697,
#62698,#62699,#62700,#62701,#62702,#62703,#62704,#62705,#62706,#62707,#62708,
#62709,#62710,#62711,#62712,#62713,#62714,#62715,#62716,#62717,#62718,#62719,
#62720,#62721,#62722,#62723,#62724,#62725,#62726,#62727,#62728,#62729,#62730,
#62731,#62732,#62733,#62734,#62735,#62736,#62737,#62738),.UNSPECIFIED.,
 .F.,.F.,(4,2,2,2,2,2,2,2,2,2,2,2,2,2,2,2,2,2,2,2,2,2,2,2,2,2,2,2,2,2,2,
2,2,2,2,2,2,2,2,2,2,2,2,2,4),(1.45662399537187,1.64572743182393,3.29145486364787,
4.9371822954718,6.58290972729574,7.4057734432077,8.22863715911967,9.05150087503164,
9.8743645909436,10.2857964488996,10.6972283068556,11.1086601648116,11.5200920227675,
11.9315238807235,12.3429557386795,12.5486716676575,12.7543875966355,12.9601035256135,
13.1658194545915,13.3537821585869,13.4477635105846,13.5417448625823,13.6357262145801,
13.6827168905789,13.7297075665778,13.7766982425766,13.8236889185755,13.8471842565749,
13.8706795945744,13.8941749325738,13.9059226015735,13.9176702705732,13.9294334979076,
13.941196725242,13.9470783389092,13.9529599525763,13.9559007594099,13.9588415662435,
13.9617823730771,13.9632527764939,13.9647231799107,13.9654795712734,13.9662359626361,
13.9669923539988,13.9673705496801),.UNSPECIFIED.) ;
#559=B_SPLINE_CURVE_WITH_KNOTS('',3,(#62743,#62744,#62745,#62746,#62747,
#62748,#62749,#62750,#62751,#62752,#62753,#62754,#62755,#62756,#62757,#62758,
#62759,#62760,#62761,#62762,#62763,#62764,#62765,#62766,#62767,#62768,#62769,
#62770,#62771,#62772,#62773,#62774,#62775,#62776,#62777,#62778,#62779,#62780,
#62781,#62782,#62783,#62784,#62785,#62786,#62787,#62788,#62789,#62790,#62791,
#62792,#62793,#62794,#62795,#62796,#62797,#62798,#62799,#62800,#62801,#62802,
#62803,#62804,#62805,#62806,#62807,#62808,#62809,#62810,#62811,#62812,#62813,
#62814,#62815,#62816,#62817,#62818,#62819,#62820,#62821,#62822,#62823,#62824,
#62825,#62826,#62827,#62828,#62829,#62830),.UNSPECIFIED.,.F.,.F.,(4,2,2,
2,2,2,2,2,2,2,2,2,2,2,2,2,2,2,2,2,2,2,2,2,2,2,2,2,2,2,2,2,2,2,2,2,2,2,2,
2,2,2,2,4),(14.1341071619772,14.1344893601054,14.1352537563619,14.1360181526184,
14.1367825488748,14.1382687596458,14.1397549704169,14.1427273919589,14.1456998135009,
14.148672235043,14.1546170781271,14.1605619212112,14.1724516073793,14.1843412935475,
14.1962164091354,14.2080915247234,14.2318417558993,14.2555919870753,14.2793422182512,
14.326842680603,14.3743431429549,14.4218436053067,14.4693440676586,14.5643449923623,
14.659345917066,14.7543468417697,14.944348691177,15.1525144738915,15.3606802566059,
15.5688460393203,15.7770118220347,16.1933433874636,16.6096749528924,17.0260065183213,
17.4423380837501,17.858669649179,18.2750012146078,19.1076643454655,19.9403274763232,
20.7729906071809,21.6056537380386,23.2709799997539,24.9363062614693,26.640443728447),
 .UNSPECIFIED.) ;
#560=B_SPLINE_CURVE_WITH_KNOTS('',3,(#62831,#62832,#62833,#62834,#62835,
#62836,#62837,#62838,#62839,#62840,#62841,#62842,#62843,#62844,#62845,#62846,
#62847,#62848,#62849,#62850,#62851,#62852,#62853,#62854,#62855,#62856,#62857,
#62858,#62859,#62860,#62861,#62862,#62863,#62864,#62865,#62866,#62867,#62868,
#62869,#62870,#62871,#62872,#62873,#62874,#62875,#62876,#62877,#62878,#62879,
#62880,#62881,#62882,#62883,#62884,#62885,#62886,#62887,#62888,#62889,#62890,
#62891,#62892,#62893,#62894,#62895,#62896,#62897,#62898,#62899,#62900,#62901,
#62902,#62903,#62904,#62905,#62906,#62907,#62908,#62909,#62910,#62911,#62912,
#62913,#62914,#62915,#62916,#62917,#62918,#62919,#62920),.UNSPECIFIED.,
 .F.,.F.,(4,2,2,2,2,2,2,2,2,2,2,2,2,2,2,2,2,2,2,2,2,2,2,2,2,2,2,2,2,2,2,
2,2,2,2,2,2,2,2,2,2,2,2,2,4),(1.62651505645996,1.66532626207607,3.33065252415214,
4.9959787862282,6.66130504830427,7.4939681793423,8.32663131038034,9.15929444141837,
9.99195757245641,10.4082891379754,10.8246207034944,11.2409522690135,11.6572838345325,
12.0736154000515,12.4899469655705,12.69811274833,12.9062785310895,13.114444313849,
13.3226100966085,13.5126119449433,13.6076128691107,13.702613793278,13.7976147174454,
13.8451151795291,13.8926156416128,13.9401161036965,13.9876165657801,14.011366796822,
14.0351170278638,14.0588672589057,14.0707423744266,14.0826174899475,14.0945071767465,
14.1063968635454,14.1123417069449,14.1182865503443,14.1212589720441,14.1242313937438,
14.1272038154435,14.1286900262934,14.1301762371433,14.1309406333205,14.1317050294977,
14.1324694256748,14.1328516237634),.UNSPECIFIED.) ;
#561=B_SPLINE_CURVE_WITH_KNOTS('',3,(#62925,#62926,#62927,#62928,#62929,
#62930,#62931,#62932,#62933,#62934,#62935,#62936,#62937,#62938,#62939,#62940,
#62941,#62942,#62943,#62944,#62945,#62946,#62947,#62948,#62949,#62950,#62951,
#62952,#62953,#62954,#62955,#62956,#62957,#62958,#62959,#62960,#62961,#62962,
#62963,#62964,#62965,#62966,#62967,#62968,#62969,#62970,#62971,#62972,#62973,
#62974,#62975,#62976,#62977,#62978,#62979,#62980,#62981,#62982,#62983,#62984,
#62985,#62986,#62987,#62988,#62989,#62990,#62991,#62992,#62993,#62994,#62995,
#62996,#62997,#62998,#62999,#63000,#63001,#63002,#63003,#63004,#63005,#63006,
#63007,#63008,#63009,#63010,#63011,#63012),.UNSPECIFIED.,.F.,.F.,(4,2,2,
2,2,2,2,2,2,2,2,2,2,2,2,2,2,2,2,2,2,2,2,2,2,2,2,2,2,2,2,2,2,2,2,2,2,2,2,
2,2,2,2,4),(14.1617069747248,14.1620898390495,14.1628555676989,14.1636212963483,
14.1643870249977,14.165875868894,14.1673647127904,14.1703424005831,14.1733200883758,
14.1762977761685,14.1822531517539,14.1882085273393,14.2001192785101,14.2120300296809,
14.2239263755092,14.2358227213376,14.2596154129943,14.2834081046509,14.3072007963076,
14.354786179621,14.4023715629344,14.4499569462477,14.4975423295611,14.5927130961878,
14.6878838628146,14.7830546294413,14.9733961626948,15.1819705398313,15.3905449169678,
15.5991192941043,15.8076936712408,16.2248424255138,16.6419911797868,17.0591399340598,
17.4762886883328,17.8934374426059,18.3105861968789,19.1448837054249,19.9791812139709,
20.813478722517,21.647776231063,23.3163712481551,24.9849662652471,26.6673570419534),
 .UNSPECIFIED.) ;
#562=B_SPLINE_CURVE_WITH_KNOTS('',3,(#63013,#63014,#63015,#63016,#63017,
#63018,#63019,#63020,#63021,#63022,#63023,#63024,#63025,#63026,#63027,#63028,
#63029,#63030,#63031,#63032,#63033,#63034,#63035,#63036,#63037,#63038,#63039,
#63040,#63041,#63042,#63043,#63044,#63045,#63046,#63047,#63048,#63049,#63050,
#63051,#63052,#63053,#63054,#63055,#63056,#63057,#63058,#63059,#63060,#63061,
#63062,#63063,#63064,#63065,#63066,#63067,#63068,#63069,#63070,#63071,#63072,
#63073,#63074,#63075,#63076,#63077,#63078,#63079,#63080,#63081,#63082,#63083,
#63084,#63085,#63086,#63087,#63088,#63089,#63090,#63091,#63092,#63093,#63094,
#63095,#63096,#63097,#63098,#63099,#63100,#63101,#63102),.UNSPECIFIED.,
 .F.,.F.,(4,2,2,2,2,2,2,2,2,2,2,2,2,2,2,2,2,2,2,2,2,2,2,2,2,2,2,2,2,2,2,
2,2,2,2,2,2,2,2,2,2,2,2,2,4),(1.65479925748125,1.66859501726426,3.33719003452851,
5.00578505179277,6.67438006905703,7.50867757768916,8.34297508632129,9.17727259495341,
10.0115701035855,10.4287188579016,10.8458676122177,11.2630163665337,11.6801651208498,
12.0973138751659,12.5144626294819,12.72303700664,12.931611383798,13.140185760956,
13.3487601381141,13.5391016709644,13.6342724373896,13.7294432038147,13.8246139702399,
13.8721993534525,13.9197847366651,13.9673701198777,14.0149555030903,14.0387481946965,
14.0625408863028,14.0863335779091,14.0982299237123,14.1101262695154,14.1220370206378,
14.1339477717601,14.1399031473213,14.1458585228825,14.1488362106631,14.1518138984437,
14.1547915862243,14.1562804301146,14.1577692740048,14.158535003378,14.1593007327512,
14.1600664621244,14.160449326811),.UNSPECIFIED.) ;
#563=B_SPLINE_CURVE_WITH_KNOTS('',3,(#63107,#63108,#63109,#63110,#63111,
#63112,#63113,#63114,#63115,#63116,#63117,#63118,#63119,#63120,#63121,#63122,
#63123,#63124,#63125,#63126,#63127,#63128,#63129,#63130,#63131,#63132,#63133,
#63134,#63135,#63136,#63137,#63138,#63139,#63140,#63141,#63142,#63143,#63144,
#63145,#63146,#63147,#63148,#63149,#63150,#63151,#63152,#63153,#63154,#63155,
#63156,#63157,#63158,#63159,#63160,#63161,#63162,#63163,#63164,#63165,#63166,
#63167,#63168,#63169,#63170,#63171,#63172,#63173,#63174,#63175,#63176,#63177,
#63178,#63179,#63180,#63181,#63182,#63183,#63184,#63185,#63186,#63187,#63188,
#63189,#63190,#63191,#63192,#63193,#63194,#63195,#63196),.UNSPECIFIED.,
 .F.,.F.,(4,2,2,2,2,2,2,2,2,2,2,2,2,2,2,2,2,2,2,2,2,2,2,2,2,2,2,2,2,2,2,
2,2,2,2,2,2,2,2,2,2,2,2,2,4),(14.0450621959468,14.0454422411604,14.0462023315876,
14.0469624220149,14.0477225124421,14.049200222119,14.0506779317958,14.0536333511496,
14.0565887705033,14.0595441898571,14.0654550285646,14.071365867272,14.083187544687,
14.095009222102,14.1068157952781,14.1186223684541,14.1422355148063,14.1658486611584,
14.1894618075106,14.2366881002148,14.2839143929191,14.3311406856234,14.3783669783277,
14.4728195637362,14.5672721491448,14.6617247345534,14.8506299053705,15.0574774949646,
15.2643250845586,15.4711726741527,15.6780202637467,16.0917154429348,16.5054106221229,
16.919105801311,17.3328009804992,17.7464961596873,18.1601913388754,18.9875816972516,
19.8149720556278,20.642362414004,21.4697527723802,23.1245334891327,24.7793142058851,
26.4340949226375,26.553707914304),.UNSPECIFIED.) ;
#564=B_SPLINE_CURVE_WITH_KNOTS('',3,(#63197,#63198,#63199,#63200,#63201,
#63202,#63203,#63204,#63205,#63206,#63207,#63208,#63209,#63210,#63211,#63212,
#63213,#63214,#63215,#63216,#63217,#63218,#63219,#63220,#63221,#63222,#63223,
#63224,#63225,#63226,#63227,#63228,#63229,#63230,#63231,#63232,#63233,#63234,
#63235,#63236,#63237,#63238,#63239,#63240,#63241,#63242,#63243,#63244,#63245,
#63246,#63247,#63248,#63249,#63250,#63251,#63252,#63253,#63254,#63255,#63256,
#63257,#63258,#63259,#63260,#63261,#63262,#63263,#63264,#63265,#63266,#63267,
#63268,#63269,#63270,#63271,#63272,#63273,#63274,#63275,#63276,#63277,#63278,
#63279,#63280,#63281,#63282,#63283,#63284,#63285,#63286),.UNSPECIFIED.,
 .F.,.F.,(4,2,2,2,2,2,2,2,2,2,2,2,2,2,2,2,2,2,2,2,2,2,2,2,2,2,2,2,2,2,2,
2,2,2,2,2,2,2,2,2,2,2,2,2,4),(1.5351677250863,1.654780716772,3.30956143354401,
4.96434215031601,6.61912286708802,7.44651322547402,8.27390358386002,9.10129394224603,
9.92868430063203,10.342379479825,10.756074659018,11.169769838211,11.583465017404,
11.997160196597,12.41085537579,12.6177029653865,12.824550554983,13.0313981445795,
13.238245734176,13.4271509053336,13.5216034909124,13.6160560764912,13.71050866207,
13.7577349548593,13.8049612476487,13.8521875404381,13.8994138332275,13.9230269796222,
13.9466401260169,13.9702532724116,13.982059845609,13.9938664188063,14.0056880957911,
14.0175097727758,14.0234206112682,14.0293314497606,14.0322868690068,14.035242288253,
14.0381977074992,14.0396754171223,14.0411531267454,14.0419132173428,14.0426733079402,
14.0434333985377,14.0438134438364),.UNSPECIFIED.) ;
#576=SHAPE_REPRESENTATION_RELATIONSHIP('SRR','None',#63890,#591) ;
#591=ADVANCED_BREP_SHAPE_REPRESENTATION('',(#621),#63820) ;
#606=STYLED_ITEM('',(#63963),#621) ;
#621=MANIFOLD_SOLID_BREP('Body1',#15505) ;
#759=FACE_BOUND('',#3239,.T.) ;
#760=FACE_BOUND('',#3240,.T.) ;
#761=FACE_BOUND('',#3243,.T.) ;
#762=FACE_BOUND('',#3244,.T.) ;
#763=FACE_BOUND('',#3245,.T.) ;
#764=FACE_BOUND('',#3246,.T.) ;
#765=FACE_BOUND('',#3247,.T.) ;
#766=FACE_BOUND('',#3248,.T.) ;
#767=FACE_BOUND('',#3249,.T.) ;
#768=FACE_BOUND('',#3250,.T.) ;
#769=FACE_BOUND('',#3251,.T.) ;
#770=FACE_BOUND('',#3252,.T.) ;
#771=FACE_BOUND('',#3253,.T.) ;
#772=FACE_BOUND('',#3254,.T.) ;
#773=FACE_BOUND('',#3255,.T.) ;
#774=FACE_BOUND('',#3256,.T.) ;
#775=FACE_BOUND('',#3257,.T.) ;
#776=FACE_BOUND('',#3258,.T.) ;
#777=FACE_BOUND('',#3259,.T.) ;
#778=FACE_BOUND('',#3260,.T.) ;
#779=FACE_BOUND('',#3261,.T.) ;
#780=FACE_BOUND('',#3262,.T.) ;
#781=FACE_BOUND('',#3263,.T.) ;
#782=FACE_BOUND('',#3264,.T.) ;
#783=FACE_BOUND('',#3265,.T.) ;
#784=FACE_BOUND('',#3266,.T.) ;
#785=FACE_BOUND('',#3267,.T.) ;
#786=FACE_BOUND('',#3268,.T.) ;
#787=FACE_BOUND('',#3269,.T.) ;
#788=FACE_BOUND('',#3270,.T.) ;
#789=FACE_BOUND('',#3271,.T.) ;
#790=FACE_BOUND('',#3280,.T.) ;
#791=FACE_BOUND('',#3282,.T.) ;
#792=FACE_BOUND('',#3284,.T.) ;
#793=FACE_BOUND('',#3314,.T.) ;
#1048=PLANE('',#17507) ;
#1049=PLANE('',#17508) ;
#1050=PLANE('',#17509) ;
#1051=PLANE('',#17510) ;
#1052=PLANE('',#17513) ;
#1053=PLANE('',#17516) ;
#1054=PLANE('',#17519) ;
#1055=PLANE('',#17522) ;
#1056=PLANE('',#17525) ;
#1057=PLANE('',#17528) ;
#1058=PLANE('',#17531) ;
#1059=PLANE('',#17534) ;
#1060=PLANE('',#17537) ;
#1061=PLANE('',#17540) ;
#1062=PLANE('',#17543) ;
#1063=PLANE('',#17546) ;
#1064=PLANE('',#17549) ;
#1065=PLANE('',#17552) ;
#1066=PLANE('',#17555) ;
#1067=PLANE('',#17558) ;
#1068=PLANE('',#17561) ;
#1069=PLANE('',#17564) ;
#1070=PLANE('',#17567) ;
#1071=PLANE('',#17570) ;
#1072=PLANE('',#17573) ;
#1073=PLANE('',#17576) ;
#1074=PLANE('',#17579) ;
#1075=PLANE('',#17582) ;
#1076=PLANE('',#17585) ;
#1077=PLANE('',#17588) ;
#1078=PLANE('',#17591) ;
#1079=PLANE('',#17594) ;
#1080=PLANE('',#17595) ;
#1081=PLANE('',#17602) ;
#1082=PLANE('',#17609) ;
#1083=PLANE('',#17616) ;
#1084=PLANE('',#17623) ;
#1085=PLANE('',#17630) ;
#1086=PLANE('',#17637) ;
#1087=PLANE('',#17644) ;
#1088=PLANE('',#17651) ;
#1089=PLANE('',#17658) ;
#1090=PLANE('',#17665) ;
#1091=PLANE('',#17672) ;
#1092=PLANE('',#17679) ;
#1093=PLANE('',#17686) ;
#1094=PLANE('',#17693) ;
#1095=PLANE('',#17700) ;
#1096=PLANE('',#17707) ;
#1097=PLANE('',#17714) ;
#1098=PLANE('',#17721) ;
#1099=PLANE('',#17728) ;
#1100=PLANE('',#17735) ;
#1101=PLANE('',#17742) ;
#1102=PLANE('',#17749) ;
#1103=PLANE('',#17756) ;
#1104=PLANE('',#17763) ;
#1105=PLANE('',#17770) ;
#1106=PLANE('',#17777) ;
#1107=PLANE('',#17784) ;
#1108=PLANE('',#17791) ;
#1109=PLANE('',#17798) ;
#1519=CYLINDRICAL_SURFACE('',#17394,29.3077933083081) ;
#1520=CYLINDRICAL_SURFACE('',#17486,27.082990178354) ;
#1521=CYLINDRICAL_SURFACE('',#17501,22.5) ;
#1522=CYLINDRICAL_SURFACE('',#17506,37.5) ;
#2242=FACE_OUTER_BOUND('',#3237,.T.) ;
#2243=FACE_OUTER_BOUND('',#3238,.T.) ;
#2244=FACE_OUTER_BOUND('',#3241,.T.) ;
#2245=FACE_OUTER_BOUND('',#3242,.T.) ;
#2246=FACE_OUTER_BOUND('',#3272,.T.) ;
#2247=FACE_OUTER_BOUND('',#3273,.T.) ;
#2248=FACE_OUTER_BOUND('',#3274,.T.) ;
#2249=FACE_OUTER_BOUND('',#3275,.T.) ;
#2250=FACE_OUTER_BOUND('',#3276,.T.) ;
#2251=FACE_OUTER_BOUND('',#3277,.T.) ;
#2252=FACE_OUTER_BOUND('',#3278,.T.) ;
#2253=FACE_OUTER_BOUND('',#3279,.T.) ;
#2254=FACE_OUTER_BOUND('',#3281,.T.) ;
#2255=FACE_OUTER_BOUND('',#3283,.T.) ;
#2256=FACE_OUTER_BOUND('',#3285,.T.) ;
#2257=FACE_OUTER_BOUND('',#3286,.T.) ;
#2258=FACE_OUTER_BOUND('',#3287,.T.) ;
#2259=FACE_OUTER_BOUND('',#3288,.T.) ;
#2260=FACE_OUTER_BOUND('',#3289,.T.) ;
#2261=FACE_OUTER_BOUND('',#3290,.T.) ;
#2262=FACE_OUTER_BOUND('',#3291,.T.) ;
#2263=FACE_OUTER_BOUND('',#3292,.T.) ;
#2264=FACE_OUTER_BOUND('',#3293,.T.) ;
#2265=FACE_OUTER_BOUND('',#3294,.T.) ;
#2266=FACE_OUTER_BOUND('',#3295,.T.) ;
#2267=FACE_OUTER_BOUND('',#3296,.T.) ;
#2268=FACE_OUTER_BOUND('',#3297,.T.) ;
#2269=FACE_OUTER_BOUND('',#3298,.T.) ;
#2270=FACE_OUTER_BOUND('',#3299,.T.) ;
#2271=FACE_OUTER_BOUND('',#3300,.T.) ;
#2272=FACE_OUTER_BOUND('',#3301,.T.) ;
#2273=FACE_OUTER_BOUND('',#3302,.T.) ;
#2274=FACE_OUTER_BOUND('',#3303,.T.) ;
#2275=FACE_OUTER_BOUND('',#3304,.T.) ;
#2276=FACE_OUTER_BOUND('',#3305,.T.) ;
#2277=FACE_OUTER_BOUND('',#3306,.T.) ;
#2278=FACE_OUTER_BOUND('',#3307,.T.) ;
#2279=FACE_OUTER_BOUND('',#3308,.T.) ;
#2280=FACE_OUTER_BOUND('',#3309,.T.) ;
#2281=FACE_OUTER_BOUND('',#3310,.T.) ;
#2282=FACE_OUTER_BOUND('',#3311,.T.) ;
#2283=FACE_OUTER_BOUND('',#3312,.T.) ;
#2284=FACE_OUTER_BOUND('',#3313,.T.) ;
#2285=FACE_OUTER_BOUND('',#3315,.T.) ;
#2286=FACE_OUTER_BOUND('',#3316,.T.) ;
#2287=FACE_OUTER_BOUND('',#3317,.T.) ;
#2288=FACE_OUTER_BOUND('',#3318,.T.) ;
#2289=FACE_OUTER_BOUND('',#3319,.T.) ;
#2290=FACE_OUTER_BOUND('',#3320,.T.) ;
#2291=FACE_OUTER_BOUND('',#3321,.T.) ;
#2292=FACE_OUTER_BOUND('',#3322,.T.) ;
#2293=FACE_OUTER_BOUND('',#3323,.T.) ;
#2294=FACE_OUTER_BOUND('',#3324,.T.) ;
#2295=FACE_OUTER_BOUND('',#3325,.T.) ;
#2296=FACE_OUTER_BOUND('',#3326,.T.) ;
#2297=FACE_OUTER_BOUND('',#3327,.T.) ;
#2298=FACE_OUTER_BOUND('',#3328,.T.) ;
#2299=FACE_OUTER_BOUND('',#3329,.T.) ;
#2300=FACE_OUTER_BOUND('',#3330,.T.) ;
#2301=FACE_OUTER_BOUND('',#3331,.T.) ;
#2302=FACE_OUTER_BOUND('',#3332,.T.) ;
#2303=FACE_OUTER_BOUND('',#3333,.T.) ;
#2304=FACE_OUTER_BOUND('',#3334,.T.) ;
#2305=FACE_OUTER_BOUND('',#3335,.T.) ;
#2306=FACE_OUTER_BOUND('',#3336,.T.) ;
#2307=FACE_OUTER_BOUND('',#3337,.T.) ;
#2308=FACE_OUTER_BOUND('',#3338,.T.) ;
#2309=FACE_OUTER_BOUND('',#3339,.T.) ;
#2310=FACE_OUTER_BOUND('',#3340,.T.) ;
#2311=FACE_OUTER_BOUND('',#3341,.T.) ;
#2312=FACE_OUTER_BOUND('',#3342,.T.) ;
#2313=FACE_OUTER_BOUND('',#3343,.T.) ;
#2314=FACE_OUTER_BOUND('',#3344,.T.) ;
#2315=FACE_OUTER_BOUND('',#3345,.T.) ;
#2316=FACE_OUTER_BOUND('',#3346,.T.) ;
#2317=FACE_OUTER_BOUND('',#3347,.T.) ;
#2318=FACE_OUTER_BOUND('',#3348,.T.) ;
#2319=FACE_OUTER_BOUND('',#3349,.T.) ;
#2320=FACE_OUTER_BOUND('',#3350,.T.) ;
#2321=FACE_OUTER_BOUND('',#3351,.T.) ;
#2322=FACE_OUTER_BOUND('',#3352,.T.) ;
#2323=FACE_OUTER_BOUND('',#3353,.T.) ;
#2324=FACE_OUTER_BOUND('',#3354,.T.) ;
#2325=FACE_OUTER_BOUND('',#3355,.T.) ;
#2326=FACE_OUTER_BOUND('',#3356,.T.) ;
#2327=FACE_OUTER_BOUND('',#3357,.T.) ;
#2328=FACE_OUTER_BOUND('',#3358,.T.) ;
#2329=FACE_OUTER_BOUND('',#3359,.T.) ;
#2330=FACE_OUTER_BOUND('',#3360,.T.) ;
#2331=FACE_OUTER_BOUND('',#3361,.T.) ;
#2332=FACE_OUTER_BOUND('',#3362,.T.) ;
#2333=FACE_OUTER_BOUND('',#3363,.T.) ;
#2334=FACE_OUTER_BOUND('',#3364,.T.) ;
#2335=FACE_OUTER_BOUND('',#3365,.T.) ;
#2336=FACE_OUTER_BOUND('',#3366,.T.) ;
#2337=FACE_OUTER_BOUND('',#3367,.T.) ;
#2338=FACE_OUTER_BOUND('',#3368,.T.) ;
#2339=FACE_OUTER_BOUND('',#3369,.T.) ;
#2340=FACE_OUTER_BOUND('',#3370,.T.) ;
#2341=FACE_OUTER_BOUND('',#3371,.T.) ;
#2342=FACE_OUTER_BOUND('',#3372,.T.) ;
#2343=FACE_OUTER_BOUND('',#3373,.T.) ;
#2344=FACE_OUTER_BOUND('',#3374,.T.) ;
#2345=FACE_OUTER_BOUND('',#3375,.T.) ;
#2346=FACE_OUTER_BOUND('',#3376,.T.) ;
#2347=FACE_OUTER_BOUND('',#3377,.T.) ;
#2348=FACE_OUTER_BOUND('',#3378,.T.) ;
#2349=FACE_OUTER_BOUND('',#3379,.T.) ;
#2350=FACE_OUTER_BOUND('',#3380,.T.) ;
#2351=FACE_OUTER_BOUND('',#3381,.T.) ;
#2352=FACE_OUTER_BOUND('',#3382,.T.) ;
#2353=FACE_OUTER_BOUND('',#3383,.T.) ;
#2354=FACE_OUTER_BOUND('',#3384,.T.) ;
#2355=FACE_OUTER_BOUND('',#3385,.T.) ;
#2356=FACE_OUTER_BOUND('',#3386,.T.) ;
#2357=FACE_OUTER_BOUND('',#3387,.T.) ;
#2358=FACE_OUTER_BOUND('',#3388,.T.) ;
#2359=FACE_OUTER_BOUND('',#3389,.T.) ;
#2360=FACE_OUTER_BOUND('',#3390,.T.) ;
#2361=FACE_OUTER_BOUND('',#3391,.T.) ;
#2362=FACE_OUTER_BOUND('',#3392,.T.) ;
#2363=FACE_OUTER_BOUND('',#3393,.T.) ;
#2364=FACE_OUTER_BOUND('',#3394,.T.) ;
#2365=FACE_OUTER_BOUND('',#3395,.T.) ;
#2366=FACE_OUTER_BOUND('',#3396,.T.) ;
#2367=FACE_OUTER_BOUND('',#3397,.T.) ;
#2368=FACE_OUTER_BOUND('',#3398,.T.) ;
#2369=FACE_OUTER_BOUND('',#3399,.T.) ;
#2370=FACE_OUTER_BOUND('',#3400,.T.) ;
#2371=FACE_OUTER_BOUND('',#3401,.T.) ;
#2372=FACE_OUTER_BOUND('',#3402,.T.) ;
#2373=FACE_OUTER_BOUND('',#3403,.T.) ;
#3237=EDGE_LOOP('',(#12958,#12959,#12960,#12961,#12962,#12963,#12964,#12965,
#12966,#12967,#12968,#12969,#12970,#12971,#12972,#12973,#12974,#12975,#12976,
#12977,#12978,#12979,#12980,#12981,#12982,#12983,#12984,#12985,#12986,#12987,
#12988,#12989,#12990,#12991,#12992,#12993,#12994,#12995,#12996,#12997,#12998,
#12999,#13000,#13001,#13002,#13003,#13004,#13005,#13006,#13007,#13008,#13009,
#13010,#13011,#13012,#13013,#13014,#13015,#13016,#13017,#13018,#13019,#13020,
#13021,#13022,#13023,#13024,#13025,#13026,#13027,#13028,#13029,#13030,#13031,
#13032,#13033,#13034,#13035,#13036,#13037,#13038,#13039,#13040,#13041,#13042,
#13043,#13044,#13045,#13046,#13047,#13048,#13049,#13050,#13051,#13052,#13053,
#13054,#13055,#13056,#13057,#13058,#13059,#13060,#13061,#13062,#13063,#13064,
#13065,#13066,#13067,#13068,#13069,#13070,#13071,#13072,#13073,#13074,#13075,
#13076,#13077,#13078,#13079,#13080,#13081,#13082,#13083,#13084,#13085,#13086,
#13087,#13088,#13089,#13090,#13091,#13092,#13093,#13094,#13095,#13096,#13097,
#13098,#13099,#13100,#13101,#13102,#13103,#13104,#13105,#13106,#13107,#13108,
#13109,#13110,#13111,#13112,#13113,#13114,#13115,#13116,#13117,#13118,#13119,
#13120,#13121,#13122,#13123,#13124,#13125,#13126,#13127,#13128,#13129,#13130,
#13131,#13132,#13133,#13134,#13135)) ;
#3238=EDGE_LOOP('',(#13136,#13137,#13138,#13139,#13140,#13141,#13142,#13143,
#13144,#13145,#13146,#13147,#13148,#13149,#13150,#13151,#13152,#13153,#13154,
#13155,#13156,#13157,#13158,#13159,#13160,#13161,#13162,#13163,#13164,#13165,
#13166,#13167,#13168,#13169,#13170,#13171,#13172,#13173,#13174,#13175,#13176,
#13177,#13178,#13179,#13180,#13181,#13182,#13183,#13184,#13185,#13186,#13187,
#13188,#13189,#13190,#13191,#13192,#13193,#13194,#13195,#13196,#13197,#13198,
#13199,#13200,#13201,#13202,#13203,#13204,#13205,#13206,#13207,#13208,#13209,
#13210,#13211,#13212,#13213,#13214,#13215,#13216,#13217,#13218,#13219,#13220,
#13221,#13222,#13223,#13224,#13225,#13226,#13227,#13228,#13229,#13230,#13231,
#13232,#13233,#13234,#13235,#13236,#13237,#13238,#13239,#13240,#13241,#13242,
#13243,#13244,#13245,#13246,#13247,#13248,#13249)) ;
#3239=EDGE_LOOP('',(#13250,#13251,#13252)) ;
#3240=EDGE_LOOP('',(#13253,#13254,#13255)) ;
#3241=EDGE_LOOP('',(#13256,#13257,#13258,#13259,#13260,#13261,#13262,#13263,
#13264,#13265,#13266,#13267,#13268,#13269,#13270,#13271,#13272,#13273,#13274,
#13275,#13276,#13277,#13278,#13279,#13280,#13281,#13282,#13283,#13284,#13285,
#13286,#13287,#13288,#13289,#13290,#13291,#13292,#13293,#13294,#13295,#13296,
#13297,#13298,#13299,#13300,#13301,#13302,#13303,#13304,#13305,#13306,#13307,
#13308,#13309,#13310,#13311,#13312,#13313,#13314,#13315,#13316,#13317,#13318,
#13319,#13320,#13321,#13322,#13323,#13324,#13325,#13326,#13327,#13328,#13329,
#13330,#13331,#13332,#13333,#13334,#13335,#13336,#13337,#13338,#13339,#13340,
#13341,#13342,#13343,#13344,#13345,#13346,#13347,#13348,#13349,#13350,#13351,
#13352,#13353,#13354,#13355,#13356,#13357,#13358,#13359,#13360,#13361,#13362,
#13363,#13364,#13365,#13366,#13367,#13368,#13369,#13370,#13371,#13372,#13373,
#13374,#13375,#13376,#13377,#13378,#13379,#13380,#13381,#13382,#13383,#13384,
#13385,#13386,#13387,#13388,#13389,#13390,#13391,#13392,#13393,#13394,#13395,
#13396,#13397,#13398,#13399,#13400,#13401,#13402,#13403,#13404,#13405,#13406,
#13407,#13408,#13409,#13410,#13411,#13412,#13413,#13414,#13415,#13416,#13417,
#13418,#13419,#13420,#13421,#13422,#13423,#13424,#13425,#13426,#13427,#13428,
#13429,#13430,#13431,#13432,#13433)) ;
#3242=EDGE_LOOP('',(#13434,#13435,#13436,#13437)) ;
#3243=EDGE_LOOP('',(#13438,#13439,#13440)) ;
#3244=EDGE_LOOP('',(#13441,#13442,#13443)) ;
#3245=EDGE_LOOP('',(#13444,#13445,#13446)) ;
#3246=EDGE_LOOP('',(#13447,#13448,#13449)) ;
#3247=EDGE_LOOP('',(#13450,#13451,#13452)) ;
#3248=EDGE_LOOP('',(#13453,#13454,#13455)) ;
#3249=EDGE_LOOP('',(#13456,#13457,#13458)) ;
#3250=EDGE_LOOP('',(#13459,#13460,#13461)) ;
#3251=EDGE_LOOP('',(#13462,#13463,#13464)) ;
#3252=EDGE_LOOP('',(#13465,#13466,#13467)) ;
#3253=EDGE_LOOP('',(#13468,#13469,#13470)) ;
#3254=EDGE_LOOP('',(#13471,#13472,#13473)) ;
#3255=EDGE_LOOP('',(#13474,#13475,#13476)) ;
#3256=EDGE_LOOP('',(#13477,#13478,#13479)) ;
#3257=EDGE_LOOP('',(#13480,#13481,#13482)) ;
#3258=EDGE_LOOP('',(#13483,#13484,#13485)) ;
#3259=EDGE_LOOP('',(#13486,#13487,#13488)) ;
#3260=EDGE_LOOP('',(#13489,#13490,#13491)) ;
#3261=EDGE_LOOP('',(#13492,#13493,#13494)) ;
#3262=EDGE_LOOP('',(#13495,#13496,#13497)) ;
#3263=EDGE_LOOP('',(#13498,#13499,#13500)) ;
#3264=EDGE_LOOP('',(#13501,#13502,#13503)) ;
#3265=EDGE_LOOP('',(#13504,#13505,#13506)) ;
#3266=EDGE_LOOP('',(#13507,#13508,#13509)) ;
#3267=EDGE_LOOP('',(#13510,#13511,#13512)) ;
#3268=EDGE_LOOP('',(#13513,#13514,#13515)) ;
#3269=EDGE_LOOP('',(#13516,#13517,#13518)) ;
#3270=EDGE_LOOP('',(#13519,#13520,#13521)) ;
#3271=EDGE_LOOP('',(#13522,#13523,#13524)) ;
#3272=EDGE_LOOP('',(#13525,#13526,#13527,#13528)) ;
#3273=EDGE_LOOP('',(#13529,#13530,#13531,#13532)) ;
#3274=EDGE_LOOP('',(#13533,#13534,#13535,#13536)) ;
#3275=EDGE_LOOP('',(#13537,#13538,#13539,#13540)) ;
#3276=EDGE_LOOP('',(#13541,#13542,#13543,#13544)) ;
#3277=EDGE_LOOP('',(#13545,#13546,#13547,#13548)) ;
#3278=EDGE_LOOP('',(#13549,#13550,#13551,#13552)) ;
#3279=EDGE_LOOP('',(#13553)) ;
#3280=EDGE_LOOP('',(#13554)) ;
#3281=EDGE_LOOP('',(#13555)) ;
#3282=EDGE_LOOP('',(#13556)) ;
#3283=EDGE_LOOP('',(#13557)) ;
#3284=EDGE_LOOP('',(#13558)) ;
#3285=EDGE_LOOP('',(#13559,#13560)) ;
#3286=EDGE_LOOP('',(#13561,#13562)) ;
#3287=EDGE_LOOP('',(#13563,#13564)) ;
#3288=EDGE_LOOP('',(#13565,#13566)) ;
#3289=EDGE_LOOP('',(#13567,#13568)) ;
#3290=EDGE_LOOP('',(#13569,#13570)) ;
#3291=EDGE_LOOP('',(#13571,#13572)) ;
#3292=EDGE_LOOP('',(#13573,#13574)) ;
#3293=EDGE_LOOP('',(#13575,#13576)) ;
#3294=EDGE_LOOP('',(#13577,#13578)) ;
#3295=EDGE_LOOP('',(#13579,#13580)) ;
#3296=EDGE_LOOP('',(#13581,#13582)) ;
#3297=EDGE_LOOP('',(#13583,#13584)) ;
#3298=EDGE_LOOP('',(#13585,#13586)) ;
#3299=EDGE_LOOP('',(#13587,#13588)) ;
#3300=EDGE_LOOP('',(#13589,#13590)) ;
#3301=EDGE_LOOP('',(#13591,#13592)) ;
#3302=EDGE_LOOP('',(#13593,#13594)) ;
#3303=EDGE_LOOP('',(#13595,#13596)) ;
#3304=EDGE_LOOP('',(#13597,#13598)) ;
#3305=EDGE_LOOP('',(#13599,#13600)) ;
#3306=EDGE_LOOP('',(#13601,#13602)) ;
#3307=EDGE_LOOP('',(#13603,#13604)) ;
#3308=EDGE_LOOP('',(#13605,#13606)) ;
#3309=EDGE_LOOP('',(#13607,#13608)) ;
#3310=EDGE_LOOP('',(#13609,#13610)) ;
#3311=EDGE_LOOP('',(#13611,#13612)) ;
#3312=EDGE_LOOP('',(#13613,#13614)) ;
#3313=EDGE_LOOP('',(#13615)) ;
#3314=EDGE_LOOP('',(#13616)) ;
#3315=EDGE_LOOP('',(#13617,#13618)) ;
#3316=EDGE_LOOP('',(#13619,#13620,#13621,#13622,#13623,#13624,#13625,#13626,
#13627,#13628,#13629,#13630,#13631,#13632,#13633,#13634,#13635,#13636,#13637,
#13638,#13639,#13640,#13641,#13642,#13643,#13644,#13645,#13646,#13647,#13648,
#13649,#13650,#13651)) ;
#3317=EDGE_LOOP('',(#13652,#13653,#13654,#13655,#13656,#13657,#13658)) ;
#3318=EDGE_LOOP('',(#13659,#13660,#13661,#13662,#13663,#13664,#13665,#13666,
#13667,#13668)) ;
#3319=EDGE_LOOP('',(#13669,#13670,#13671,#13672,#13673,#13674,#13675)) ;
#3320=EDGE_LOOP('',(#13676,#13677,#13678,#13679,#13680,#13681,#13682)) ;
#3321=EDGE_LOOP('',(#13683,#13684,#13685,#13686,#13687,#13688,#13689,#13690,
#13691,#13692)) ;
#3322=EDGE_LOOP('',(#13693,#13694,#13695,#13696,#13697,#13698,#13699)) ;
#3323=EDGE_LOOP('',(#13700,#13701,#13702,#13703,#13704,#13705,#13706)) ;
#3324=EDGE_LOOP('',(#13707,#13708,#13709,#13710,#13711,#13712,#13713,#13714,
#13715,#13716)) ;
#3325=EDGE_LOOP('',(#13717,#13718,#13719,#13720,#13721,#13722,#13723)) ;
#3326=EDGE_LOOP('',(#13724,#13725,#13726,#13727,#13728,#13729,#13730)) ;
#3327=EDGE_LOOP('',(#13731,#13732,#13733,#13734,#13735,#13736,#13737,#13738,
#13739,#13740)) ;
#3328=EDGE_LOOP('',(#13741,#13742,#13743,#13744,#13745,#13746,#13747)) ;
#3329=EDGE_LOOP('',(#13748,#13749,#13750,#13751,#13752,#13753,#13754)) ;
#3330=EDGE_LOOP('',(#13755,#13756,#13757,#13758,#13759,#13760,#13761,#13762,
#13763,#13764)) ;
#3331=EDGE_LOOP('',(#13765,#13766,#13767,#13768,#13769,#13770,#13771)) ;
#3332=EDGE_LOOP('',(#13772,#13773,#13774,#13775,#13776,#13777,#13778)) ;
#3333=EDGE_LOOP('',(#13779,#13780,#13781,#13782,#13783,#13784,#13785,#13786,
#13787,#13788)) ;
#3334=EDGE_LOOP('',(#13789,#13790,#13791,#13792,#13793,#13794,#13795)) ;
#3335=EDGE_LOOP('',(#13796,#13797,#13798,#13799,#13800,#13801,#13802)) ;
#3336=EDGE_LOOP('',(#13803,#13804,#13805,#13806,#13807,#13808,#13809,#13810,
#13811,#13812)) ;
#3337=EDGE_LOOP('',(#13813,#13814,#13815,#13816,#13817,#13818,#13819)) ;
#3338=EDGE_LOOP('',(#13820,#13821,#13822,#13823,#13824,#13825,#13826)) ;
#3339=EDGE_LOOP('',(#13827,#13828,#13829,#13830,#13831,#13832,#13833,#13834,
#13835,#13836)) ;
#3340=EDGE_LOOP('',(#13837,#13838,#13839,#13840,#13841,#13842,#13843)) ;
#3341=EDGE_LOOP('',(#13844,#13845,#13846,#13847,#13848,#13849,#13850)) ;
#3342=EDGE_LOOP('',(#13851,#13852,#13853,#13854,#13855,#13856,#13857,#13858,
#13859,#13860)) ;
#3343=EDGE_LOOP('',(#13861,#13862,#13863,#13864,#13865,#13866,#13867)) ;
#3344=EDGE_LOOP('',(#13868,#13869,#13870,#13871,#13872,#13873,#13874)) ;
#3345=EDGE_LOOP('',(#13875,#13876,#13877,#13878,#13879,#13880,#13881,#13882,
#13883,#13884)) ;
#3346=EDGE_LOOP('',(#13885,#13886,#13887,#13888,#13889,#13890,#13891)) ;
#3347=EDGE_LOOP('',(#13892,#13893,#13894,#13895,#13896,#13897,#13898)) ;
#3348=EDGE_LOOP('',(#13899,#13900,#13901,#13902,#13903,#13904,#13905,#13906,
#13907,#13908)) ;
#3349=EDGE_LOOP('',(#13909,#13910,#13911,#13912,#13913,#13914,#13915)) ;
#3350=EDGE_LOOP('',(#13916,#13917,#13918,#13919,#13920,#13921,#13922)) ;
#3351=EDGE_LOOP('',(#13923,#13924,#13925,#13926,#13927,#13928,#13929,#13930,
#13931,#13932)) ;
#3352=EDGE_LOOP('',(#13933,#13934,#13935,#13936,#13937,#13938,#13939)) ;
#3353=EDGE_LOOP('',(#13940,#13941,#13942,#13943,#13944,#13945,#13946)) ;
#3354=EDGE_LOOP('',(#13947,#13948,#13949,#13950,#13951,#13952,#13953,#13954,
#13955,#13956)) ;
#3355=EDGE_LOOP('',(#13957,#13958,#13959,#13960,#13961,#13962,#13963)) ;
#3356=EDGE_LOOP('',(#13964,#13965,#13966,#13967,#13968,#13969,#13970)) ;
#3357=EDGE_LOOP('',(#13971,#13972,#13973,#13974,#13975,#13976,#13977,#13978,
#13979,#13980)) ;
#3358=EDGE_LOOP('',(#13981,#13982,#13983,#13984,#13985,#13986,#13987)) ;
#3359=EDGE_LOOP('',(#13988,#13989,#13990,#13991,#13992,#13993,#13994)) ;
#3360=EDGE_LOOP('',(#13995,#13996,#13997,#13998,#13999,#14000,#14001,#14002,
#14003,#14004)) ;
#3361=EDGE_LOOP('',(#14005,#14006,#14007,#14008,#14009,#14010,#14011)) ;
#3362=EDGE_LOOP('',(#14012,#14013,#14014,#14015,#14016,#14017,#14018)) ;
#3363=EDGE_LOOP('',(#14019,#14020,#14021,#14022,#14023,#14024,#14025,#14026,
#14027,#14028)) ;
#3364=EDGE_LOOP('',(#14029,#14030,#14031,#14032,#14033,#14034,#14035)) ;
#3365=EDGE_LOOP('',(#14036,#14037,#14038,#14039,#14040,#14041,#14042)) ;
#3366=EDGE_LOOP('',(#14043,#14044,#14045,#14046,#14047,#14048,#14049,#14050,
#14051,#14052)) ;
#3367=EDGE_LOOP('',(#14053,#14054,#14055,#14056,#14057,#14058,#14059)) ;
#3368=EDGE_LOOP('',(#14060,#14061,#14062,#14063,#14064,#14065,#14066)) ;
#3369=EDGE_LOOP('',(#14067,#14068,#14069,#14070,#14071,#14072,#14073,#14074,
#14075,#14076)) ;
#3370=EDGE_LOOP('',(#14077,#14078,#14079,#14080,#14081,#14082,#14083)) ;
#3371=EDGE_LOOP('',(#14084,#14085,#14086,#14087,#14088,#14089,#14090)) ;
#3372=EDGE_LOOP('',(#14091,#14092,#14093,#14094,#14095,#14096,#14097,#14098,
#14099,#14100)) ;
#3373=EDGE_LOOP('',(#14101,#14102,#14103,#14104,#14105,#14106,#14107)) ;
#3374=EDGE_LOOP('',(#14108,#14109,#14110,#14111,#14112,#14113,#14114)) ;
#3375=EDGE_LOOP('',(#14115,#14116,#14117,#14118,#14119,#14120,#14121,#14122,
#14123,#14124)) ;
#3376=EDGE_LOOP('',(#14125,#14126,#14127,#14128,#14129,#14130,#14131)) ;
#3377=EDGE_LOOP('',(#14132,#14133,#14134,#14135,#14136,#14137,#14138)) ;
#3378=EDGE_LOOP('',(#14139,#14140,#14141,#14142,#14143,#14144,#14145,#14146,
#14147,#14148)) ;
#3379=EDGE_LOOP('',(#14149,#14150,#14151,#14152,#14153,#14154,#14155)) ;
#3380=EDGE_LOOP('',(#14156,#14157,#14158,#14159,#14160,#14161,#14162)) ;
#3381=EDGE_LOOP('',(#14163,#14164,#14165,#14166,#14167,#14168,#14169,#14170,
#14171,#14172)) ;
#3382=EDGE_LOOP('',(#14173,#14174,#14175,#14176,#14177,#14178,#14179)) ;
#3383=EDGE_LOOP('',(#14180,#14181,#14182,#14183,#14184,#14185,#14186)) ;
#3384=EDGE_LOOP('',(#14187,#14188,#14189,#14190,#14191,#14192,#14193,#14194,
#14195,#14196)) ;
#3385=EDGE_LOOP('',(#14197,#14198,#14199,#14200,#14201,#14202,#14203)) ;
#3386=EDGE_LOOP('',(#14204,#14205,#14206,#14207,#14208,#14209,#14210)) ;
#3387=EDGE_LOOP('',(#14211,#14212,#14213,#14214,#14215,#14216,#14217,#14218,
#14219,#14220)) ;
#3388=EDGE_LOOP('',(#14221,#14222,#14223,#14224,#14225,#14226,#14227)) ;
#3389=EDGE_LOOP('',(#14228,#14229,#14230,#14231,#14232,#14233,#14234)) ;
#3390=EDGE_LOOP('',(#14235,#14236,#14237,#14238,#14239,#14240,#14241,#14242,
#14243,#14244)) ;
#3391=EDGE_LOOP('',(#14245,#14246,#14247,#14248,#14249,#14250,#14251)) ;
#3392=EDGE_LOOP('',(#14252,#14253,#14254,#14255,#14256,#14257,#14258)) ;
#3393=EDGE_LOOP('',(#14259,#14260,#14261,#14262,#14263,#14264,#14265,#14266,
#14267,#14268)) ;
#3394=EDGE_LOOP('',(#14269,#14270,#14271,#14272,#14273,#14274,#14275)) ;
#3395=EDGE_LOOP('',(#14276,#14277,#14278,#14279,#14280,#14281,#14282)) ;
#3396=EDGE_LOOP('',(#14283,#14284,#14285,#14286,#14287,#14288,#14289,#14290,
#14291,#14292)) ;
#3397=EDGE_LOOP('',(#14293,#14294,#14295,#14296,#14297,#14298,#14299)) ;
#3398=EDGE_LOOP('',(#14300,#14301,#14302,#14303,#14304,#14305,#14306)) ;
#3399=EDGE_LOOP('',(#14307,#14308,#14309,#14310,#14311,#14312,#14313,#14314,
#14315,#14316)) ;
#3400=EDGE_LOOP('',(#14317,#14318,#14319,#14320,#14321,#14322,#14323)) ;
#3401=EDGE_LOOP('',(#14324,#14325,#14326,#14327,#14328,#14329,#14330)) ;
#3402=EDGE_LOOP('',(#14331,#14332,#14333,#14334,#14335,#14336,#14337,#14338,
#14339,#14340)) ;
#3403=EDGE_LOOP('',(#14341,#14342,#14343,#14344,#14345,#14346,#14347)) ;
#4361=CIRCLE('',#17274,27.7395230264339) ;
#4362=CIRCLE('',#17275,29.3077933083081) ;
#4363=CIRCLE('',#17276,29.3077933083081) ;
#4364=CIRCLE('',#17277,29.3077933083081) ;
#4365=CIRCLE('',#17278,29.3077933083081) ;
#4366=CIRCLE('',#17279,29.3077933083081) ;
#4367=CIRCLE('',#17280,29.3077933083081) ;
#4368=CIRCLE('',#17281,29.3077933083081) ;
#4369=CIRCLE('',#17282,29.3077933083081) ;
#4370=CIRCLE('',#17283,29.3077933083081) ;
#4371=CIRCLE('',#17284,29.3077933083081) ;
#4372=CIRCLE('',#17285,29.3077933083081) ;
#4373=CIRCLE('',#17286,29.3077933083081) ;
#4374=CIRCLE('',#17287,29.3077933083081) ;
#4375=CIRCLE('',#17288,29.3077933083081) ;
#4376=CIRCLE('',#17289,29.3077933083081) ;
#4377=CIRCLE('',#17290,29.3077933083081) ;
#4378=CIRCLE('',#17291,29.3077933083081) ;
#4379=CIRCLE('',#17292,29.3077933083081) ;
#4380=CIRCLE('',#17293,29.3077933083081) ;
#4381=CIRCLE('',#17294,29.3077933083081) ;
#4382=CIRCLE('',#17295,29.3077933083081) ;
#4383=CIRCLE('',#17296,29.3077933083081) ;
#4384=CIRCLE('',#17297,29.3077933083081) ;
#4385=CIRCLE('',#17298,29.3077933083081) ;
#4386=CIRCLE('',#17299,29.3077933083081) ;
#4387=CIRCLE('',#17300,29.3077933083081) ;
#4388=CIRCLE('',#17301,29.3077933083081) ;
#4389=CIRCLE('',#17302,29.3077933083081) ;
#4390=CIRCLE('',#17303,29.3077933083081) ;
#4391=CIRCLE('',#17304,29.3077933083081) ;
#4392=CIRCLE('',#17305,29.3077933083081) ;
#4393=CIRCLE('',#17306,29.3077933083081) ;
#4394=CIRCLE('',#17307,29.3077933083081) ;
#4395=CIRCLE('',#17308,29.3077933083081) ;
#4396=CIRCLE('',#17309,29.3077933083081) ;
#4397=CIRCLE('',#17310,29.3077933083081) ;
#4398=CIRCLE('',#17311,29.3077933083081) ;
#4399=CIRCLE('',#17312,29.3077933083081) ;
#4400=CIRCLE('',#17313,29.3077933083081) ;
#4401=CIRCLE('',#17314,29.3077933083081) ;
#4402=CIRCLE('',#17315,29.3077933083081) ;
#4403=CIRCLE('',#17316,29.3077933083081) ;
#4404=CIRCLE('',#17317,29.3077933083081) ;
#4405=CIRCLE('',#17318,29.3077933083081) ;
#4406=CIRCLE('',#17319,29.3077933083081) ;
#4407=CIRCLE('',#17320,29.3077933083081) ;
#4408=CIRCLE('',#17321,29.3077933083081) ;
#4409=CIRCLE('',#17322,29.3077933083081) ;
#4410=CIRCLE('',#17323,29.3077933083081) ;
#4411=CIRCLE('',#17324,29.3077933083081) ;
#4412=CIRCLE('',#17325,29.3077933083081) ;
#4413=CIRCLE('',#17326,29.3077933083081) ;
#4414=CIRCLE('',#17327,29.3077933083081) ;
#4415=CIRCLE('',#17328,29.3077933083081) ;
#4416=CIRCLE('',#17329,29.3077933083081) ;
#4417=CIRCLE('',#17330,29.3077933083081) ;
#4418=CIRCLE('',#17331,29.3077933083081) ;
#4419=CIRCLE('',#17332,29.3077933083081) ;
#4420=CIRCLE('',#17333,29.3077933083081) ;
#4421=CIRCLE('',#17335,25.5228270063586) ;
#4422=CIRCLE('',#17337,25.5228270063586) ;
#4423=CIRCLE('',#17339,25.5228270063586) ;
#4424=CIRCLE('',#17341,25.5228270063586) ;
#4425=CIRCLE('',#17343,25.5228270063586) ;
#4426=CIRCLE('',#17345,25.5228270063586) ;
#4427=CIRCLE('',#17347,25.5228270063586) ;
#4428=CIRCLE('',#17349,25.5228270063586) ;
#4429=CIRCLE('',#17351,25.5228270063586) ;
#4430=CIRCLE('',#17352,25.5228270063586) ;
#4431=CIRCLE('',#17354,25.5228270063586) ;
#4432=CIRCLE('',#17356,25.5228270063586) ;
#4433=CIRCLE('',#17358,25.5228270063586) ;
#4434=CIRCLE('',#17360,25.5228270063586) ;
#4435=CIRCLE('',#17361,25.5228270063586) ;
#4436=CIRCLE('',#17363,25.5228270063586) ;
#4437=CIRCLE('',#17365,25.5228270063586) ;
#4438=CIRCLE('',#17367,25.5228270063586) ;
#4439=CIRCLE('',#17369,25.5228270063586) ;
#4440=CIRCLE('',#17371,25.5228270063586) ;
#4441=CIRCLE('',#17373,25.5228270063586) ;
#4442=CIRCLE('',#17375,25.5228270063586) ;
#4443=CIRCLE('',#17377,25.5228270063586) ;
#4444=CIRCLE('',#17379,25.5228270063586) ;
#4445=CIRCLE('',#17381,25.5228270063586) ;
#4446=CIRCLE('',#17383,25.5228270063586) ;
#4447=CIRCLE('',#17385,25.5228270063586) ;
#4448=CIRCLE('',#17387,25.5228270063586) ;
#4449=CIRCLE('',#17389,25.5228270063586) ;
#4450=CIRCLE('',#17391,25.5228270063586) ;
#4451=CIRCLE('',#17453,29.3077933083081) ;
#4452=CIRCLE('',#17455,30.8653235080594) ;
#4453=CIRCLE('',#17456,34.0685435652414) ;
#4454=CIRCLE('',#17487,27.082990178354) ;
#4455=CIRCLE('',#17488,27.082990178354) ;
#4456=CIRCLE('',#17490,23.5) ;
#4457=CIRCLE('',#17491,1.) ;
#4458=CIRCLE('',#17492,22.5) ;
#4459=CIRCLE('',#17494,36.5) ;
#4460=CIRCLE('',#17495,1.) ;
#4461=CIRCLE('',#17496,37.5) ;
#4462=CIRCLE('',#17498,37.5) ;
#4463=CIRCLE('',#17499,0.25) ;
#4464=CIRCLE('',#17500,37.25) ;
#4465=CIRCLE('',#17502,22.5) ;
#4466=CIRCLE('',#17504,0.249999999999998) ;
#4467=CIRCLE('',#17505,22.75) ;
#4468=CIRCLE('',#17511,2.91746266896347) ;
#4469=CIRCLE('',#17512,2.91746266896347) ;
#4470=CIRCLE('',#17514,2.91746266896347) ;
#4471=CIRCLE('',#17515,2.91746266896347) ;
#4472=CIRCLE('',#17517,2.91746266896347) ;
#4473=CIRCLE('',#17518,2.91746266896347) ;
#4474=CIRCLE('',#17520,2.91746266896347) ;
#4475=CIRCLE('',#17521,2.91746266896347) ;
#4476=CIRCLE('',#17523,2.91746266896347) ;
#4477=CIRCLE('',#17524,2.91746266896347) ;
#4478=CIRCLE('',#17526,2.91746266896347) ;
#4479=CIRCLE('',#17527,2.91746266896347) ;
#4480=CIRCLE('',#17529,2.91746266896347) ;
#4481=CIRCLE('',#17530,2.91746266896347) ;
#4482=CIRCLE('',#17532,2.91746266896347) ;
#4483=CIRCLE('',#17533,2.91746266896347) ;
#4484=CIRCLE('',#17535,2.91746266896347) ;
#4485=CIRCLE('',#17536,2.91746266896347) ;
#4486=CIRCLE('',#17538,2.91746266896347) ;
#4487=CIRCLE('',#17539,2.91746266896347) ;
#4488=CIRCLE('',#17541,2.91746266896347) ;
#4489=CIRCLE('',#17542,2.91746266896347) ;
#4490=CIRCLE('',#17544,2.91746266896347) ;
#4491=CIRCLE('',#17545,2.91746266896347) ;
#4492=CIRCLE('',#17547,2.91746266896347) ;
#4493=CIRCLE('',#17548,2.91746266896347) ;
#4494=CIRCLE('',#17550,2.91746266896347) ;
#4495=CIRCLE('',#17551,2.91746266896347) ;
#4496=CIRCLE('',#17553,2.91746266896347) ;
#4497=CIRCLE('',#17554,2.91746266896347) ;
#4498=CIRCLE('',#17556,2.91746266896347) ;
#4499=CIRCLE('',#17557,2.91746266896347) ;
#4500=CIRCLE('',#17559,2.91746266896347) ;
#4501=CIRCLE('',#17560,2.91746266896347) ;
#4502=CIRCLE('',#17562,2.91746266896347) ;
#4503=CIRCLE('',#17563,2.91746266896347) ;
#4504=CIRCLE('',#17565,2.91746266896347) ;
#4505=CIRCLE('',#17566,2.91746266896347) ;
#4506=CIRCLE('',#17568,2.91746266896347) ;
#4507=CIRCLE('',#17569,2.91746266896347) ;
#4508=CIRCLE('',#17571,2.91746266896347) ;
#4509=CIRCLE('',#17572,2.91746266896347) ;
#4510=CIRCLE('',#17574,2.91746266896347) ;
#4511=CIRCLE('',#17575,2.91746266896347) ;
#4512=CIRCLE('',#17577,2.91746266896347) ;
#4513=CIRCLE('',#17578,2.91746266896347) ;
#4514=CIRCLE('',#17580,2.91746266896347) ;
#4515=CIRCLE('',#17581,2.91746266896347) ;
#4516=CIRCLE('',#17583,2.91746266896347) ;
#4517=CIRCLE('',#17584,2.91746266896347) ;
#4518=CIRCLE('',#17586,2.91746266896347) ;
#4519=CIRCLE('',#17587,2.91746266896347) ;
#4520=CIRCLE('',#17589,2.91746266896347) ;
#4521=CIRCLE('',#17590,2.91746266896347) ;
#4522=CIRCLE('',#17592,2.91746266896347) ;
#4523=CIRCLE('',#17593,2.91746266896347) ;
#4524=CIRCLE('',#17596,2.91746266896347) ;
#4525=CIRCLE('',#17597,2.91746266896347) ;
#4526=CIRCLE('',#17600,3.17084870199964) ;
#4527=CIRCLE('',#17601,3.17084870199964) ;
#4528=CIRCLE('',#17603,3.17084870199964) ;
#4529=CIRCLE('',#17604,3.17084870199964) ;
#4530=CIRCLE('',#17607,3.17084870199964) ;
#4531=CIRCLE('',#17608,3.17084870199964) ;
#4532=CIRCLE('',#17610,3.17084870199964) ;
#4533=CIRCLE('',#17611,3.17084870199964) ;
#4534=CIRCLE('',#17614,3.17084870199964) ;
#4535=CIRCLE('',#17615,3.17084870199964) ;
#4536=CIRCLE('',#17617,3.17084870199964) ;
#4537=CIRCLE('',#17618,3.17084870199964) ;
#4538=CIRCLE('',#17621,3.17084870199964) ;
#4539=CIRCLE('',#17622,3.17084870199964) ;
#4540=CIRCLE('',#17624,3.17084870199964) ;
#4541=CIRCLE('',#17625,3.17084870199964) ;
#4542=CIRCLE('',#17628,3.17084870199964) ;
#4543=CIRCLE('',#17629,3.17084870199964) ;
#4544=CIRCLE('',#17631,3.17084870199964) ;
#4545=CIRCLE('',#17632,3.17084870199964) ;
#4546=CIRCLE('',#17635,3.17084870199964) ;
#4547=CIRCLE('',#17636,3.17084870199964) ;
#4548=CIRCLE('',#17638,3.17084870199964) ;
#4549=CIRCLE('',#17639,3.17084870199964) ;
#4550=CIRCLE('',#17642,3.17084870199964) ;
#4551=CIRCLE('',#17643,3.17084870199964) ;
#4552=CIRCLE('',#17645,3.17084870199964) ;
#4553=CIRCLE('',#17646,3.17084870199964) ;
#4554=CIRCLE('',#17649,3.17084870199964) ;
#4555=CIRCLE('',#17650,3.17084870199964) ;
#4556=CIRCLE('',#17652,3.17084870199964) ;
#4557=CIRCLE('',#17653,3.17084870199964) ;
#4558=CIRCLE('',#17656,3.17084870199964) ;
#4559=CIRCLE('',#17657,3.17084870199964) ;
#4560=CIRCLE('',#17659,3.17084870199964) ;
#4561=CIRCLE('',#17660,3.17084870199964) ;
#4562=CIRCLE('',#17663,3.17084870199964) ;
#4563=CIRCLE('',#17664,3.17084870199964) ;
#4564=CIRCLE('',#17666,3.17084870199964) ;
#4565=CIRCLE('',#17667,3.17084870199964) ;
#4566=CIRCLE('',#17670,3.17084870199964) ;
#4567=CIRCLE('',#17671,3.17084870199964) ;
#4568=CIRCLE('',#17673,3.17084870199964) ;
#4569=CIRCLE('',#17674,3.17084870199964) ;
#4570=CIRCLE('',#17677,3.17084870199964) ;
#4571=CIRCLE('',#17678,3.17084870199964) ;
#4572=CIRCLE('',#17680,3.17084870199964) ;
#4573=CIRCLE('',#17681,3.17084870199964) ;
#4574=CIRCLE('',#17684,3.17084870199964) ;
#4575=CIRCLE('',#17685,3.17084870199964) ;
#4576=CIRCLE('',#17687,3.17084870199964) ;
#4577=CIRCLE('',#17688,3.17084870199964) ;
#4578=CIRCLE('',#17691,3.17084870199964) ;
#4579=CIRCLE('',#17692,3.17084870199964) ;
#4580=CIRCLE('',#17694,3.17084870199964) ;
#4581=CIRCLE('',#17695,3.17084870199964) ;
#4582=CIRCLE('',#17698,3.17084870199964) ;
#4583=CIRCLE('',#17699,3.17084870199964) ;
#4584=CIRCLE('',#17701,3.17084870199964) ;
#4585=CIRCLE('',#17702,3.17084870199964) ;
#4586=CIRCLE('',#17705,3.17084870199964) ;
#4587=CIRCLE('',#17706,3.17084870199964) ;
#4588=CIRCLE('',#17708,3.17084870199964) ;
#4589=CIRCLE('',#17709,3.17084870199964) ;
#4590=CIRCLE('',#17712,3.17084870199964) ;
#4591=CIRCLE('',#17713,3.17084870199964) ;
#4592=CIRCLE('',#17715,3.17084870199964) ;
#4593=CIRCLE('',#17716,3.17084870199964) ;
#4594=CIRCLE('',#17719,3.17084870199964) ;
#4595=CIRCLE('',#17720,3.17084870199964) ;
#4596=CIRCLE('',#17722,3.17084870199964) ;
#4597=CIRCLE('',#17723,3.17084870199964) ;
#4598=CIRCLE('',#17726,3.17084870199964) ;
#4599=CIRCLE('',#17727,3.17084870199964) ;
#4600=CIRCLE('',#17729,3.17084870199964) ;
#4601=CIRCLE('',#17730,3.17084870199964) ;
#4602=CIRCLE('',#17733,3.17084870199964) ;
#4603=CIRCLE('',#17734,3.17084870199964) ;
#4604=CIRCLE('',#17736,3.17084870199964) ;
#4605=CIRCLE('',#17737,3.17084870199964) ;
#4606=CIRCLE('',#17740,3.17084870199964) ;
#4607=CIRCLE('',#17741,3.17084870199964) ;
#4608=CIRCLE('',#17743,3.17084870199964) ;
#4609=CIRCLE('',#17744,3.17084870199964) ;
#4610=CIRCLE('',#17747,3.17084870199964) ;
#4611=CIRCLE('',#17748,3.17084870199964) ;
#4612=CIRCLE('',#17750,3.17084870199964) ;
#4613=CIRCLE('',#17751,3.17084870199964) ;
#4614=CIRCLE('',#17754,3.17084870199964) ;
#4615=CIRCLE('',#17755,3.17084870199964) ;
#4616=CIRCLE('',#17757,3.17084870199964) ;
#4617=CIRCLE('',#17758,3.17084870199964) ;
#4618=CIRCLE('',#17761,3.17084870199964) ;
#4619=CIRCLE('',#17762,3.17084870199964) ;
#4620=CIRCLE('',#17764,3.17084870199964) ;
#4621=CIRCLE('',#17765,3.17084870199964) ;
#4622=CIRCLE('',#17768,3.17084870199964) ;
#4623=CIRCLE('',#17769,3.17084870199964) ;
#4624=CIRCLE('',#17771,3.17084870199964) ;
#4625=CIRCLE('',#17772,3.17084870199964) ;
#4626=CIRCLE('',#17775,3.17084870199964) ;
#4627=CIRCLE('',#17776,3.17084870199964) ;
#4628=CIRCLE('',#17778,3.17084870199964) ;
#4629=CIRCLE('',#17779,3.17084870199964) ;
#4630=CIRCLE('',#17782,3.17084870199964) ;
#4631=CIRCLE('',#17783,3.17084870199964) ;
#4632=CIRCLE('',#17785,3.17084870199964) ;
#4633=CIRCLE('',#17786,3.17084870199964) ;
#4634=CIRCLE('',#17789,3.17084870199964) ;
#4635=CIRCLE('',#17790,3.17084870199964) ;
#4636=CIRCLE('',#17792,3.17084870199964) ;
#4637=CIRCLE('',#17793,3.17084870199964) ;
#4638=CIRCLE('',#17796,3.17084870199964) ;
#4639=CIRCLE('',#17797,3.17084870199964) ;
#4640=CIRCLE('',#17799,3.17084870199964) ;
#4641=CIRCLE('',#17800,3.17084870199964) ;
#5254=LINE('',#53882,#5910) ;
#5255=LINE('',#56612,#5911) ;
#5256=LINE('',#57803,#5912) ;
#5257=LINE('',#57807,#5913) ;
#5258=LINE('',#57809,#5914) ;
#5259=LINE('',#57813,#5915) ;
#5260=LINE('',#57815,#5916) ;
#5261=LINE('',#57819,#5917) ;
#5262=LINE('',#57821,#5918) ;
#5263=LINE('',#57825,#5919) ;
#5264=LINE('',#57827,#5920) ;
#5265=LINE('',#57831,#5921) ;
#5266=LINE('',#57833,#5922) ;
#5267=LINE('',#57837,#5923) ;
#5268=LINE('',#57839,#5924) ;
#5269=LINE('',#57843,#5925) ;
#5270=LINE('',#57845,#5926) ;
#5271=LINE('',#57849,#5927) ;
#5272=LINE('',#57851,#5928) ;
#5273=LINE('',#57855,#5929) ;
#5274=LINE('',#57857,#5930) ;
#5275=LINE('',#57861,#5931) ;
#5276=LINE('',#57863,#5932) ;
#5277=LINE('',#57867,#5933) ;
#5278=LINE('',#57869,#5934) ;
#5279=LINE('',#57873,#5935) ;
#5280=LINE('',#57875,#5936) ;
#5281=LINE('',#57879,#5937) ;
#5282=LINE('',#57881,#5938) ;
#5283=LINE('',#57885,#5939) ;
#5284=LINE('',#57887,#5940) ;
#5285=LINE('',#57891,#5941) ;
#5286=LINE('',#57893,#5942) ;
#5287=LINE('',#57897,#5943) ;
#5288=LINE('',#57899,#5944) ;
#5289=LINE('',#57903,#5945) ;
#5290=LINE('',#57905,#5946) ;
#5291=LINE('',#57909,#5947) ;
#5292=LINE('',#57911,#5948) ;
#5293=LINE('',#57915,#5949) ;
#5294=LINE('',#57917,#5950) ;
#5295=LINE('',#57921,#5951) ;
#5296=LINE('',#57923,#5952) ;
#5297=LINE('',#57927,#5953) ;
#5298=LINE('',#57929,#5954) ;
#5299=LINE('',#57933,#5955) ;
#5300=LINE('',#57935,#5956) ;
#5301=LINE('',#57939,#5957) ;
#5302=LINE('',#57941,#5958) ;
#5303=LINE('',#57945,#5959) ;
#5304=LINE('',#57947,#5960) ;
#5305=LINE('',#57951,#5961) ;
#5306=LINE('',#57953,#5962) ;
#5307=LINE('',#57957,#5963) ;
#5308=LINE('',#57959,#5964) ;
#5309=LINE('',#57963,#5965) ;
#5310=LINE('',#57965,#5966) ;
#5311=LINE('',#57969,#5967) ;
#5312=LINE('',#57971,#5968) ;
#5313=LINE('',#57975,#5969) ;
#5314=LINE('',#57977,#5970) ;
#5315=LINE('',#57983,#5971) ;
#5316=LINE('',#63291,#5972) ;
#5317=LINE('',#63313,#5973) ;
#5318=LINE('',#63320,#5974) ;
#5319=LINE('',#63413,#5975) ;
#5910=VECTOR('',#21666,28.523658167371) ;
#5911=VECTOR('',#21787,26.6311750163962) ;
#5912=VECTOR('',#21908,10.) ;
#5913=VECTOR('',#21913,10.) ;
#5914=VECTOR('',#21914,9.99999999999998) ;
#5915=VECTOR('',#21919,10.) ;
#5916=VECTOR('',#21920,10.) ;
#5917=VECTOR('',#21925,10.) ;
#5918=VECTOR('',#21926,10.) ;
#5919=VECTOR('',#21931,10.) ;
#5920=VECTOR('',#21932,10.) ;
#5921=VECTOR('',#21937,10.) ;
#5922=VECTOR('',#21938,10.) ;
#5923=VECTOR('',#21943,10.) ;
#5924=VECTOR('',#21944,9.99999999999999) ;
#5925=VECTOR('',#21949,10.) ;
#5926=VECTOR('',#21950,10.) ;
#5927=VECTOR('',#21955,10.) ;
#5928=VECTOR('',#21956,10.) ;
#5929=VECTOR('',#21961,10.) ;
#5930=VECTOR('',#21962,10.) ;
#5931=VECTOR('',#21967,10.) ;
#5932=VECTOR('',#21968,10.) ;
#5933=VECTOR('',#21973,10.) ;
#5934=VECTOR('',#21974,10.) ;
#5935=VECTOR('',#21979,10.) ;
#5936=VECTOR('',#21980,10.) ;
#5937=VECTOR('',#21985,10.) ;
#5938=VECTOR('',#21986,10.) ;
#5939=VECTOR('',#21991,10.) ;
#5940=VECTOR('',#21992,10.) ;
#5941=VECTOR('',#21997,10.) ;
#5942=VECTOR('',#21998,10.) ;
#5943=VECTOR('',#22003,9.99999999999998) ;
#5944=VECTOR('',#22004,10.) ;
#5945=VECTOR('',#22009,10.) ;
#5946=VECTOR('',#22010,10.) ;
#5947=VECTOR('',#22015,10.) ;
#5948=VECTOR('',#22016,10.) ;
#5949=VECTOR('',#22021,10.) ;
#5950=VECTOR('',#22022,10.) ;
#5951=VECTOR('',#22027,10.) ;
#5952=VECTOR('',#22028,10.) ;
#5953=VECTOR('',#22033,10.) ;
#5954=VECTOR('',#22034,10.) ;
#5955=VECTOR('',#22039,10.) ;
#5956=VECTOR('',#22040,10.) ;
#5957=VECTOR('',#22045,10.) ;
#5958=VECTOR('',#22046,10.) ;
#5959=VECTOR('',#22051,10.) ;
#5960=VECTOR('',#22052,10.) ;
#5961=VECTOR('',#22057,10.) ;
#5962=VECTOR('',#22058,10.) ;
#5963=VECTOR('',#22063,10.) ;
#5964=VECTOR('',#22064,10.) ;
#5965=VECTOR('',#22069,10.) ;
#5966=VECTOR('',#22070,10.) ;
#5967=VECTOR('',#22075,10.) ;
#5968=VECTOR('',#22076,10.) ;
#5969=VECTOR('',#22081,10.) ;
#5970=VECTOR('',#22082,29.3077933083081) ;
#5971=VECTOR('',#22089,32.4669335366504) ;
#5972=VECTOR('',#22154,27.082990178354) ;
#5973=VECTOR('',#22183,22.5) ;
#5974=VECTOR('',#22194,37.5) ;
#5975=VECTOR('',#22379,26.3029085923563) ;
#6985=VERTEX_POINT('',#53879) ;
#6986=VERTEX_POINT('',#53881) ;
#6987=VERTEX_POINT('',#53883) ;
#6988=VERTEX_POINT('',#53885) ;
#6989=VERTEX_POINT('',#53926) ;
#6990=VERTEX_POINT('',#53930) ;
#6991=VERTEX_POINT('',#53932) ;
#6992=VERTEX_POINT('',#53936) ;
#6993=VERTEX_POINT('',#53977) ;
#6994=VERTEX_POINT('',#53979) ;
#6995=VERTEX_POINT('',#54020) ;
#6996=VERTEX_POINT('',#54024) ;
#6997=VERTEX_POINT('',#54026) ;
#6998=VERTEX_POINT('',#54030) ;
#6999=VERTEX_POINT('',#54071) ;
#7000=VERTEX_POINT('',#54073) ;
#7001=VERTEX_POINT('',#54114) ;
#7002=VERTEX_POINT('',#54118) ;
#7003=VERTEX_POINT('',#54120) ;
#7004=VERTEX_POINT('',#54124) ;
#7005=VERTEX_POINT('',#54165) ;
#7006=VERTEX_POINT('',#54167) ;
#7007=VERTEX_POINT('',#54208) ;
#7008=VERTEX_POINT('',#54212) ;
#7009=VERTEX_POINT('',#54214) ;
#7010=VERTEX_POINT('',#54218) ;
#7011=VERTEX_POINT('',#54259) ;
#7012=VERTEX_POINT('',#54261) ;
#7013=VERTEX_POINT('',#54302) ;
#7014=VERTEX_POINT('',#54306) ;
#7015=VERTEX_POINT('',#54308) ;
#7016=VERTEX_POINT('',#54312) ;
#7017=VERTEX_POINT('',#54353) ;
#7018=VERTEX_POINT('',#54355) ;
#7019=VERTEX_POINT('',#54396) ;
#7020=VERTEX_POINT('',#54400) ;
#7021=VERTEX_POINT('',#54402) ;
#7022=VERTEX_POINT('',#54406) ;
#7023=VERTEX_POINT('',#54447) ;
#7024=VERTEX_POINT('',#54449) ;
#7025=VERTEX_POINT('',#54490) ;
#7026=VERTEX_POINT('',#54494) ;
#7027=VERTEX_POINT('',#54496) ;
#7028=VERTEX_POINT('',#54500) ;
#7029=VERTEX_POINT('',#54541) ;
#7030=VERTEX_POINT('',#54543) ;
#7031=VERTEX_POINT('',#54584) ;
#7032=VERTEX_POINT('',#54588) ;
#7033=VERTEX_POINT('',#54590) ;
#7034=VERTEX_POINT('',#54594) ;
#7035=VERTEX_POINT('',#54635) ;
#7036=VERTEX_POINT('',#54637) ;
#7037=VERTEX_POINT('',#54678) ;
#7038=VERTEX_POINT('',#54682) ;
#7039=VERTEX_POINT('',#54684) ;
#7040=VERTEX_POINT('',#54688) ;
#7041=VERTEX_POINT('',#54729) ;
#7042=VERTEX_POINT('',#54731) ;
#7043=VERTEX_POINT('',#54772) ;
#7044=VERTEX_POINT('',#54776) ;
#7045=VERTEX_POINT('',#54778) ;
#7046=VERTEX_POINT('',#54782) ;
#7047=VERTEX_POINT('',#54823) ;
#7048=VERTEX_POINT('',#54825) ;
#7049=VERTEX_POINT('',#54866) ;
#7050=VERTEX_POINT('',#54870) ;
#7051=VERTEX_POINT('',#54872) ;
#7052=VERTEX_POINT('',#54876) ;
#7053=VERTEX_POINT('',#54917) ;
#7054=VERTEX_POINT('',#54919) ;
#7055=VERTEX_POINT('',#54960) ;
#7056=VERTEX_POINT('',#54964) ;
#7057=VERTEX_POINT('',#54966) ;
#7058=VERTEX_POINT('',#54970) ;
#7059=VERTEX_POINT('',#55011) ;
#7060=VERTEX_POINT('',#55013) ;
#7061=VERTEX_POINT('',#55054) ;
#7062=VERTEX_POINT('',#55058) ;
#7063=VERTEX_POINT('',#55060) ;
#7064=VERTEX_POINT('',#55064) ;
#7065=VERTEX_POINT('',#55105) ;
#7066=VERTEX_POINT('',#55107) ;
#7067=VERTEX_POINT('',#55148) ;
#7068=VERTEX_POINT('',#55152) ;
#7069=VERTEX_POINT('',#55154) ;
#7070=VERTEX_POINT('',#55158) ;
#7071=VERTEX_POINT('',#55199) ;
#7072=VERTEX_POINT('',#55201) ;
#7073=VERTEX_POINT('',#55242) ;
#7074=VERTEX_POINT('',#55246) ;
#7075=VERTEX_POINT('',#55248) ;
#7076=VERTEX_POINT('',#55252) ;
#7077=VERTEX_POINT('',#55293) ;
#7078=VERTEX_POINT('',#55295) ;
#7079=VERTEX_POINT('',#55336) ;
#7080=VERTEX_POINT('',#55340) ;
#7081=VERTEX_POINT('',#55342) ;
#7082=VERTEX_POINT('',#55346) ;
#7083=VERTEX_POINT('',#55387) ;
#7084=VERTEX_POINT('',#55389) ;
#7085=VERTEX_POINT('',#55430) ;
#7086=VERTEX_POINT('',#55434) ;
#7087=VERTEX_POINT('',#55436) ;
#7088=VERTEX_POINT('',#55440) ;
#7089=VERTEX_POINT('',#55481) ;
#7090=VERTEX_POINT('',#55483) ;
#7091=VERTEX_POINT('',#55524) ;
#7092=VERTEX_POINT('',#55528) ;
#7093=VERTEX_POINT('',#55530) ;
#7094=VERTEX_POINT('',#55534) ;
#7095=VERTEX_POINT('',#55575) ;
#7096=VERTEX_POINT('',#55577) ;
#7097=VERTEX_POINT('',#55618) ;
#7098=VERTEX_POINT('',#55622) ;
#7099=VERTEX_POINT('',#55624) ;
#7100=VERTEX_POINT('',#55628) ;
#7101=VERTEX_POINT('',#55669) ;
#7102=VERTEX_POINT('',#55671) ;
#7103=VERTEX_POINT('',#55712) ;
#7104=VERTEX_POINT('',#55716) ;
#7105=VERTEX_POINT('',#55718) ;
#7106=VERTEX_POINT('',#55722) ;
#7107=VERTEX_POINT('',#55763) ;
#7108=VERTEX_POINT('',#55765) ;
#7109=VERTEX_POINT('',#55806) ;
#7110=VERTEX_POINT('',#55810) ;
#7111=VERTEX_POINT('',#55812) ;
#7112=VERTEX_POINT('',#55816) ;
#7113=VERTEX_POINT('',#55857) ;
#7114=VERTEX_POINT('',#55859) ;
#7115=VERTEX_POINT('',#55900) ;
#7116=VERTEX_POINT('',#55904) ;
#7117=VERTEX_POINT('',#55906) ;
#7118=VERTEX_POINT('',#55910) ;
#7119=VERTEX_POINT('',#55951) ;
#7120=VERTEX_POINT('',#55953) ;
#7121=VERTEX_POINT('',#55994) ;
#7122=VERTEX_POINT('',#55998) ;
#7123=VERTEX_POINT('',#56000) ;
#7124=VERTEX_POINT('',#56004) ;
#7125=VERTEX_POINT('',#56045) ;
#7126=VERTEX_POINT('',#56047) ;
#7127=VERTEX_POINT('',#56088) ;
#7128=VERTEX_POINT('',#56092) ;
#7129=VERTEX_POINT('',#56094) ;
#7130=VERTEX_POINT('',#56098) ;
#7131=VERTEX_POINT('',#56139) ;
#7132=VERTEX_POINT('',#56141) ;
#7133=VERTEX_POINT('',#56182) ;
#7134=VERTEX_POINT('',#56186) ;
#7135=VERTEX_POINT('',#56188) ;
#7136=VERTEX_POINT('',#56192) ;
#7137=VERTEX_POINT('',#56233) ;
#7138=VERTEX_POINT('',#56235) ;
#7139=VERTEX_POINT('',#56276) ;
#7140=VERTEX_POINT('',#56280) ;
#7141=VERTEX_POINT('',#56282) ;
#7142=VERTEX_POINT('',#56286) ;
#7143=VERTEX_POINT('',#56327) ;
#7144=VERTEX_POINT('',#56329) ;
#7145=VERTEX_POINT('',#56370) ;
#7146=VERTEX_POINT('',#56374) ;
#7147=VERTEX_POINT('',#56376) ;
#7148=VERTEX_POINT('',#56380) ;
#7149=VERTEX_POINT('',#56421) ;
#7150=VERTEX_POINT('',#56423) ;
#7151=VERTEX_POINT('',#56464) ;
#7152=VERTEX_POINT('',#56468) ;
#7153=VERTEX_POINT('',#56470) ;
#7154=VERTEX_POINT('',#56474) ;
#7155=VERTEX_POINT('',#56515) ;
#7156=VERTEX_POINT('',#56517) ;
#7157=VERTEX_POINT('',#56558) ;
#7158=VERTEX_POINT('',#56562) ;
#7159=VERTEX_POINT('',#56564) ;
#7160=VERTEX_POINT('',#56568) ;
#7161=VERTEX_POINT('',#56611) ;
#7162=VERTEX_POINT('',#56613) ;
#7163=VERTEX_POINT('',#56615) ;
#7164=VERTEX_POINT('',#56638) ;
#7165=VERTEX_POINT('',#56650) ;
#7166=VERTEX_POINT('',#56652) ;
#7167=VERTEX_POINT('',#56675) ;
#7168=VERTEX_POINT('',#56689) ;
#7169=VERTEX_POINT('',#56691) ;
#7170=VERTEX_POINT('',#56714) ;
#7171=VERTEX_POINT('',#56726) ;
#7172=VERTEX_POINT('',#56728) ;
#7173=VERTEX_POINT('',#56751) ;
#7174=VERTEX_POINT('',#56765) ;
#7175=VERTEX_POINT('',#56767) ;
#7176=VERTEX_POINT('',#56790) ;
#7177=VERTEX_POINT('',#56802) ;
#7178=VERTEX_POINT('',#56804) ;
#7179=VERTEX_POINT('',#56827) ;
#7180=VERTEX_POINT('',#56857) ;
#7181=VERTEX_POINT('',#56859) ;
#7182=VERTEX_POINT('',#56882) ;
#7183=VERTEX_POINT('',#56894) ;
#7184=VERTEX_POINT('',#56896) ;
#7185=VERTEX_POINT('',#56919) ;
#7186=VERTEX_POINT('',#56933) ;
#7187=VERTEX_POINT('',#56935) ;
#7188=VERTEX_POINT('',#56937) ;
#7189=VERTEX_POINT('',#56960) ;
#7190=VERTEX_POINT('',#56972) ;
#7191=VERTEX_POINT('',#56974) ;
#7192=VERTEX_POINT('',#56997) ;
#7193=VERTEX_POINT('',#57015) ;
#7194=VERTEX_POINT('',#57017) ;
#7195=VERTEX_POINT('',#57040) ;
#7196=VERTEX_POINT('',#57054) ;
#7197=VERTEX_POINT('',#57056) ;
#7198=VERTEX_POINT('',#57079) ;
#7199=VERTEX_POINT('',#57091) ;
#7200=VERTEX_POINT('',#57093) ;
#7201=VERTEX_POINT('',#57095) ;
#7202=VERTEX_POINT('',#57118) ;
#7203=VERTEX_POINT('',#57132) ;
#7204=VERTEX_POINT('',#57134) ;
#7205=VERTEX_POINT('',#57161) ;
#7206=VERTEX_POINT('',#57183) ;
#7207=VERTEX_POINT('',#57185) ;
#7208=VERTEX_POINT('',#57208) ;
#7209=VERTEX_POINT('',#57220) ;
#7210=VERTEX_POINT('',#57222) ;
#7211=VERTEX_POINT('',#57245) ;
#7212=VERTEX_POINT('',#57259) ;
#7213=VERTEX_POINT('',#57261) ;
#7214=VERTEX_POINT('',#57284) ;
#7215=VERTEX_POINT('',#57298) ;
#7216=VERTEX_POINT('',#57300) ;
#7217=VERTEX_POINT('',#57323) ;
#7218=VERTEX_POINT('',#57343) ;
#7219=VERTEX_POINT('',#57345) ;
#7220=VERTEX_POINT('',#57374) ;
#7221=VERTEX_POINT('',#57394) ;
#7222=VERTEX_POINT('',#57396) ;
#7223=VERTEX_POINT('',#57419) ;
#7224=VERTEX_POINT('',#57433) ;
#7225=VERTEX_POINT('',#57435) ;
#7226=VERTEX_POINT('',#57458) ;
#7227=VERTEX_POINT('',#57470) ;
#7228=VERTEX_POINT('',#57472) ;
#7229=VERTEX_POINT('',#57495) ;
#7230=VERTEX_POINT('',#57509) ;
#7231=VERTEX_POINT('',#57511) ;
#7232=VERTEX_POINT('',#57534) ;
#7233=VERTEX_POINT('',#57546) ;
#7234=VERTEX_POINT('',#57548) ;
#7235=VERTEX_POINT('',#57571) ;
#7236=VERTEX_POINT('',#57585) ;
#7237=VERTEX_POINT('',#57587) ;
#7238=VERTEX_POINT('',#57610) ;
#7239=VERTEX_POINT('',#57622) ;
#7240=VERTEX_POINT('',#57624) ;
#7241=VERTEX_POINT('',#57647) ;
#7242=VERTEX_POINT('',#57661) ;
#7243=VERTEX_POINT('',#57663) ;
#7244=VERTEX_POINT('',#57686) ;
#7245=VERTEX_POINT('',#57701) ;
#7246=VERTEX_POINT('',#57728) ;
#7247=VERTEX_POINT('',#57750) ;
#7248=VERTEX_POINT('',#57779) ;
#7249=VERTEX_POINT('',#57802) ;
#7250=VERTEX_POINT('',#57805) ;
#7251=VERTEX_POINT('',#57808) ;
#7252=VERTEX_POINT('',#57811) ;
#7253=VERTEX_POINT('',#57814) ;
#7254=VERTEX_POINT('',#57817) ;
#7255=VERTEX_POINT('',#57820) ;
#7256=VERTEX_POINT('',#57823) ;
#7257=VERTEX_POINT('',#57826) ;
#7258=VERTEX_POINT('',#57829) ;
#7259=VERTEX_POINT('',#57832) ;
#7260=VERTEX_POINT('',#57835) ;
#7261=VERTEX_POINT('',#57838) ;
#7262=VERTEX_POINT('',#57841) ;
#7263=VERTEX_POINT('',#57844) ;
#7264=VERTEX_POINT('',#57847) ;
#7265=VERTEX_POINT('',#57850) ;
#7266=VERTEX_POINT('',#57853) ;
#7267=VERTEX_POINT('',#57856) ;
#7268=VERTEX_POINT('',#57859) ;
#7269=VERTEX_POINT('',#57862) ;
#7270=VERTEX_POINT('',#57865) ;
#7271=VERTEX_POINT('',#57868) ;
#7272=VERTEX_POINT('',#57871) ;
#7273=VERTEX_POINT('',#57874) ;
#7274=VERTEX_POINT('',#57877) ;
#7275=VERTEX_POINT('',#57880) ;
#7276=VERTEX_POINT('',#57883) ;
#7277=VERTEX_POINT('',#57886) ;
#7278=VERTEX_POINT('',#57889) ;
#7279=VERTEX_POINT('',#57892) ;
#7280=VERTEX_POINT('',#57895) ;
#7281=VERTEX_POINT('',#57898) ;
#7282=VERTEX_POINT('',#57901) ;
#7283=VERTEX_POINT('',#57904) ;
#7284=VERTEX_POINT('',#57907) ;
#7285=VERTEX_POINT('',#57910) ;
#7286=VERTEX_POINT('',#57913) ;
#7287=VERTEX_POINT('',#57916) ;
#7288=VERTEX_POINT('',#57919) ;
#7289=VERTEX_POINT('',#57922) ;
#7290=VERTEX_POINT('',#57925) ;
#7291=VERTEX_POINT('',#57928) ;
#7292=VERTEX_POINT('',#57931) ;
#7293=VERTEX_POINT('',#57934) ;
#7294=VERTEX_POINT('',#57937) ;
#7295=VERTEX_POINT('',#57940) ;
#7296=VERTEX_POINT('',#57943) ;
#7297=VERTEX_POINT('',#57946) ;
#7298=VERTEX_POINT('',#57949) ;
#7299=VERTEX_POINT('',#57952) ;
#7300=VERTEX_POINT('',#57955) ;
#7301=VERTEX_POINT('',#57958) ;
#7302=VERTEX_POINT('',#57961) ;
#7303=VERTEX_POINT('',#57964) ;
#7304=VERTEX_POINT('',#57967) ;
#7305=VERTEX_POINT('',#57970) ;
#7306=VERTEX_POINT('',#57973) ;
#7307=VERTEX_POINT('',#57976) ;
#7308=VERTEX_POINT('',#57980) ;
#7309=VERTEX_POINT('',#57982) ;
#7310=VERTEX_POINT('',#57985) ;
#7311=VERTEX_POINT('',#57986) ;
#7312=VERTEX_POINT('',#58077) ;
#7313=VERTEX_POINT('',#58169) ;
#7314=VERTEX_POINT('',#58170) ;
#7315=VERTEX_POINT('',#58172) ;
#7316=VERTEX_POINT('',#58351) ;
#7317=VERTEX_POINT('',#58352) ;
#7318=VERTEX_POINT('',#58354) ;
#7319=VERTEX_POINT('',#58533) ;
#7320=VERTEX_POINT('',#58534) ;
#7321=VERTEX_POINT('',#58536) ;
#7322=VERTEX_POINT('',#58716) ;
#7323=VERTEX_POINT('',#58717) ;
#7324=VERTEX_POINT('',#58719) ;
#7325=VERTEX_POINT('',#58900) ;
#7326=VERTEX_POINT('',#58901) ;
#7327=VERTEX_POINT('',#58903) ;
#7328=VERTEX_POINT('',#59082) ;
#7329=VERTEX_POINT('',#59083) ;
#7330=VERTEX_POINT('',#59085) ;
#7331=VERTEX_POINT('',#59264) ;
#7332=VERTEX_POINT('',#59265) ;
#7333=VERTEX_POINT('',#59267) ;
#7334=VERTEX_POINT('',#59448) ;
#7335=VERTEX_POINT('',#59449) ;
#7336=VERTEX_POINT('',#59451) ;
#7337=VERTEX_POINT('',#59631) ;
#7338=VERTEX_POINT('',#59632) ;
#7339=VERTEX_POINT('',#59634) ;
#7340=VERTEX_POINT('',#59813) ;
#7341=VERTEX_POINT('',#59814) ;
#7342=VERTEX_POINT('',#59816) ;
#7343=VERTEX_POINT('',#59996) ;
#7344=VERTEX_POINT('',#59997) ;
#7345=VERTEX_POINT('',#59999) ;
#7346=VERTEX_POINT('',#60180) ;
#7347=VERTEX_POINT('',#60181) ;
#7348=VERTEX_POINT('',#60183) ;
#7349=VERTEX_POINT('',#60362) ;
#7350=VERTEX_POINT('',#60363) ;
#7351=VERTEX_POINT('',#60365) ;
#7352=VERTEX_POINT('',#60544) ;
#7353=VERTEX_POINT('',#60545) ;
#7354=VERTEX_POINT('',#60547) ;
#7355=VERTEX_POINT('',#60728) ;
#7356=VERTEX_POINT('',#60729) ;
#7357=VERTEX_POINT('',#60731) ;
#7358=VERTEX_POINT('',#60910) ;
#7359=VERTEX_POINT('',#60911) ;
#7360=VERTEX_POINT('',#60913) ;
#7361=VERTEX_POINT('',#61092) ;
#7362=VERTEX_POINT('',#61093) ;
#7363=VERTEX_POINT('',#61095) ;
#7364=VERTEX_POINT('',#61275) ;
#7365=VERTEX_POINT('',#61276) ;
#7366=VERTEX_POINT('',#61278) ;
#7367=VERTEX_POINT('',#61459) ;
#7368=VERTEX_POINT('',#61460) ;
#7369=VERTEX_POINT('',#61462) ;
#7370=VERTEX_POINT('',#61641) ;
#7371=VERTEX_POINT('',#61642) ;
#7372=VERTEX_POINT('',#61644) ;
#7373=VERTEX_POINT('',#61823) ;
#7374=VERTEX_POINT('',#61824) ;
#7375=VERTEX_POINT('',#61826) ;
#7376=VERTEX_POINT('',#62007) ;
#7377=VERTEX_POINT('',#62008) ;
#7378=VERTEX_POINT('',#62010) ;
#7379=VERTEX_POINT('',#62190) ;
#7380=VERTEX_POINT('',#62191) ;
#7381=VERTEX_POINT('',#62193) ;
#7382=VERTEX_POINT('',#62372) ;
#7383=VERTEX_POINT('',#62373) ;
#7384=VERTEX_POINT('',#62375) ;
#7385=VERTEX_POINT('',#62555) ;
#7386=VERTEX_POINT('',#62556) ;
#7387=VERTEX_POINT('',#62558) ;
#7388=VERTEX_POINT('',#62739) ;
#7389=VERTEX_POINT('',#62740) ;
#7390=VERTEX_POINT('',#62742) ;
#7391=VERTEX_POINT('',#62921) ;
#7392=VERTEX_POINT('',#62922) ;
#7393=VERTEX_POINT('',#62924) ;
#7394=VERTEX_POINT('',#63103) ;
#7395=VERTEX_POINT('',#63104) ;
#7396=VERTEX_POINT('',#63106) ;
#7397=VERTEX_POINT('',#63288) ;
#7398=VERTEX_POINT('',#63290) ;
#7399=VERTEX_POINT('',#63294) ;
#7400=VERTEX_POINT('',#63296) ;
#7401=VERTEX_POINT('',#63300) ;
#7402=VERTEX_POINT('',#63302) ;
#7403=VERTEX_POINT('',#63306) ;
#7404=VERTEX_POINT('',#63308) ;
#7405=VERTEX_POINT('',#63312) ;
#7406=VERTEX_POINT('',#63316) ;
#9033=EDGE_CURVE('',#6985,#6985,#4361,.T.) ;
#9034=EDGE_CURVE('',#6985,#6986,#5254,.T.) ;
#9035=EDGE_CURVE('',#6986,#6987,#4362,.T.) ;
#9036=EDGE_CURVE('',#6987,#6988,#333,.T.) ;
#9037=EDGE_CURVE('',#6989,#6988,#334,.T.) ;
#9038=EDGE_CURVE('',#6989,#6990,#4363,.T.) ;
#9039=EDGE_CURVE('',#6991,#6990,#335,.T.) ;
#9040=EDGE_CURVE('',#6991,#6992,#336,.T.) ;
#9041=EDGE_CURVE('',#6992,#6993,#4364,.T.) ;
#9042=EDGE_CURVE('',#6993,#6994,#337,.T.) ;
#9043=EDGE_CURVE('',#6995,#6994,#338,.T.) ;
#9044=EDGE_CURVE('',#6995,#6996,#4365,.T.) ;
#9045=EDGE_CURVE('',#6997,#6996,#339,.T.) ;
#9046=EDGE_CURVE('',#6997,#6998,#340,.T.) ;
#9047=EDGE_CURVE('',#6998,#6999,#4366,.T.) ;
#9048=EDGE_CURVE('',#6999,#7000,#341,.T.) ;
#9049=EDGE_CURVE('',#7001,#7000,#342,.T.) ;
#9050=EDGE_CURVE('',#7001,#7002,#4367,.T.) ;
#9051=EDGE_CURVE('',#7003,#7002,#343,.T.) ;
#9052=EDGE_CURVE('',#7003,#7004,#344,.T.) ;
#9053=EDGE_CURVE('',#7004,#7005,#4368,.T.) ;
#9054=EDGE_CURVE('',#7005,#7006,#345,.T.) ;
#9055=EDGE_CURVE('',#7007,#7006,#346,.T.) ;
#9056=EDGE_CURVE('',#7007,#7008,#4369,.T.) ;
#9057=EDGE_CURVE('',#7009,#7008,#347,.T.) ;
#9058=EDGE_CURVE('',#7009,#7010,#348,.T.) ;
#9059=EDGE_CURVE('',#7010,#7011,#4370,.T.) ;
#9060=EDGE_CURVE('',#7011,#7012,#349,.T.) ;
#9061=EDGE_CURVE('',#7013,#7012,#350,.T.) ;
#9062=EDGE_CURVE('',#7013,#7014,#4371,.T.) ;
#9063=EDGE_CURVE('',#7015,#7014,#351,.T.) ;
#9064=EDGE_CURVE('',#7015,#7016,#352,.T.) ;
#9065=EDGE_CURVE('',#7016,#7017,#4372,.T.) ;
#9066=EDGE_CURVE('',#7017,#7018,#353,.T.) ;
#9067=EDGE_CURVE('',#7019,#7018,#354,.T.) ;
#9068=EDGE_CURVE('',#7019,#7020,#4373,.T.) ;
#9069=EDGE_CURVE('',#7021,#7020,#355,.T.) ;
#9070=EDGE_CURVE('',#7021,#7022,#356,.T.) ;
#9071=EDGE_CURVE('',#7022,#7023,#4374,.T.) ;
#9072=EDGE_CURVE('',#7023,#7024,#357,.T.) ;
#9073=EDGE_CURVE('',#7025,#7024,#358,.T.) ;
#9074=EDGE_CURVE('',#7025,#7026,#4375,.T.) ;
#9075=EDGE_CURVE('',#7027,#7026,#359,.T.) ;
#9076=EDGE_CURVE('',#7027,#7028,#360,.T.) ;
#9077=EDGE_CURVE('',#7028,#7029,#4376,.T.) ;
#9078=EDGE_CURVE('',#7029,#7030,#361,.T.) ;
#9079=EDGE_CURVE('',#7031,#7030,#362,.T.) ;
#9080=EDGE_CURVE('',#7031,#7032,#4377,.T.) ;
#9081=EDGE_CURVE('',#7033,#7032,#363,.T.) ;
#9082=EDGE_CURVE('',#7033,#7034,#364,.T.) ;
#9083=EDGE_CURVE('',#7034,#7035,#4378,.T.) ;
#9084=EDGE_CURVE('',#7035,#7036,#365,.T.) ;
#9085=EDGE_CURVE('',#7037,#7036,#366,.T.) ;
#9086=EDGE_CURVE('',#7037,#7038,#4379,.T.) ;
#9087=EDGE_CURVE('',#7039,#7038,#367,.T.) ;
#9088=EDGE_CURVE('',#7039,#7040,#368,.T.) ;
#9089=EDGE_CURVE('',#7040,#7041,#4380,.T.) ;
#9090=EDGE_CURVE('',#7041,#7042,#369,.T.) ;
#9091=EDGE_CURVE('',#7043,#7042,#370,.T.) ;
#9092=EDGE_CURVE('',#7043,#7044,#4381,.T.) ;
#9093=EDGE_CURVE('',#7045,#7044,#371,.T.) ;
#9094=EDGE_CURVE('',#7045,#7046,#372,.T.) ;
#9095=EDGE_CURVE('',#7046,#7047,#4382,.T.) ;
#9096=EDGE_CURVE('',#7047,#7048,#373,.T.) ;
#9097=EDGE_CURVE('',#7049,#7048,#374,.T.) ;
#9098=EDGE_CURVE('',#7049,#7050,#4383,.T.) ;
#9099=EDGE_CURVE('',#7051,#7050,#375,.T.) ;
#9100=EDGE_CURVE('',#7051,#7052,#376,.T.) ;
#9101=EDGE_CURVE('',#7052,#7053,#4384,.T.) ;
#9102=EDGE_CURVE('',#7053,#7054,#377,.T.) ;
#9103=EDGE_CURVE('',#7055,#7054,#378,.T.) ;
#9104=EDGE_CURVE('',#7055,#7056,#4385,.T.) ;
#9105=EDGE_CURVE('',#7057,#7056,#379,.T.) ;
#9106=EDGE_CURVE('',#7057,#7058,#380,.T.) ;
#9107=EDGE_CURVE('',#7058,#7059,#4386,.T.) ;
#9108=EDGE_CURVE('',#7059,#7060,#381,.T.) ;
#9109=EDGE_CURVE('',#7061,#7060,#382,.T.) ;
#9110=EDGE_CURVE('',#7061,#7062,#4387,.T.) ;
#9111=EDGE_CURVE('',#7063,#7062,#383,.T.) ;
#9112=EDGE_CURVE('',#7063,#7064,#384,.T.) ;
#9113=EDGE_CURVE('',#7064,#7065,#4388,.T.) ;
#9114=EDGE_CURVE('',#7065,#7066,#385,.T.) ;
#9115=EDGE_CURVE('',#7067,#7066,#386,.T.) ;
#9116=EDGE_CURVE('',#7067,#7068,#4389,.T.) ;
#9117=EDGE_CURVE('',#7069,#7068,#387,.T.) ;
#9118=EDGE_CURVE('',#7069,#7070,#388,.T.) ;
#9119=EDGE_CURVE('',#7070,#7071,#4390,.T.) ;
#9120=EDGE_CURVE('',#7071,#7072,#389,.T.) ;
#9121=EDGE_CURVE('',#7073,#7072,#390,.T.) ;
#9122=EDGE_CURVE('',#7073,#7074,#4391,.T.) ;
#9123=EDGE_CURVE('',#7075,#7074,#391,.T.) ;
#9124=EDGE_CURVE('',#7075,#7076,#392,.T.) ;
#9125=EDGE_CURVE('',#7076,#7077,#4392,.T.) ;
#9126=EDGE_CURVE('',#7077,#7078,#393,.T.) ;
#9127=EDGE_CURVE('',#7079,#7078,#394,.T.) ;
#9128=EDGE_CURVE('',#7079,#7080,#4393,.T.) ;
#9129=EDGE_CURVE('',#7081,#7080,#395,.T.) ;
#9130=EDGE_CURVE('',#7081,#7082,#396,.T.) ;
#9131=EDGE_CURVE('',#7082,#7083,#4394,.T.) ;
#9132=EDGE_CURVE('',#7083,#7084,#397,.T.) ;
#9133=EDGE_CURVE('',#7085,#7084,#398,.T.) ;
#9134=EDGE_CURVE('',#7085,#7086,#4395,.T.) ;
#9135=EDGE_CURVE('',#7087,#7086,#399,.T.) ;
#9136=EDGE_CURVE('',#7087,#7088,#400,.T.) ;
#9137=EDGE_CURVE('',#7088,#7089,#4396,.T.) ;
#9138=EDGE_CURVE('',#7089,#7090,#401,.T.) ;
#9139=EDGE_CURVE('',#7091,#7090,#402,.T.) ;
#9140=EDGE_CURVE('',#7091,#7092,#4397,.T.) ;
#9141=EDGE_CURVE('',#7093,#7092,#403,.T.) ;
#9142=EDGE_CURVE('',#7093,#7094,#404,.T.) ;
#9143=EDGE_CURVE('',#7094,#7095,#4398,.T.) ;
#9144=EDGE_CURVE('',#7095,#7096,#405,.T.) ;
#9145=EDGE_CURVE('',#7097,#7096,#406,.T.) ;
#9146=EDGE_CURVE('',#7097,#7098,#4399,.T.) ;
#9147=EDGE_CURVE('',#7099,#7098,#407,.T.) ;
#9148=EDGE_CURVE('',#7099,#7100,#408,.T.) ;
#9149=EDGE_CURVE('',#7100,#7101,#4400,.T.) ;
#9150=EDGE_CURVE('',#7101,#7102,#409,.T.) ;
#9151=EDGE_CURVE('',#7103,#7102,#410,.T.) ;
#9152=EDGE_CURVE('',#7103,#7104,#4401,.T.) ;
#9153=EDGE_CURVE('',#7105,#7104,#411,.T.) ;
#9154=EDGE_CURVE('',#7105,#7106,#412,.T.) ;
#9155=EDGE_CURVE('',#7106,#7107,#4402,.T.) ;
#9156=EDGE_CURVE('',#7107,#7108,#413,.T.) ;
#9157=EDGE_CURVE('',#7109,#7108,#414,.T.) ;
#9158=EDGE_CURVE('',#7109,#7110,#4403,.T.) ;
#9159=EDGE_CURVE('',#7111,#7110,#415,.T.) ;
#9160=EDGE_CURVE('',#7111,#7112,#416,.T.) ;
#9161=EDGE_CURVE('',#7112,#7113,#4404,.T.) ;
#9162=EDGE_CURVE('',#7113,#7114,#417,.T.) ;
#9163=EDGE_CURVE('',#7115,#7114,#418,.T.) ;
#9164=EDGE_CURVE('',#7115,#7116,#4405,.T.) ;
#9165=EDGE_CURVE('',#7117,#7116,#419,.T.) ;
#9166=EDGE_CURVE('',#7117,#7118,#420,.T.) ;
#9167=EDGE_CURVE('',#7118,#7119,#4406,.T.) ;
#9168=EDGE_CURVE('',#7119,#7120,#421,.T.) ;
#9169=EDGE_CURVE('',#7121,#7120,#422,.T.) ;
#9170=EDGE_CURVE('',#7121,#7122,#4407,.T.) ;
#9171=EDGE_CURVE('',#7123,#7122,#423,.T.) ;
#9172=EDGE_CURVE('',#7123,#7124,#424,.T.) ;
#9173=EDGE_CURVE('',#7124,#7125,#4408,.T.) ;
#9174=EDGE_CURVE('',#7125,#7126,#425,.T.) ;
#9175=EDGE_CURVE('',#7127,#7126,#426,.T.) ;
#9176=EDGE_CURVE('',#7127,#7128,#4409,.T.) ;
#9177=EDGE_CURVE('',#7129,#7128,#427,.T.) ;
#9178=EDGE_CURVE('',#7129,#7130,#428,.T.) ;
#9179=EDGE_CURVE('',#7130,#7131,#4410,.T.) ;
#9180=EDGE_CURVE('',#7131,#7132,#429,.T.) ;
#9181=EDGE_CURVE('',#7133,#7132,#430,.T.) ;
#9182=EDGE_CURVE('',#7133,#7134,#4411,.T.) ;
#9183=EDGE_CURVE('',#7135,#7134,#431,.T.) ;
#9184=EDGE_CURVE('',#7135,#7136,#432,.T.) ;
#9185=EDGE_CURVE('',#7136,#7137,#4412,.T.) ;
#9186=EDGE_CURVE('',#7137,#7138,#433,.T.) ;
#9187=EDGE_CURVE('',#7139,#7138,#434,.T.) ;
#9188=EDGE_CURVE('',#7139,#7140,#4413,.T.) ;
#9189=EDGE_CURVE('',#7141,#7140,#435,.T.) ;
#9190=EDGE_CURVE('',#7141,#7142,#436,.T.) ;
#9191=EDGE_CURVE('',#7142,#7143,#4414,.T.) ;
#9192=EDGE_CURVE('',#7143,#7144,#437,.T.) ;
#9193=EDGE_CURVE('',#7145,#7144,#438,.T.) ;
#9194=EDGE_CURVE('',#7145,#7146,#4415,.T.) ;
#9195=EDGE_CURVE('',#7147,#7146,#439,.T.) ;
#9196=EDGE_CURVE('',#7147,#7148,#440,.T.) ;
#9197=EDGE_CURVE('',#7148,#7149,#4416,.T.) ;
#9198=EDGE_CURVE('',#7149,#7150,#441,.T.) ;
#9199=EDGE_CURVE('',#7151,#7150,#442,.T.) ;
#9200=EDGE_CURVE('',#7151,#7152,#4417,.T.) ;
#9201=EDGE_CURVE('',#7153,#7152,#443,.T.) ;
#9202=EDGE_CURVE('',#7153,#7154,#444,.T.) ;
#9203=EDGE_CURVE('',#7154,#7155,#4418,.T.) ;
#9204=EDGE_CURVE('',#7155,#7156,#445,.T.) ;
#9205=EDGE_CURVE('',#7157,#7156,#446,.T.) ;
#9206=EDGE_CURVE('',#7157,#7158,#4419,.T.) ;
#9207=EDGE_CURVE('',#7159,#7158,#447,.T.) ;
#9208=EDGE_CURVE('',#7159,#7160,#448,.T.) ;
#9209=EDGE_CURVE('',#7160,#6986,#4420,.T.) ;
#9210=EDGE_CURVE('',#6985,#7161,#5255,.T.) ;
#9211=EDGE_CURVE('',#7162,#7161,#4421,.T.) ;
#9212=EDGE_CURVE('',#7163,#7162,#449,.T.) ;
#9213=EDGE_CURVE('',#7164,#7163,#99,.T.) ;
#9214=EDGE_CURVE('',#7162,#7164,#450,.T.) ;
#9215=EDGE_CURVE('',#7165,#7162,#4422,.T.) ;
#9216=EDGE_CURVE('',#7166,#7165,#451,.T.) ;
#9217=EDGE_CURVE('',#7167,#7166,#100,.T.) ;
#9218=EDGE_CURVE('',#7165,#7167,#452,.T.) ;
#9219=EDGE_CURVE('',#7168,#7165,#4423,.T.) ;
#9220=EDGE_CURVE('',#7169,#7168,#453,.T.) ;
#9221=EDGE_CURVE('',#7170,#7169,#101,.T.) ;
#9222=EDGE_CURVE('',#7168,#7170,#454,.T.) ;
#9223=EDGE_CURVE('',#7171,#7168,#4424,.T.) ;
#9224=EDGE_CURVE('',#7172,#7171,#455,.T.) ;
#9225=EDGE_CURVE('',#7173,#7172,#102,.T.) ;
#9226=EDGE_CURVE('',#7171,#7173,#456,.T.) ;
#9227=EDGE_CURVE('',#7174,#7171,#4425,.T.) ;
#9228=EDGE_CURVE('',#7175,#7174,#457,.T.) ;
#9229=EDGE_CURVE('',#7176,#7175,#103,.T.) ;
#9230=EDGE_CURVE('',#7174,#7176,#458,.T.) ;
#9231=EDGE_CURVE('',#7177,#7174,#4426,.T.) ;
#9232=EDGE_CURVE('',#7178,#7177,#459,.T.) ;
#9233=EDGE_CURVE('',#7179,#7178,#104,.T.) ;
#9234=EDGE_CURVE('',#7177,#7179,#460,.T.) ;
#9235=EDGE_CURVE('',#7180,#7177,#4427,.T.) ;
#9236=EDGE_CURVE('',#7181,#7180,#461,.T.) ;
#9237=EDGE_CURVE('',#7182,#7181,#105,.T.) ;
#9238=EDGE_CURVE('',#7180,#7182,#462,.T.) ;
#9239=EDGE_CURVE('',#7183,#7180,#4428,.T.) ;
#9240=EDGE_CURVE('',#7184,#7183,#463,.T.) ;
#9241=EDGE_CURVE('',#7185,#7184,#106,.T.) ;
#9242=EDGE_CURVE('',#7183,#7185,#464,.T.) ;
#9243=EDGE_CURVE('',#7186,#7183,#4429,.T.) ;
#9244=EDGE_CURVE('',#7187,#7186,#4430,.T.) ;
#9245=EDGE_CURVE('',#7188,#7187,#465,.T.) ;
#9246=EDGE_CURVE('',#7189,#7188,#107,.T.) ;
#9247=EDGE_CURVE('',#7187,#7189,#466,.T.) ;
#9248=EDGE_CURVE('',#7190,#7187,#4431,.T.) ;
#9249=EDGE_CURVE('',#7191,#7190,#467,.T.) ;
#9250=EDGE_CURVE('',#7192,#7191,#108,.T.) ;
#9251=EDGE_CURVE('',#7190,#7192,#468,.T.) ;
#9252=EDGE_CURVE('',#7193,#7190,#4432,.T.) ;
#9253=EDGE_CURVE('',#7194,#7193,#469,.T.) ;
#9254=EDGE_CURVE('',#7195,#7194,#109,.T.) ;
#9255=EDGE_CURVE('',#7193,#7195,#470,.T.) ;
#9256=EDGE_CURVE('',#7196,#7193,#4433,.T.) ;
#9257=EDGE_CURVE('',#7197,#7196,#471,.T.) ;
#9258=EDGE_CURVE('',#7198,#7197,#110,.T.) ;
#9259=EDGE_CURVE('',#7196,#7198,#472,.T.) ;
#9260=EDGE_CURVE('',#7199,#7196,#4434,.T.) ;
#9261=EDGE_CURVE('',#7200,#7199,#4435,.T.) ;
#9262=EDGE_CURVE('',#7201,#7200,#473,.T.) ;
#9263=EDGE_CURVE('',#7202,#7201,#111,.T.) ;
#9264=EDGE_CURVE('',#7200,#7202,#474,.T.) ;
#9265=EDGE_CURVE('',#7203,#7200,#4436,.T.) ;
#9266=EDGE_CURVE('',#7204,#7203,#475,.T.) ;
#9267=EDGE_CURVE('',#7205,#7204,#112,.T.) ;
#9268=EDGE_CURVE('',#7203,#7205,#476,.T.) ;
#9269=EDGE_CURVE('',#7206,#7203,#4437,.T.) ;
#9270=EDGE_CURVE('',#7207,#7206,#477,.T.) ;
#9271=EDGE_CURVE('',#7208,#7207,#113,.T.) ;
#9272=EDGE_CURVE('',#7206,#7208,#478,.T.) ;
#9273=EDGE_CURVE('',#7209,#7206,#4438,.T.) ;
#9274=EDGE_CURVE('',#7210,#7209,#479,.T.) ;
#9275=EDGE_CURVE('',#7211,#7210,#114,.T.) ;
#9276=EDGE_CURVE('',#7209,#7211,#480,.T.) ;
#9277=EDGE_CURVE('',#7212,#7209,#4439,.T.) ;
#9278=EDGE_CURVE('',#7213,#7212,#481,.T.) ;
#9279=EDGE_CURVE('',#7214,#7213,#115,.T.) ;
#9280=EDGE_CURVE('',#7212,#7214,#482,.T.) ;
#9281=EDGE_CURVE('',#7215,#7212,#4440,.T.) ;
#9282=EDGE_CURVE('',#7216,#7215,#483,.T.) ;
#9283=EDGE_CURVE('',#7217,#7216,#116,.T.) ;
#9284=EDGE_CURVE('',#7215,#7217,#484,.T.) ;
#9285=EDGE_CURVE('',#7218,#7215,#4441,.T.) ;
#9286=EDGE_CURVE('',#7219,#7218,#485,.T.) ;
#9287=EDGE_CURVE('',#7220,#7219,#117,.T.) ;
#9288=EDGE_CURVE('',#7218,#7220,#486,.T.) ;
#9289=EDGE_CURVE('',#7221,#7218,#4442,.T.) ;
#9290=EDGE_CURVE('',#7222,#7221,#487,.T.) ;
#9291=EDGE_CURVE('',#7223,#7222,#118,.T.) ;
#9292=EDGE_CURVE('',#7221,#7223,#488,.T.) ;
#9293=EDGE_CURVE('',#7224,#7221,#4443,.T.) ;
#9294=EDGE_CURVE('',#7225,#7224,#489,.T.) ;
#9295=EDGE_CURVE('',#7226,#7225,#119,.T.) ;
#9296=EDGE_CURVE('',#7224,#7226,#490,.T.) ;
#9297=EDGE_CURVE('',#7227,#7224,#4444,.T.) ;
#9298=EDGE_CURVE('',#7228,#7227,#491,.T.) ;
#9299=EDGE_CURVE('',#7229,#7228,#120,.T.) ;
#9300=EDGE_CURVE('',#7227,#7229,#492,.T.) ;
#9301=EDGE_CURVE('',#7230,#7227,#4445,.T.) ;
#9302=EDGE_CURVE('',#7231,#7230,#493,.T.) ;
#9303=EDGE_CURVE('',#7232,#7231,#121,.T.) ;
#9304=EDGE_CURVE('',#7230,#7232,#494,.T.) ;
#9305=EDGE_CURVE('',#7233,#7230,#4446,.T.) ;
#9306=EDGE_CURVE('',#7234,#7233,#495,.T.) ;
#9307=EDGE_CURVE('',#7235,#7234,#122,.T.) ;
#9308=EDGE_CURVE('',#7233,#7235,#496,.T.) ;
#9309=EDGE_CURVE('',#7236,#7233,#4447,.T.) ;
#9310=EDGE_CURVE('',#7237,#7236,#497,.T.) ;
#9311=EDGE_CURVE('',#7238,#7237,#123,.T.) ;
#9312=EDGE_CURVE('',#7236,#7238,#498,.T.) ;
#9313=EDGE_CURVE('',#7239,#7236,#4448,.T.) ;
#9314=EDGE_CURVE('',#7240,#7239,#499,.T.) ;
#9315=EDGE_CURVE('',#7241,#7240,#124,.T.) ;
#9316=EDGE_CURVE('',#7239,#7241,#500,.T.) ;
#9317=EDGE_CURVE('',#7242,#7239,#4449,.T.) ;
#9318=EDGE_CURVE('',#7243,#7242,#501,.T.) ;
#9319=EDGE_CURVE('',#7244,#7243,#125,.T.) ;
#9320=EDGE_CURVE('',#7242,#7244,#502,.T.) ;
#9321=EDGE_CURVE('',#7161,#7242,#4450,.T.) ;
#9322=EDGE_CURVE('',#7245,#7186,#503,.T.) ;
#9323=EDGE_CURVE('',#7246,#7245,#126,.T.) ;
#9324=EDGE_CURVE('',#7186,#7246,#504,.T.) ;
#9325=EDGE_CURVE('',#7247,#7199,#505,.T.) ;
#9326=EDGE_CURVE('',#7248,#7247,#127,.T.) ;
#9327=EDGE_CURVE('',#7199,#7248,#506,.T.) ;
#9328=EDGE_CURVE('',#7160,#7249,#5256,.T.) ;
#9329=EDGE_CURVE('',#7158,#7249,#128,.T.) ;
#9330=EDGE_CURVE('',#7250,#7157,#129,.T.) ;
#9331=EDGE_CURVE('',#7250,#7155,#5257,.T.) ;
#9332=EDGE_CURVE('',#7154,#7251,#5258,.T.) ;
#9333=EDGE_CURVE('',#7152,#7251,#130,.T.) ;
#9334=EDGE_CURVE('',#7252,#7151,#131,.T.) ;
#9335=EDGE_CURVE('',#7252,#7149,#5259,.T.) ;
#9336=EDGE_CURVE('',#7148,#7253,#5260,.T.) ;
#9337=EDGE_CURVE('',#7146,#7253,#132,.T.) ;
#9338=EDGE_CURVE('',#7254,#7145,#133,.T.) ;
#9339=EDGE_CURVE('',#7254,#7143,#5261,.T.) ;
#9340=EDGE_CURVE('',#7142,#7255,#5262,.T.) ;
#9341=EDGE_CURVE('',#7140,#7255,#134,.T.) ;
#9342=EDGE_CURVE('',#7256,#7139,#135,.T.) ;
#9343=EDGE_CURVE('',#7256,#7137,#5263,.T.) ;
#9344=EDGE_CURVE('',#7136,#7257,#5264,.T.) ;
#9345=EDGE_CURVE('',#7134,#7257,#136,.T.) ;
#9346=EDGE_CURVE('',#7258,#7133,#137,.T.) ;
#9347=EDGE_CURVE('',#7258,#7131,#5265,.T.) ;
#9348=EDGE_CURVE('',#7130,#7259,#5266,.T.) ;
#9349=EDGE_CURVE('',#7128,#7259,#138,.T.) ;
#9350=EDGE_CURVE('',#7260,#7127,#139,.T.) ;
#9351=EDGE_CURVE('',#7260,#7125,#5267,.T.) ;
#9352=EDGE_CURVE('',#7124,#7261,#5268,.T.) ;
#9353=EDGE_CURVE('',#7122,#7261,#140,.T.) ;
#9354=EDGE_CURVE('',#7262,#7121,#141,.T.) ;
#9355=EDGE_CURVE('',#7262,#7119,#5269,.T.) ;
#9356=EDGE_CURVE('',#7118,#7263,#5270,.T.) ;
#9357=EDGE_CURVE('',#7116,#7263,#142,.T.) ;
#9358=EDGE_CURVE('',#7264,#7115,#143,.T.) ;
#9359=EDGE_CURVE('',#7264,#7113,#5271,.T.) ;
#9360=EDGE_CURVE('',#7112,#7265,#5272,.T.) ;
#9361=EDGE_CURVE('',#7110,#7265,#144,.T.) ;
#9362=EDGE_CURVE('',#7266,#7109,#145,.T.) ;
#9363=EDGE_CURVE('',#7266,#7107,#5273,.T.) ;
#9364=EDGE_CURVE('',#7106,#7267,#5274,.T.) ;
#9365=EDGE_CURVE('',#7104,#7267,#146,.T.) ;
#9366=EDGE_CURVE('',#7268,#7103,#147,.T.) ;
#9367=EDGE_CURVE('',#7268,#7101,#5275,.T.) ;
#9368=EDGE_CURVE('',#7100,#7269,#5276,.T.) ;
#9369=EDGE_CURVE('',#7098,#7269,#148,.T.) ;
#9370=EDGE_CURVE('',#7270,#7097,#149,.T.) ;
#9371=EDGE_CURVE('',#7270,#7095,#5277,.T.) ;
#9372=EDGE_CURVE('',#7094,#7271,#5278,.T.) ;
#9373=EDGE_CURVE('',#7092,#7271,#150,.T.) ;
#9374=EDGE_CURVE('',#7272,#7091,#151,.T.) ;
#9375=EDGE_CURVE('',#7272,#7089,#5279,.T.) ;
#9376=EDGE_CURVE('',#7088,#7273,#5280,.T.) ;
#9377=EDGE_CURVE('',#7086,#7273,#152,.T.) ;
#9378=EDGE_CURVE('',#7274,#7085,#153,.T.) ;
#9379=EDGE_CURVE('',#7274,#7083,#5281,.T.) ;
#9380=EDGE_CURVE('',#7082,#7275,#5282,.T.) ;
#9381=EDGE_CURVE('',#7080,#7275,#154,.T.) ;
#9382=EDGE_CURVE('',#7276,#7079,#155,.T.) ;
#9383=EDGE_CURVE('',#7276,#7077,#5283,.T.) ;
#9384=EDGE_CURVE('',#7076,#7277,#5284,.T.) ;
#9385=EDGE_CURVE('',#7074,#7277,#156,.T.) ;
#9386=EDGE_CURVE('',#7278,#7073,#157,.T.) ;
#9387=EDGE_CURVE('',#7278,#7071,#5285,.T.) ;
#9388=EDGE_CURVE('',#7070,#7279,#5286,.T.) ;
#9389=EDGE_CURVE('',#7068,#7279,#158,.T.) ;
#9390=EDGE_CURVE('',#7280,#7067,#159,.T.) ;
#9391=EDGE_CURVE('',#7280,#7065,#5287,.T.) ;
#9392=EDGE_CURVE('',#7064,#7281,#5288,.T.) ;
#9393=EDGE_CURVE('',#7062,#7281,#160,.T.) ;
#9394=EDGE_CURVE('',#7282,#7061,#161,.T.) ;
#9395=EDGE_CURVE('',#7282,#7059,#5289,.T.) ;
#9396=EDGE_CURVE('',#7058,#7283,#5290,.T.) ;
#9397=EDGE_CURVE('',#7056,#7283,#162,.T.) ;
#9398=EDGE_CURVE('',#7284,#7055,#163,.T.) ;
#9399=EDGE_CURVE('',#7284,#7053,#5291,.T.) ;
#9400=EDGE_CURVE('',#7052,#7285,#5292,.T.) ;
#9401=EDGE_CURVE('',#7050,#7285,#164,.T.) ;
#9402=EDGE_CURVE('',#7286,#7049,#165,.T.) ;
#9403=EDGE_CURVE('',#7286,#7047,#5293,.T.) ;
#9404=EDGE_CURVE('',#7046,#7287,#5294,.T.) ;
#9405=EDGE_CURVE('',#7044,#7287,#166,.T.) ;
#9406=EDGE_CURVE('',#7288,#7043,#167,.T.) ;
#9407=EDGE_CURVE('',#7288,#7041,#5295,.T.) ;
#9408=EDGE_CURVE('',#7040,#7289,#5296,.T.) ;
#9409=EDGE_CURVE('',#7038,#7289,#168,.T.) ;
#9410=EDGE_CURVE('',#7290,#7037,#169,.T.) ;
#9411=EDGE_CURVE('',#7290,#7035,#5297,.T.) ;
#9412=EDGE_CURVE('',#7034,#7291,#5298,.T.) ;
#9413=EDGE_CURVE('',#7032,#7291,#170,.T.) ;
#9414=EDGE_CURVE('',#7292,#7031,#171,.T.) ;
#9415=EDGE_CURVE('',#7292,#7029,#5299,.T.) ;
#9416=EDGE_CURVE('',#7028,#7293,#5300,.T.) ;
#9417=EDGE_CURVE('',#7026,#7293,#172,.T.) ;
#9418=EDGE_CURVE('',#7294,#7025,#173,.T.) ;
#9419=EDGE_CURVE('',#7294,#7023,#5301,.T.) ;
#9420=EDGE_CURVE('',#7022,#7295,#5302,.T.) ;
#9421=EDGE_CURVE('',#7020,#7295,#174,.T.) ;
#9422=EDGE_CURVE('',#7296,#7019,#175,.T.) ;
#9423=EDGE_CURVE('',#7296,#7017,#5303,.T.) ;
#9424=EDGE_CURVE('',#7016,#7297,#5304,.T.) ;
#9425=EDGE_CURVE('',#7014,#7297,#176,.T.) ;
#9426=EDGE_CURVE('',#7298,#7013,#177,.T.) ;
#9427=EDGE_CURVE('',#7298,#7011,#5305,.T.) ;
#9428=EDGE_CURVE('',#7010,#7299,#5306,.T.) ;
#9429=EDGE_CURVE('',#7008,#7299,#178,.T.) ;
#9430=EDGE_CURVE('',#7300,#7007,#179,.T.) ;
#9431=EDGE_CURVE('',#7300,#7005,#5307,.T.) ;
#9432=EDGE_CURVE('',#7004,#7301,#5308,.T.) ;
#9433=EDGE_CURVE('',#7002,#7301,#180,.T.) ;
#9434=EDGE_CURVE('',#7302,#7001,#181,.T.) ;
#9435=EDGE_CURVE('',#7302,#6999,#5309,.T.) ;
#9436=EDGE_CURVE('',#6998,#7303,#5310,.T.) ;
#9437=EDGE_CURVE('',#6996,#7303,#182,.T.) ;
#9438=EDGE_CURVE('',#7304,#6995,#183,.T.) ;
#9439=EDGE_CURVE('',#7304,#6993,#5311,.T.) ;
#9440=EDGE_CURVE('',#6992,#7305,#5312,.T.) ;
#9441=EDGE_CURVE('',#6990,#7305,#184,.T.) ;
#9442=EDGE_CURVE('',#7306,#6989,#185,.T.) ;
#9443=EDGE_CURVE('',#7306,#6987,#5313,.T.) ;
#9444=EDGE_CURVE('',#6986,#7307,#5314,.T.) ;
#9445=EDGE_CURVE('',#7307,#7307,#4451,.T.) ;
#9446=EDGE_CURVE('',#7308,#7308,#4452,.T.) ;
#9447=EDGE_CURVE('',#7308,#7309,#5315,.T.) ;
#9448=EDGE_CURVE('',#7309,#7309,#4453,.T.) ;
#9449=EDGE_CURVE('',#7310,#7311,#507,.T.) ;
#9450=EDGE_CURVE('',#7312,#7310,#186,.T.) ;
#9451=EDGE_CURVE('',#7311,#7312,#508,.T.) ;
#9452=EDGE_CURVE('',#7313,#7314,#187,.T.) ;
#9453=EDGE_CURVE('',#7315,#7313,#509,.T.) ;
#9454=EDGE_CURVE('',#7314,#7315,#510,.T.) ;
#9455=EDGE_CURVE('',#7316,#7317,#188,.T.) ;
#9456=EDGE_CURVE('',#7318,#7316,#511,.T.) ;
#9457=EDGE_CURVE('',#7317,#7318,#512,.T.) ;
#9458=EDGE_CURVE('',#7319,#7320,#189,.T.) ;
#9459=EDGE_CURVE('',#7321,#7319,#513,.T.) ;
#9460=EDGE_CURVE('',#7320,#7321,#514,.T.) ;
#9461=EDGE_CURVE('',#7322,#7323,#190,.T.) ;
#9462=EDGE_CURVE('',#7324,#7322,#515,.T.) ;
#9463=EDGE_CURVE('',#7323,#7324,#516,.T.) ;
#9464=EDGE_CURVE('',#7325,#7326,#191,.T.) ;
#9465=EDGE_CURVE('',#7327,#7325,#517,.T.) ;
#9466=EDGE_CURVE('',#7326,#7327,#518,.T.) ;
#9467=EDGE_CURVE('',#7328,#7329,#192,.T.) ;
#9468=EDGE_CURVE('',#7330,#7328,#519,.T.) ;
#9469=EDGE_CURVE('',#7329,#7330,#520,.T.) ;
#9470=EDGE_CURVE('',#7331,#7332,#193,.T.) ;
#9471=EDGE_CURVE('',#7333,#7331,#521,.T.) ;
#9472=EDGE_CURVE('',#7332,#7333,#522,.T.) ;
#9473=EDGE_CURVE('',#7334,#7335,#194,.T.) ;
#9474=EDGE_CURVE('',#7336,#7334,#523,.T.) ;
#9475=EDGE_CURVE('',#7335,#7336,#524,.T.) ;
#9476=EDGE_CURVE('',#7337,#7338,#195,.T.) ;
#9477=EDGE_CURVE('',#7339,#7337,#525,.T.) ;
#9478=EDGE_CURVE('',#7338,#7339,#526,.T.) ;
#9479=EDGE_CURVE('',#7340,#7341,#196,.T.) ;
#9480=EDGE_CURVE('',#7342,#7340,#527,.T.) ;
#9481=EDGE_CURVE('',#7341,#7342,#528,.T.) ;
#9482=EDGE_CURVE('',#7343,#7344,#197,.T.) ;
#9483=EDGE_CURVE('',#7345,#7343,#529,.T.) ;
#9484=EDGE_CURVE('',#7344,#7345,#530,.T.) ;
#9485=EDGE_CURVE('',#7346,#7347,#198,.T.) ;
#9486=EDGE_CURVE('',#7348,#7346,#531,.T.) ;
#9487=EDGE_CURVE('',#7347,#7348,#532,.T.) ;
#9488=EDGE_CURVE('',#7349,#7350,#199,.T.) ;
#9489=EDGE_CURVE('',#7351,#7349,#533,.T.) ;
#9490=EDGE_CURVE('',#7350,#7351,#534,.T.) ;
#9491=EDGE_CURVE('',#7352,#7353,#200,.T.) ;
#9492=EDGE_CURVE('',#7354,#7352,#535,.T.) ;
#9493=EDGE_CURVE('',#7353,#7354,#536,.T.) ;
#9494=EDGE_CURVE('',#7355,#7356,#201,.T.) ;
#9495=EDGE_CURVE('',#7357,#7355,#537,.T.) ;
#9496=EDGE_CURVE('',#7356,#7357,#538,.T.) ;
#9497=EDGE_CURVE('',#7358,#7359,#202,.T.) ;
#9498=EDGE_CURVE('',#7360,#7358,#539,.T.) ;
#9499=EDGE_CURVE('',#7359,#7360,#540,.T.) ;
#9500=EDGE_CURVE('',#7361,#7362,#203,.T.) ;
#9501=EDGE_CURVE('',#7363,#7361,#541,.T.) ;
#9502=EDGE_CURVE('',#7362,#7363,#542,.T.) ;
#9503=EDGE_CURVE('',#7364,#7365,#204,.T.) ;
#9504=EDGE_CURVE('',#7366,#7364,#543,.T.) ;
#9505=EDGE_CURVE('',#7365,#7366,#544,.T.) ;
#9506=EDGE_CURVE('',#7367,#7368,#205,.T.) ;
#9507=EDGE_CURVE('',#7369,#7367,#545,.T.) ;
#9508=EDGE_CURVE('',#7368,#7369,#546,.T.) ;
#9509=EDGE_CURVE('',#7370,#7371,#206,.T.) ;
#9510=EDGE_CURVE('',#7372,#7370,#547,.T.) ;
#9511=EDGE_CURVE('',#7371,#7372,#548,.T.) ;
#9512=EDGE_CURVE('',#7373,#7374,#207,.T.) ;
#9513=EDGE_CURVE('',#7375,#7373,#549,.T.) ;
#9514=EDGE_CURVE('',#7374,#7375,#550,.T.) ;
#9515=EDGE_CURVE('',#7376,#7377,#208,.T.) ;
#9516=EDGE_CURVE('',#7378,#7376,#551,.T.) ;
#9517=EDGE_CURVE('',#7377,#7378,#552,.T.) ;
#9518=EDGE_CURVE('',#7379,#7380,#209,.T.) ;
#9519=EDGE_CURVE('',#7381,#7379,#553,.T.) ;
#9520=EDGE_CURVE('',#7380,#7381,#554,.T.) ;
#9521=EDGE_CURVE('',#7382,#7383,#210,.T.) ;
#9522=EDGE_CURVE('',#7384,#7382,#555,.T.) ;
#9523=EDGE_CURVE('',#7383,#7384,#556,.T.) ;
#9524=EDGE_CURVE('',#7385,#7386,#211,.T.) ;
#9525=EDGE_CURVE('',#7387,#7385,#557,.T.) ;
#9526=EDGE_CURVE('',#7386,#7387,#558,.T.) ;
#9527=EDGE_CURVE('',#7388,#7389,#212,.T.) ;
#9528=EDGE_CURVE('',#7390,#7388,#559,.T.) ;
#9529=EDGE_CURVE('',#7389,#7390,#560,.T.) ;
#9530=EDGE_CURVE('',#7391,#7392,#213,.T.) ;
#9531=EDGE_CURVE('',#7393,#7391,#561,.T.) ;
#9532=EDGE_CURVE('',#7392,#7393,#562,.T.) ;
#9533=EDGE_CURVE('',#7394,#7395,#214,.T.) ;
#9534=EDGE_CURVE('',#7396,#7394,#563,.T.) ;
#9535=EDGE_CURVE('',#7395,#7396,#564,.T.) ;
#9536=EDGE_CURVE('',#7397,#7397,#4454,.T.) ;
#9537=EDGE_CURVE('',#7397,#7398,#5316,.T.) ;
#9538=EDGE_CURVE('',#7398,#7398,#4455,.T.) ;
#9539=EDGE_CURVE('',#7399,#7399,#4456,.T.) ;
#9540=EDGE_CURVE('',#7399,#7400,#4457,.T.) ;
#9541=EDGE_CURVE('',#7400,#7400,#4458,.T.) ;
#9542=EDGE_CURVE('',#7401,#7401,#4459,.T.) ;
#9543=EDGE_CURVE('',#7401,#7402,#4460,.T.) ;
#9544=EDGE_CURVE('',#7402,#7402,#4461,.T.) ;
#9545=EDGE_CURVE('',#7403,#7403,#4462,.T.) ;
#9546=EDGE_CURVE('',#7403,#7404,#4463,.T.) ;
#9547=EDGE_CURVE('',#7404,#7404,#4464,.T.) ;
#9548=EDGE_CURVE('',#7400,#7405,#5317,.T.) ;
#9549=EDGE_CURVE('',#7405,#7405,#4465,.T.) ;
#9550=EDGE_CURVE('',#7405,#7406,#4466,.T.) ;
#9551=EDGE_CURVE('',#7406,#7406,#4467,.T.) ;
#9552=EDGE_CURVE('',#7402,#7403,#5318,.T.) ;
#9553=EDGE_CURVE('',#7311,#7200,#4468,.T.) ;
#9554=EDGE_CURVE('',#7200,#7311,#4469,.T.) ;
#9555=EDGE_CURVE('',#7396,#7203,#4470,.T.) ;
#9556=EDGE_CURVE('',#7203,#7396,#4471,.T.) ;
#9557=EDGE_CURVE('',#7357,#7206,#4472,.T.) ;
#9558=EDGE_CURVE('',#7206,#7357,#4473,.T.) ;
#9559=EDGE_CURVE('',#7393,#7209,#4474,.T.) ;
#9560=EDGE_CURVE('',#7209,#7393,#4475,.T.) ;
#9561=EDGE_CURVE('',#7360,#7212,#4476,.T.) ;
#9562=EDGE_CURVE('',#7212,#7360,#4477,.T.) ;
#9563=EDGE_CURVE('',#7390,#7215,#4478,.T.) ;
#9564=EDGE_CURVE('',#7215,#7390,#4479,.T.) ;
#9565=EDGE_CURVE('',#7363,#7218,#4480,.T.) ;
#9566=EDGE_CURVE('',#7218,#7363,#4481,.T.) ;
#9567=EDGE_CURVE('',#7387,#7221,#4482,.T.) ;
#9568=EDGE_CURVE('',#7221,#7387,#4483,.T.) ;
#9569=EDGE_CURVE('',#7366,#7224,#4484,.T.) ;
#9570=EDGE_CURVE('',#7224,#7366,#4485,.T.) ;
#9571=EDGE_CURVE('',#7384,#7227,#4486,.T.) ;
#9572=EDGE_CURVE('',#7227,#7384,#4487,.T.) ;
#9573=EDGE_CURVE('',#7369,#7230,#4488,.T.) ;
#9574=EDGE_CURVE('',#7230,#7369,#4489,.T.) ;
#9575=EDGE_CURVE('',#7381,#7233,#4490,.T.) ;
#9576=EDGE_CURVE('',#7233,#7381,#4491,.T.) ;
#9577=EDGE_CURVE('',#7372,#7236,#4492,.T.) ;
#9578=EDGE_CURVE('',#7236,#7372,#4493,.T.) ;
#9579=EDGE_CURVE('',#7378,#7239,#4494,.T.) ;
#9580=EDGE_CURVE('',#7239,#7378,#4495,.T.) ;
#9581=EDGE_CURVE('',#7375,#7242,#4496,.T.) ;
#9582=EDGE_CURVE('',#7242,#7375,#4497,.T.) ;
#9583=EDGE_CURVE('',#7333,#7162,#4498,.T.) ;
#9584=EDGE_CURVE('',#7162,#7333,#4499,.T.) ;
#9585=EDGE_CURVE('',#7336,#7165,#4500,.T.) ;
#9586=EDGE_CURVE('',#7165,#7336,#4501,.T.) ;
#9587=EDGE_CURVE('',#7330,#7168,#4502,.T.) ;
#9588=EDGE_CURVE('',#7168,#7330,#4503,.T.) ;
#9589=EDGE_CURVE('',#7339,#7171,#4504,.T.) ;
#9590=EDGE_CURVE('',#7171,#7339,#4505,.T.) ;
#9591=EDGE_CURVE('',#7327,#7174,#4506,.T.) ;
#9592=EDGE_CURVE('',#7174,#7327,#4507,.T.) ;
#9593=EDGE_CURVE('',#7342,#7177,#4508,.T.) ;
#9594=EDGE_CURVE('',#7177,#7342,#4509,.T.) ;
#9595=EDGE_CURVE('',#7324,#7180,#4510,.T.) ;
#9596=EDGE_CURVE('',#7180,#7324,#4511,.T.) ;
#9597=EDGE_CURVE('',#7345,#7183,#4512,.T.) ;
#9598=EDGE_CURVE('',#7183,#7345,#4513,.T.) ;
#9599=EDGE_CURVE('',#7321,#7186,#4514,.T.) ;
#9600=EDGE_CURVE('',#7186,#7321,#4515,.T.) ;
#9601=EDGE_CURVE('',#7348,#7187,#4516,.T.) ;
#9602=EDGE_CURVE('',#7187,#7348,#4517,.T.) ;
#9603=EDGE_CURVE('',#7318,#7190,#4518,.T.) ;
#9604=EDGE_CURVE('',#7190,#7318,#4519,.T.) ;
#9605=EDGE_CURVE('',#7351,#7193,#4520,.T.) ;
#9606=EDGE_CURVE('',#7193,#7351,#4521,.T.) ;
#9607=EDGE_CURVE('',#7315,#7196,#4522,.T.) ;
#9608=EDGE_CURVE('',#7196,#7315,#4523,.T.) ;
#9609=EDGE_CURVE('',#7354,#7199,#4524,.T.) ;
#9610=EDGE_CURVE('',#7199,#7354,#4525,.T.) ;
#9611=EDGE_CURVE('',#7398,#7161,#5319,.T.) ;
#9612=EDGE_CURVE('',#7075,#7201,#4526,.T.) ;
#9613=EDGE_CURVE('',#7312,#7277,#4527,.T.) ;
#9614=EDGE_CURVE('',#7202,#7072,#4528,.T.) ;
#9615=EDGE_CURVE('',#7278,#7310,#4529,.T.) ;
#9616=EDGE_CURVE('',#7069,#7204,#4530,.T.) ;
#9617=EDGE_CURVE('',#7394,#7279,#4531,.T.) ;
#9618=EDGE_CURVE('',#7205,#7066,#4532,.T.) ;
#9619=EDGE_CURVE('',#7280,#7395,#4533,.T.) ;
#9620=EDGE_CURVE('',#7063,#7207,#4534,.T.) ;
#9621=EDGE_CURVE('',#7355,#7281,#4535,.T.) ;
#9622=EDGE_CURVE('',#7208,#7060,#4536,.T.) ;
#9623=EDGE_CURVE('',#7282,#7356,#4537,.T.) ;
#9624=EDGE_CURVE('',#7057,#7210,#4538,.T.) ;
#9625=EDGE_CURVE('',#7391,#7283,#4539,.T.) ;
#9626=EDGE_CURVE('',#7211,#7054,#4540,.T.) ;
#9627=EDGE_CURVE('',#7284,#7392,#4541,.T.) ;
#9628=EDGE_CURVE('',#7051,#7213,#4542,.T.) ;
#9629=EDGE_CURVE('',#7358,#7285,#4543,.T.) ;
#9630=EDGE_CURVE('',#7214,#7048,#4544,.T.) ;
#9631=EDGE_CURVE('',#7286,#7359,#4545,.T.) ;
#9632=EDGE_CURVE('',#7045,#7216,#4546,.T.) ;
#9633=EDGE_CURVE('',#7388,#7287,#4547,.T.) ;
#9634=EDGE_CURVE('',#7217,#7042,#4548,.T.) ;
#9635=EDGE_CURVE('',#7288,#7389,#4549,.T.) ;
#9636=EDGE_CURVE('',#7039,#7219,#4550,.T.) ;
#9637=EDGE_CURVE('',#7361,#7289,#4551,.T.) ;
#9638=EDGE_CURVE('',#7220,#7036,#4552,.T.) ;
#9639=EDGE_CURVE('',#7290,#7362,#4553,.T.) ;
#9640=EDGE_CURVE('',#7033,#7222,#4554,.T.) ;
#9641=EDGE_CURVE('',#7385,#7291,#4555,.T.) ;
#9642=EDGE_CURVE('',#7223,#7030,#4556,.T.) ;
#9643=EDGE_CURVE('',#7292,#7386,#4557,.T.) ;
#9644=EDGE_CURVE('',#7027,#7225,#4558,.T.) ;
#9645=EDGE_CURVE('',#7364,#7293,#4559,.T.) ;
#9646=EDGE_CURVE('',#7294,#7365,#4560,.T.) ;
#9647=EDGE_CURVE('',#7226,#7024,#4561,.T.) ;
#9648=EDGE_CURVE('',#7021,#7228,#4562,.T.) ;
#9649=EDGE_CURVE('',#7382,#7295,#4563,.T.) ;
#9650=EDGE_CURVE('',#7296,#7383,#4564,.T.) ;
#9651=EDGE_CURVE('',#7229,#7018,#4565,.T.) ;
#9652=EDGE_CURVE('',#7015,#7231,#4566,.T.) ;
#9653=EDGE_CURVE('',#7367,#7297,#4567,.T.) ;
#9654=EDGE_CURVE('',#7298,#7368,#4568,.T.) ;
#9655=EDGE_CURVE('',#7232,#7012,#4569,.T.) ;
#9656=EDGE_CURVE('',#7009,#7234,#4570,.T.) ;
#9657=EDGE_CURVE('',#7379,#7299,#4571,.T.) ;
#9658=EDGE_CURVE('',#7300,#7380,#4572,.T.) ;
#9659=EDGE_CURVE('',#7235,#7006,#4573,.T.) ;
#9660=EDGE_CURVE('',#7003,#7237,#4574,.T.) ;
#9661=EDGE_CURVE('',#7370,#7301,#4575,.T.) ;
#9662=EDGE_CURVE('',#7302,#7371,#4576,.T.) ;
#9663=EDGE_CURVE('',#7238,#7000,#4577,.T.) ;
#9664=EDGE_CURVE('',#6997,#7240,#4578,.T.) ;
#9665=EDGE_CURVE('',#7376,#7303,#4579,.T.) ;
#9666=EDGE_CURVE('',#7304,#7377,#4580,.T.) ;
#9667=EDGE_CURVE('',#7241,#6994,#4581,.T.) ;
#9668=EDGE_CURVE('',#6991,#7243,#4582,.T.) ;
#9669=EDGE_CURVE('',#7373,#7305,#4583,.T.) ;
#9670=EDGE_CURVE('',#7306,#7374,#4584,.T.) ;
#9671=EDGE_CURVE('',#7244,#6988,#4585,.T.) ;
#9672=EDGE_CURVE('',#7159,#7163,#4586,.T.) ;
#9673=EDGE_CURVE('',#7331,#7249,#4587,.T.) ;
#9674=EDGE_CURVE('',#7250,#7332,#4588,.T.) ;
#9675=EDGE_CURVE('',#7164,#7156,#4589,.T.) ;
#9676=EDGE_CURVE('',#7153,#7166,#4590,.T.) ;
#9677=EDGE_CURVE('',#7334,#7251,#4591,.T.) ;
#9678=EDGE_CURVE('',#7252,#7335,#4592,.T.) ;
#9679=EDGE_CURVE('',#7167,#7150,#4593,.T.) ;
#9680=EDGE_CURVE('',#7147,#7169,#4594,.T.) ;
#9681=EDGE_CURVE('',#7328,#7253,#4595,.T.) ;
#9682=EDGE_CURVE('',#7254,#7329,#4596,.T.) ;
#9683=EDGE_CURVE('',#7170,#7144,#4597,.T.) ;
#9684=EDGE_CURVE('',#7141,#7172,#4598,.T.) ;
#9685=EDGE_CURVE('',#7337,#7255,#4599,.T.) ;
#9686=EDGE_CURVE('',#7256,#7338,#4600,.T.) ;
#9687=EDGE_CURVE('',#7173,#7138,#4601,.T.) ;
#9688=EDGE_CURVE('',#7135,#7175,#4602,.T.) ;
#9689=EDGE_CURVE('',#7325,#7257,#4603,.T.) ;
#9690=EDGE_CURVE('',#7258,#7326,#4604,.T.) ;
#9691=EDGE_CURVE('',#7176,#7132,#4605,.T.) ;
#9692=EDGE_CURVE('',#7129,#7178,#4606,.T.) ;
#9693=EDGE_CURVE('',#7340,#7259,#4607,.T.) ;
#9694=EDGE_CURVE('',#7260,#7341,#4608,.T.) ;
#9695=EDGE_CURVE('',#7179,#7126,#4609,.T.) ;
#9696=EDGE_CURVE('',#7123,#7181,#4610,.T.) ;
#9697=EDGE_CURVE('',#7322,#7261,#4611,.T.) ;
#9698=EDGE_CURVE('',#7262,#7323,#4612,.T.) ;
#9699=EDGE_CURVE('',#7182,#7120,#4613,.T.) ;
#9700=EDGE_CURVE('',#7117,#7184,#4614,.T.) ;
#9701=EDGE_CURVE('',#7343,#7263,#4615,.T.) ;
#9702=EDGE_CURVE('',#7185,#7114,#4616,.T.) ;
#9703=EDGE_CURVE('',#7264,#7344,#4617,.T.) ;
#9704=EDGE_CURVE('',#7111,#7245,#4618,.T.) ;
#9705=EDGE_CURVE('',#7319,#7265,#4619,.T.) ;
#9706=EDGE_CURVE('',#7246,#7108,#4620,.T.) ;
#9707=EDGE_CURVE('',#7266,#7320,#4621,.T.) ;
#9708=EDGE_CURVE('',#7105,#7188,#4622,.T.) ;
#9709=EDGE_CURVE('',#7346,#7267,#4623,.T.) ;
#9710=EDGE_CURVE('',#7189,#7102,#4624,.T.) ;
#9711=EDGE_CURVE('',#7268,#7347,#4625,.T.) ;
#9712=EDGE_CURVE('',#7099,#7191,#4626,.T.) ;
#9713=EDGE_CURVE('',#7316,#7269,#4627,.T.) ;
#9714=EDGE_CURVE('',#7192,#7096,#4628,.T.) ;
#9715=EDGE_CURVE('',#7270,#7317,#4629,.T.) ;
#9716=EDGE_CURVE('',#7093,#7194,#4630,.T.) ;
#9717=EDGE_CURVE('',#7349,#7271,#4631,.T.) ;
#9718=EDGE_CURVE('',#7195,#7090,#4632,.T.) ;
#9719=EDGE_CURVE('',#7272,#7350,#4633,.T.) ;
#9720=EDGE_CURVE('',#7087,#7197,#4634,.T.) ;
#9721=EDGE_CURVE('',#7313,#7273,#4635,.T.) ;
#9722=EDGE_CURVE('',#7198,#7084,#4636,.T.) ;
#9723=EDGE_CURVE('',#7274,#7314,#4637,.T.) ;
#9724=EDGE_CURVE('',#7081,#7247,#4638,.T.) ;
#9725=EDGE_CURVE('',#7352,#7275,#4639,.T.) ;
#9726=EDGE_CURVE('',#7248,#7078,#4640,.T.) ;
#9727=EDGE_CURVE('',#7276,#7353,#4641,.T.) ;
#12958=ORIENTED_EDGE('',*,*,#9033,.F.) ;
#12959=ORIENTED_EDGE('',*,*,#9034,.T.) ;
#12960=ORIENTED_EDGE('',*,*,#9035,.T.) ;
#12961=ORIENTED_EDGE('',*,*,#9036,.T.) ;
#12962=ORIENTED_EDGE('',*,*,#9037,.F.) ;
#12963=ORIENTED_EDGE('',*,*,#9038,.T.) ;
#12964=ORIENTED_EDGE('',*,*,#9039,.F.) ;
#12965=ORIENTED_EDGE('',*,*,#9040,.T.) ;
#12966=ORIENTED_EDGE('',*,*,#9041,.T.) ;
#12967=ORIENTED_EDGE('',*,*,#9042,.T.) ;
#12968=ORIENTED_EDGE('',*,*,#9043,.F.) ;
#12969=ORIENTED_EDGE('',*,*,#9044,.T.) ;
#12970=ORIENTED_EDGE('',*,*,#9045,.F.) ;
#12971=ORIENTED_EDGE('',*,*,#9046,.T.) ;
#12972=ORIENTED_EDGE('',*,*,#9047,.T.) ;
#12973=ORIENTED_EDGE('',*,*,#9048,.T.) ;
#12974=ORIENTED_EDGE('',*,*,#9049,.F.) ;
#12975=ORIENTED_EDGE('',*,*,#9050,.T.) ;
#12976=ORIENTED_EDGE('',*,*,#9051,.F.) ;
#12977=ORIENTED_EDGE('',*,*,#9052,.T.) ;
#12978=ORIENTED_EDGE('',*,*,#9053,.T.) ;
#12979=ORIENTED_EDGE('',*,*,#9054,.T.) ;
#12980=ORIENTED_EDGE('',*,*,#9055,.F.) ;
#12981=ORIENTED_EDGE('',*,*,#9056,.T.) ;
#12982=ORIENTED_EDGE('',*,*,#9057,.F.) ;
#12983=ORIENTED_EDGE('',*,*,#9058,.T.) ;
#12984=ORIENTED_EDGE('',*,*,#9059,.T.) ;
#12985=ORIENTED_EDGE('',*,*,#9060,.T.) ;
#12986=ORIENTED_EDGE('',*,*,#9061,.F.) ;
#12987=ORIENTED_EDGE('',*,*,#9062,.T.) ;
#12988=ORIENTED_EDGE('',*,*,#9063,.F.) ;
#12989=ORIENTED_EDGE('',*,*,#9064,.T.) ;
#12990=ORIENTED_EDGE('',*,*,#9065,.T.) ;
#12991=ORIENTED_EDGE('',*,*,#9066,.T.) ;
#12992=ORIENTED_EDGE('',*,*,#9067,.F.) ;
#12993=ORIENTED_EDGE('',*,*,#9068,.T.) ;
#12994=ORIENTED_EDGE('',*,*,#9069,.F.) ;
#12995=ORIENTED_EDGE('',*,*,#9070,.T.) ;
#12996=ORIENTED_EDGE('',*,*,#9071,.T.) ;
#12997=ORIENTED_EDGE('',*,*,#9072,.T.) ;
#12998=ORIENTED_EDGE('',*,*,#9073,.F.) ;
#12999=ORIENTED_EDGE('',*,*,#9074,.T.) ;
#13000=ORIENTED_EDGE('',*,*,#9075,.F.) ;
#13001=ORIENTED_EDGE('',*,*,#9076,.T.) ;
#13002=ORIENTED_EDGE('',*,*,#9077,.T.) ;
#13003=ORIENTED_EDGE('',*,*,#9078,.T.) ;
#13004=ORIENTED_EDGE('',*,*,#9079,.F.) ;
#13005=ORIENTED_EDGE('',*,*,#9080,.T.) ;
#13006=ORIENTED_EDGE('',*,*,#9081,.F.) ;
#13007=ORIENTED_EDGE('',*,*,#9082,.T.) ;
#13008=ORIENTED_EDGE('',*,*,#9083,.T.) ;
#13009=ORIENTED_EDGE('',*,*,#9084,.T.) ;
#13010=ORIENTED_EDGE('',*,*,#9085,.F.) ;
#13011=ORIENTED_EDGE('',*,*,#9086,.T.) ;
#13012=ORIENTED_EDGE('',*,*,#9087,.F.) ;
#13013=ORIENTED_EDGE('',*,*,#9088,.T.) ;
#13014=ORIENTED_EDGE('',*,*,#9089,.T.) ;
#13015=ORIENTED_EDGE('',*,*,#9090,.T.) ;
#13016=ORIENTED_EDGE('',*,*,#9091,.F.) ;
#13017=ORIENTED_EDGE('',*,*,#9092,.T.) ;
#13018=ORIENTED_EDGE('',*,*,#9093,.F.) ;
#13019=ORIENTED_EDGE('',*,*,#9094,.T.) ;
#13020=ORIENTED_EDGE('',*,*,#9095,.T.) ;
#13021=ORIENTED_EDGE('',*,*,#9096,.T.) ;
#13022=ORIENTED_EDGE('',*,*,#9097,.F.) ;
#13023=ORIENTED_EDGE('',*,*,#9098,.T.) ;
#13024=ORIENTED_EDGE('',*,*,#9099,.F.) ;
#13025=ORIENTED_EDGE('',*,*,#9100,.T.) ;
#13026=ORIENTED_EDGE('',*,*,#9101,.T.) ;
#13027=ORIENTED_EDGE('',*,*,#9102,.T.) ;
#13028=ORIENTED_EDGE('',*,*,#9103,.F.) ;
#13029=ORIENTED_EDGE('',*,*,#9104,.T.) ;
#13030=ORIENTED_EDGE('',*,*,#9105,.F.) ;
#13031=ORIENTED_EDGE('',*,*,#9106,.T.) ;
#13032=ORIENTED_EDGE('',*,*,#9107,.T.) ;
#13033=ORIENTED_EDGE('',*,*,#9108,.T.) ;
#13034=ORIENTED_EDGE('',*,*,#9109,.F.) ;
#13035=ORIENTED_EDGE('',*,*,#9110,.T.) ;
#13036=ORIENTED_EDGE('',*,*,#9111,.F.) ;
#13037=ORIENTED_EDGE('',*,*,#9112,.T.) ;
#13038=ORIENTED_EDGE('',*,*,#9113,.T.) ;
#13039=ORIENTED_EDGE('',*,*,#9114,.T.) ;
#13040=ORIENTED_EDGE('',*,*,#9115,.F.) ;
#13041=ORIENTED_EDGE('',*,*,#9116,.T.) ;
#13042=ORIENTED_EDGE('',*,*,#9117,.F.) ;
#13043=ORIENTED_EDGE('',*,*,#9118,.T.) ;
#13044=ORIENTED_EDGE('',*,*,#9119,.T.) ;
#13045=ORIENTED_EDGE('',*,*,#9120,.T.) ;
#13046=ORIENTED_EDGE('',*,*,#9121,.F.) ;
#13047=ORIENTED_EDGE('',*,*,#9122,.T.) ;
#13048=ORIENTED_EDGE('',*,*,#9123,.F.) ;
#13049=ORIENTED_EDGE('',*,*,#9124,.T.) ;
#13050=ORIENTED_EDGE('',*,*,#9125,.T.) ;
#13051=ORIENTED_EDGE('',*,*,#9126,.T.) ;
#13052=ORIENTED_EDGE('',*,*,#9127,.F.) ;
#13053=ORIENTED_EDGE('',*,*,#9128,.T.) ;
#13054=ORIENTED_EDGE('',*,*,#9129,.F.) ;
#13055=ORIENTED_EDGE('',*,*,#9130,.T.) ;
#13056=ORIENTED_EDGE('',*,*,#9131,.T.) ;
#13057=ORIENTED_EDGE('',*,*,#9132,.T.) ;
#13058=ORIENTED_EDGE('',*,*,#9133,.F.) ;
#13059=ORIENTED_EDGE('',*,*,#9134,.T.) ;
#13060=ORIENTED_EDGE('',*,*,#9135,.F.) ;
#13061=ORIENTED_EDGE('',*,*,#9136,.T.) ;
#13062=ORIENTED_EDGE('',*,*,#9137,.T.) ;
#13063=ORIENTED_EDGE('',*,*,#9138,.T.) ;
#13064=ORIENTED_EDGE('',*,*,#9139,.F.) ;
#13065=ORIENTED_EDGE('',*,*,#9140,.T.) ;
#13066=ORIENTED_EDGE('',*,*,#9141,.F.) ;
#13067=ORIENTED_EDGE('',*,*,#9142,.T.) ;
#13068=ORIENTED_EDGE('',*,*,#9143,.T.) ;
#13069=ORIENTED_EDGE('',*,*,#9144,.T.) ;
#13070=ORIENTED_EDGE('',*,*,#9145,.F.) ;
#13071=ORIENTED_EDGE('',*,*,#9146,.T.) ;
#13072=ORIENTED_EDGE('',*,*,#9147,.F.) ;
#13073=ORIENTED_EDGE('',*,*,#9148,.T.) ;
#13074=ORIENTED_EDGE('',*,*,#9149,.T.) ;
#13075=ORIENTED_EDGE('',*,*,#9150,.T.) ;
#13076=ORIENTED_EDGE('',*,*,#9151,.F.) ;
#13077=ORIENTED_EDGE('',*,*,#9152,.T.) ;
#13078=ORIENTED_EDGE('',*,*,#9153,.F.) ;
#13079=ORIENTED_EDGE('',*,*,#9154,.T.) ;
#13080=ORIENTED_EDGE('',*,*,#9155,.T.) ;
#13081=ORIENTED_EDGE('',*,*,#9156,.T.) ;
#13082=ORIENTED_EDGE('',*,*,#9157,.F.) ;
#13083=ORIENTED_EDGE('',*,*,#9158,.T.) ;
#13084=ORIENTED_EDGE('',*,*,#9159,.F.) ;
#13085=ORIENTED_EDGE('',*,*,#9160,.T.) ;
#13086=ORIENTED_EDGE('',*,*,#9161,.T.) ;
#13087=ORIENTED_EDGE('',*,*,#9162,.T.) ;
#13088=ORIENTED_EDGE('',*,*,#9163,.F.) ;
#13089=ORIENTED_EDGE('',*,*,#9164,.T.) ;
#13090=ORIENTED_EDGE('',*,*,#9165,.F.) ;
#13091=ORIENTED_EDGE('',*,*,#9166,.T.) ;
#13092=ORIENTED_EDGE('',*,*,#9167,.T.) ;
#13093=ORIENTED_EDGE('',*,*,#9168,.T.) ;
#13094=ORIENTED_EDGE('',*,*,#9169,.F.) ;
#13095=ORIENTED_EDGE('',*,*,#9170,.T.) ;
#13096=ORIENTED_EDGE('',*,*,#9171,.F.) ;
#13097=ORIENTED_EDGE('',*,*,#9172,.T.) ;
#13098=ORIENTED_EDGE('',*,*,#9173,.T.) ;
#13099=ORIENTED_EDGE('',*,*,#9174,.T.) ;
#13100=ORIENTED_EDGE('',*,*,#9175,.F.) ;
#13101=ORIENTED_EDGE('',*,*,#9176,.T.) ;
#13102=ORIENTED_EDGE('',*,*,#9177,.F.) ;
#13103=ORIENTED_EDGE('',*,*,#9178,.T.) ;
#13104=ORIENTED_EDGE('',*,*,#9179,.T.) ;
#13105=ORIENTED_EDGE('',*,*,#9180,.T.) ;
#13106=ORIENTED_EDGE('',*,*,#9181,.F.) ;
#13107=ORIENTED_EDGE('',*,*,#9182,.T.) ;
#13108=ORIENTED_EDGE('',*,*,#9183,.F.) ;
#13109=ORIENTED_EDGE('',*,*,#9184,.T.) ;
#13110=ORIENTED_EDGE('',*,*,#9185,.T.) ;
#13111=ORIENTED_EDGE('',*,*,#9186,.T.) ;
#13112=ORIENTED_EDGE('',*,*,#9187,.F.) ;
#13113=ORIENTED_EDGE('',*,*,#9188,.T.) ;
#13114=ORIENTED_EDGE('',*,*,#9189,.F.) ;
#13115=ORIENTED_EDGE('',*,*,#9190,.T.) ;
#13116=ORIENTED_EDGE('',*,*,#9191,.T.) ;
#13117=ORIENTED_EDGE('',*,*,#9192,.T.) ;
#13118=ORIENTED_EDGE('',*,*,#9193,.F.) ;
#13119=ORIENTED_EDGE('',*,*,#9194,.T.) ;
#13120=ORIENTED_EDGE('',*,*,#9195,.F.) ;
#13121=ORIENTED_EDGE('',*,*,#9196,.T.) ;
#13122=ORIENTED_EDGE('',*,*,#9197,.T.) ;
#13123=ORIENTED_EDGE('',*,*,#9198,.T.) ;
#13124=ORIENTED_EDGE('',*,*,#9199,.F.) ;
#13125=ORIENTED_EDGE('',*,*,#9200,.T.) ;
#13126=ORIENTED_EDGE('',*,*,#9201,.F.) ;
#13127=ORIENTED_EDGE('',*,*,#9202,.T.) ;
#13128=ORIENTED_EDGE('',*,*,#9203,.T.) ;
#13129=ORIENTED_EDGE('',*,*,#9204,.T.) ;
#13130=ORIENTED_EDGE('',*,*,#9205,.F.) ;
#13131=ORIENTED_EDGE('',*,*,#9206,.T.) ;
#13132=ORIENTED_EDGE('',*,*,#9207,.F.) ;
#13133=ORIENTED_EDGE('',*,*,#9208,.T.) ;
#13134=ORIENTED_EDGE('',*,*,#9209,.T.) ;
#13135=ORIENTED_EDGE('',*,*,#9034,.F.) ;
#13136=ORIENTED_EDGE('',*,*,#9033,.T.) ;
#13137=ORIENTED_EDGE('',*,*,#9210,.T.) ;
#13138=ORIENTED_EDGE('',*,*,#9211,.F.) ;
#13139=ORIENTED_EDGE('',*,*,#9212,.F.) ;
#13140=ORIENTED_EDGE('',*,*,#9213,.F.) ;
#13141=ORIENTED_EDGE('',*,*,#9214,.F.) ;
#13142=ORIENTED_EDGE('',*,*,#9215,.F.) ;
#13143=ORIENTED_EDGE('',*,*,#9216,.F.) ;
#13144=ORIENTED_EDGE('',*,*,#9217,.F.) ;
#13145=ORIENTED_EDGE('',*,*,#9218,.F.) ;
#13146=ORIENTED_EDGE('',*,*,#9219,.F.) ;
#13147=ORIENTED_EDGE('',*,*,#9220,.F.) ;
#13148=ORIENTED_EDGE('',*,*,#9221,.F.) ;
#13149=ORIENTED_EDGE('',*,*,#9222,.F.) ;
#13150=ORIENTED_EDGE('',*,*,#9223,.F.) ;
#13151=ORIENTED_EDGE('',*,*,#9224,.F.) ;
#13152=ORIENTED_EDGE('',*,*,#9225,.F.) ;
#13153=ORIENTED_EDGE('',*,*,#9226,.F.) ;
#13154=ORIENTED_EDGE('',*,*,#9227,.F.) ;
#13155=ORIENTED_EDGE('',*,*,#9228,.F.) ;
#13156=ORIENTED_EDGE('',*,*,#9229,.F.) ;
#13157=ORIENTED_EDGE('',*,*,#9230,.F.) ;
#13158=ORIENTED_EDGE('',*,*,#9231,.F.) ;
#13159=ORIENTED_EDGE('',*,*,#9232,.F.) ;
#13160=ORIENTED_EDGE('',*,*,#9233,.F.) ;
#13161=ORIENTED_EDGE('',*,*,#9234,.F.) ;
#13162=ORIENTED_EDGE('',*,*,#9235,.F.) ;
#13163=ORIENTED_EDGE('',*,*,#9236,.F.) ;
#13164=ORIENTED_EDGE('',*,*,#9237,.F.) ;
#13165=ORIENTED_EDGE('',*,*,#9238,.F.) ;
#13166=ORIENTED_EDGE('',*,*,#9239,.F.) ;
#13167=ORIENTED_EDGE('',*,*,#9240,.F.) ;
#13168=ORIENTED_EDGE('',*,*,#9241,.F.) ;
#13169=ORIENTED_EDGE('',*,*,#9242,.F.) ;
#13170=ORIENTED_EDGE('',*,*,#9243,.F.) ;
#13171=ORIENTED_EDGE('',*,*,#9244,.F.) ;
#13172=ORIENTED_EDGE('',*,*,#9245,.F.) ;
#13173=ORIENTED_EDGE('',*,*,#9246,.F.) ;
#13174=ORIENTED_EDGE('',*,*,#9247,.F.) ;
#13175=ORIENTED_EDGE('',*,*,#9248,.F.) ;
#13176=ORIENTED_EDGE('',*,*,#9249,.F.) ;
#13177=ORIENTED_EDGE('',*,*,#9250,.F.) ;
#13178=ORIENTED_EDGE('',*,*,#9251,.F.) ;
#13179=ORIENTED_EDGE('',*,*,#9252,.F.) ;
#13180=ORIENTED_EDGE('',*,*,#9253,.F.) ;
#13181=ORIENTED_EDGE('',*,*,#9254,.F.) ;
#13182=ORIENTED_EDGE('',*,*,#9255,.F.) ;
#13183=ORIENTED_EDGE('',*,*,#9256,.F.) ;
#13184=ORIENTED_EDGE('',*,*,#9257,.F.) ;
#13185=ORIENTED_EDGE('',*,*,#9258,.F.) ;
#13186=ORIENTED_EDGE('',*,*,#9259,.F.) ;
#13187=ORIENTED_EDGE('',*,*,#9260,.F.) ;
#13188=ORIENTED_EDGE('',*,*,#9261,.F.) ;
#13189=ORIENTED_EDGE('',*,*,#9262,.F.) ;
#13190=ORIENTED_EDGE('',*,*,#9263,.F.) ;
#13191=ORIENTED_EDGE('',*,*,#9264,.F.) ;
#13192=ORIENTED_EDGE('',*,*,#9265,.F.) ;
#13193=ORIENTED_EDGE('',*,*,#9266,.F.) ;
#13194=ORIENTED_EDGE('',*,*,#9267,.F.) ;
#13195=ORIENTED_EDGE('',*,*,#9268,.F.) ;
#13196=ORIENTED_EDGE('',*,*,#9269,.F.) ;
#13197=ORIENTED_EDGE('',*,*,#9270,.F.) ;
#13198=ORIENTED_EDGE('',*,*,#9271,.F.) ;
#13199=ORIENTED_EDGE('',*,*,#9272,.F.) ;
#13200=ORIENTED_EDGE('',*,*,#9273,.F.) ;
#13201=ORIENTED_EDGE('',*,*,#9274,.F.) ;
#13202=ORIENTED_EDGE('',*,*,#9275,.F.) ;
#13203=ORIENTED_EDGE('',*,*,#9276,.F.) ;
#13204=ORIENTED_EDGE('',*,*,#9277,.F.) ;
#13205=ORIENTED_EDGE('',*,*,#9278,.F.) ;
#13206=ORIENTED_EDGE('',*,*,#9279,.F.) ;
#13207=ORIENTED_EDGE('',*,*,#9280,.F.) ;
#13208=ORIENTED_EDGE('',*,*,#9281,.F.) ;
#13209=ORIENTED_EDGE('',*,*,#9282,.F.) ;
#13210=ORIENTED_EDGE('',*,*,#9283,.F.) ;
#13211=ORIENTED_EDGE('',*,*,#9284,.F.) ;
#13212=ORIENTED_EDGE('',*,*,#9285,.F.) ;
#13213=ORIENTED_EDGE('',*,*,#9286,.F.) ;
#13214=ORIENTED_EDGE('',*,*,#9287,.F.) ;
#13215=ORIENTED_EDGE('',*,*,#9288,.F.) ;
#13216=ORIENTED_EDGE('',*,*,#9289,.F.) ;
#13217=ORIENTED_EDGE('',*,*,#9290,.F.) ;
#13218=ORIENTED_EDGE('',*,*,#9291,.F.) ;
#13219=ORIENTED_EDGE('',*,*,#9292,.F.) ;
#13220=ORIENTED_EDGE('',*,*,#9293,.F.) ;
#13221=ORIENTED_EDGE('',*,*,#9294,.F.) ;
#13222=ORIENTED_EDGE('',*,*,#9295,.F.) ;
#13223=ORIENTED_EDGE('',*,*,#9296,.F.) ;
#13224=ORIENTED_EDGE('',*,*,#9297,.F.) ;
#13225=ORIENTED_EDGE('',*,*,#9298,.F.) ;
#13226=ORIENTED_EDGE('',*,*,#9299,.F.) ;
#13227=ORIENTED_EDGE('',*,*,#9300,.F.) ;
#13228=ORIENTED_EDGE('',*,*,#9301,.F.) ;
#13229=ORIENTED_EDGE('',*,*,#9302,.F.) ;
#13230=ORIENTED_EDGE('',*,*,#9303,.F.) ;
#13231=ORIENTED_EDGE('',*,*,#9304,.F.) ;
#13232=ORIENTED_EDGE('',*,*,#9305,.F.) ;
#13233=ORIENTED_EDGE('',*,*,#9306,.F.) ;
#13234=ORIENTED_EDGE('',*,*,#9307,.F.) ;
#13235=ORIENTED_EDGE('',*,*,#9308,.F.) ;
#13236=ORIENTED_EDGE('',*,*,#9309,.F.) ;
#13237=ORIENTED_EDGE('',*,*,#9310,.F.) ;
#13238=ORIENTED_EDGE('',*,*,#9311,.F.) ;
#13239=ORIENTED_EDGE('',*,*,#9312,.F.) ;
#13240=ORIENTED_EDGE('',*,*,#9313,.F.) ;
#13241=ORIENTED_EDGE('',*,*,#9314,.F.) ;
#13242=ORIENTED_EDGE('',*,*,#9315,.F.) ;
#13243=ORIENTED_EDGE('',*,*,#9316,.F.) ;
#13244=ORIENTED_EDGE('',*,*,#9317,.F.) ;
#13245=ORIENTED_EDGE('',*,*,#9318,.F.) ;
#13246=ORIENTED_EDGE('',*,*,#9319,.F.) ;
#13247=ORIENTED_EDGE('',*,*,#9320,.F.) ;
#13248=ORIENTED_EDGE('',*,*,#9321,.F.) ;
#13249=ORIENTED_EDGE('',*,*,#9210,.F.) ;
#13250=ORIENTED_EDGE('',*,*,#9322,.F.) ;
#13251=ORIENTED_EDGE('',*,*,#9323,.F.) ;
#13252=ORIENTED_EDGE('',*,*,#9324,.F.) ;
#13253=ORIENTED_EDGE('',*,*,#9325,.F.) ;
#13254=ORIENTED_EDGE('',*,*,#9326,.F.) ;
#13255=ORIENTED_EDGE('',*,*,#9327,.F.) ;
#13256=ORIENTED_EDGE('',*,*,#9209,.F.) ;
#13257=ORIENTED_EDGE('',*,*,#9328,.T.) ;
#13258=ORIENTED_EDGE('',*,*,#9329,.F.) ;
#13259=ORIENTED_EDGE('',*,*,#9206,.F.) ;
#13260=ORIENTED_EDGE('',*,*,#9330,.F.) ;
#13261=ORIENTED_EDGE('',*,*,#9331,.T.) ;
#13262=ORIENTED_EDGE('',*,*,#9203,.F.) ;
#13263=ORIENTED_EDGE('',*,*,#9332,.T.) ;
#13264=ORIENTED_EDGE('',*,*,#9333,.F.) ;
#13265=ORIENTED_EDGE('',*,*,#9200,.F.) ;
#13266=ORIENTED_EDGE('',*,*,#9334,.F.) ;
#13267=ORIENTED_EDGE('',*,*,#9335,.T.) ;
#13268=ORIENTED_EDGE('',*,*,#9197,.F.) ;
#13269=ORIENTED_EDGE('',*,*,#9336,.T.) ;
#13270=ORIENTED_EDGE('',*,*,#9337,.F.) ;
#13271=ORIENTED_EDGE('',*,*,#9194,.F.) ;
#13272=ORIENTED_EDGE('',*,*,#9338,.F.) ;
#13273=ORIENTED_EDGE('',*,*,#9339,.T.) ;
#13274=ORIENTED_EDGE('',*,*,#9191,.F.) ;
#13275=ORIENTED_EDGE('',*,*,#9340,.T.) ;
#13276=ORIENTED_EDGE('',*,*,#9341,.F.) ;
#13277=ORIENTED_EDGE('',*,*,#9188,.F.) ;
#13278=ORIENTED_EDGE('',*,*,#9342,.F.) ;
#13279=ORIENTED_EDGE('',*,*,#9343,.T.) ;
#13280=ORIENTED_EDGE('',*,*,#9185,.F.) ;
#13281=ORIENTED_EDGE('',*,*,#9344,.T.) ;
#13282=ORIENTED_EDGE('',*,*,#9345,.F.) ;
#13283=ORIENTED_EDGE('',*,*,#9182,.F.) ;
#13284=ORIENTED_EDGE('',*,*,#9346,.F.) ;
#13285=ORIENTED_EDGE('',*,*,#9347,.T.) ;
#13286=ORIENTED_EDGE('',*,*,#9179,.F.) ;
#13287=ORIENTED_EDGE('',*,*,#9348,.T.) ;
#13288=ORIENTED_EDGE('',*,*,#9349,.F.) ;
#13289=ORIENTED_EDGE('',*,*,#9176,.F.) ;
#13290=ORIENTED_EDGE('',*,*,#9350,.F.) ;
#13291=ORIENTED_EDGE('',*,*,#9351,.T.) ;
#13292=ORIENTED_EDGE('',*,*,#9173,.F.) ;
#13293=ORIENTED_EDGE('',*,*,#9352,.T.) ;
#13294=ORIENTED_EDGE('',*,*,#9353,.F.) ;
#13295=ORIENTED_EDGE('',*,*,#9170,.F.) ;
#13296=ORIENTED_EDGE('',*,*,#9354,.F.) ;
#13297=ORIENTED_EDGE('',*,*,#9355,.T.) ;
#13298=ORIENTED_EDGE('',*,*,#9167,.F.) ;
#13299=ORIENTED_EDGE('',*,*,#9356,.T.) ;
#13300=ORIENTED_EDGE('',*,*,#9357,.F.) ;
#13301=ORIENTED_EDGE('',*,*,#9164,.F.) ;
#13302=ORIENTED_EDGE('',*,*,#9358,.F.) ;
#13303=ORIENTED_EDGE('',*,*,#9359,.T.) ;
#13304=ORIENTED_EDGE('',*,*,#9161,.F.) ;
#13305=ORIENTED_EDGE('',*,*,#9360,.T.) ;
#13306=ORIENTED_EDGE('',*,*,#9361,.F.) ;
#13307=ORIENTED_EDGE('',*,*,#9158,.F.) ;
#13308=ORIENTED_EDGE('',*,*,#9362,.F.) ;
#13309=ORIENTED_EDGE('',*,*,#9363,.T.) ;
#13310=ORIENTED_EDGE('',*,*,#9155,.F.) ;
#13311=ORIENTED_EDGE('',*,*,#9364,.T.) ;
#13312=ORIENTED_EDGE('',*,*,#9365,.F.) ;
#13313=ORIENTED_EDGE('',*,*,#9152,.F.) ;
#13314=ORIENTED_EDGE('',*,*,#9366,.F.) ;
#13315=ORIENTED_EDGE('',*,*,#9367,.T.) ;
#13316=ORIENTED_EDGE('',*,*,#9149,.F.) ;
#13317=ORIENTED_EDGE('',*,*,#9368,.T.) ;
#13318=ORIENTED_EDGE('',*,*,#9369,.F.) ;
#13319=ORIENTED_EDGE('',*,*,#9146,.F.) ;
#13320=ORIENTED_EDGE('',*,*,#9370,.F.) ;
#13321=ORIENTED_EDGE('',*,*,#9371,.T.) ;
#13322=ORIENTED_EDGE('',*,*,#9143,.F.) ;
#13323=ORIENTED_EDGE('',*,*,#9372,.T.) ;
#13324=ORIENTED_EDGE('',*,*,#9373,.F.) ;
#13325=ORIENTED_EDGE('',*,*,#9140,.F.) ;
#13326=ORIENTED_EDGE('',*,*,#9374,.F.) ;
#13327=ORIENTED_EDGE('',*,*,#9375,.T.) ;
#13328=ORIENTED_EDGE('',*,*,#9137,.F.) ;
#13329=ORIENTED_EDGE('',*,*,#9376,.T.) ;
#13330=ORIENTED_EDGE('',*,*,#9377,.F.) ;
#13331=ORIENTED_EDGE('',*,*,#9134,.F.) ;
#13332=ORIENTED_EDGE('',*,*,#9378,.F.) ;
#13333=ORIENTED_EDGE('',*,*,#9379,.T.) ;
#13334=ORIENTED_EDGE('',*,*,#9131,.F.) ;
#13335=ORIENTED_EDGE('',*,*,#9380,.T.) ;
#13336=ORIENTED_EDGE('',*,*,#9381,.F.) ;
#13337=ORIENTED_EDGE('',*,*,#9128,.F.) ;
#13338=ORIENTED_EDGE('',*,*,#9382,.F.) ;
#13339=ORIENTED_EDGE('',*,*,#9383,.T.) ;
#13340=ORIENTED_EDGE('',*,*,#9125,.F.) ;
#13341=ORIENTED_EDGE('',*,*,#9384,.T.) ;
#13342=ORIENTED_EDGE('',*,*,#9385,.F.) ;
#13343=ORIENTED_EDGE('',*,*,#9122,.F.) ;
#13344=ORIENTED_EDGE('',*,*,#9386,.F.) ;
#13345=ORIENTED_EDGE('',*,*,#9387,.T.) ;
#13346=ORIENTED_EDGE('',*,*,#9119,.F.) ;
#13347=ORIENTED_EDGE('',*,*,#9388,.T.) ;
#13348=ORIENTED_EDGE('',*,*,#9389,.F.) ;
#13349=ORIENTED_EDGE('',*,*,#9116,.F.) ;
#13350=ORIENTED_EDGE('',*,*,#9390,.F.) ;
#13351=ORIENTED_EDGE('',*,*,#9391,.T.) ;
#13352=ORIENTED_EDGE('',*,*,#9113,.F.) ;
#13353=ORIENTED_EDGE('',*,*,#9392,.T.) ;
#13354=ORIENTED_EDGE('',*,*,#9393,.F.) ;
#13355=ORIENTED_EDGE('',*,*,#9110,.F.) ;
#13356=ORIENTED_EDGE('',*,*,#9394,.F.) ;
#13357=ORIENTED_EDGE('',*,*,#9395,.T.) ;
#13358=ORIENTED_EDGE('',*,*,#9107,.F.) ;
#13359=ORIENTED_EDGE('',*,*,#9396,.T.) ;
#13360=ORIENTED_EDGE('',*,*,#9397,.F.) ;
#13361=ORIENTED_EDGE('',*,*,#9104,.F.) ;
#13362=ORIENTED_EDGE('',*,*,#9398,.F.) ;
#13363=ORIENTED_EDGE('',*,*,#9399,.T.) ;
#13364=ORIENTED_EDGE('',*,*,#9101,.F.) ;
#13365=ORIENTED_EDGE('',*,*,#9400,.T.) ;
#13366=ORIENTED_EDGE('',*,*,#9401,.F.) ;
#13367=ORIENTED_EDGE('',*,*,#9098,.F.) ;
#13368=ORIENTED_EDGE('',*,*,#9402,.F.) ;
#13369=ORIENTED_EDGE('',*,*,#9403,.T.) ;
#13370=ORIENTED_EDGE('',*,*,#9095,.F.) ;
#13371=ORIENTED_EDGE('',*,*,#9404,.T.) ;
#13372=ORIENTED_EDGE('',*,*,#9405,.F.) ;
#13373=ORIENTED_EDGE('',*,*,#9092,.F.) ;
#13374=ORIENTED_EDGE('',*,*,#9406,.F.) ;
#13375=ORIENTED_EDGE('',*,*,#9407,.T.) ;
#13376=ORIENTED_EDGE('',*,*,#9089,.F.) ;
#13377=ORIENTED_EDGE('',*,*,#9408,.T.) ;
#13378=ORIENTED_EDGE('',*,*,#9409,.F.) ;
#13379=ORIENTED_EDGE('',*,*,#9086,.F.) ;
#13380=ORIENTED_EDGE('',*,*,#9410,.F.) ;
#13381=ORIENTED_EDGE('',*,*,#9411,.T.) ;
#13382=ORIENTED_EDGE('',*,*,#9083,.F.) ;
#13383=ORIENTED_EDGE('',*,*,#9412,.T.) ;
#13384=ORIENTED_EDGE('',*,*,#9413,.F.) ;
#13385=ORIENTED_EDGE('',*,*,#9080,.F.) ;
#13386=ORIENTED_EDGE('',*,*,#9414,.F.) ;
#13387=ORIENTED_EDGE('',*,*,#9415,.T.) ;
#13388=ORIENTED_EDGE('',*,*,#9077,.F.) ;
#13389=ORIENTED_EDGE('',*,*,#9416,.T.) ;
#13390=ORIENTED_EDGE('',*,*,#9417,.F.) ;
#13391=ORIENTED_EDGE('',*,*,#9074,.F.) ;
#13392=ORIENTED_EDGE('',*,*,#9418,.F.) ;
#13393=ORIENTED_EDGE('',*,*,#9419,.T.) ;
#13394=ORIENTED_EDGE('',*,*,#9071,.F.) ;
#13395=ORIENTED_EDGE('',*,*,#9420,.T.) ;
#13396=ORIENTED_EDGE('',*,*,#9421,.F.) ;
#13397=ORIENTED_EDGE('',*,*,#9068,.F.) ;
#13398=ORIENTED_EDGE('',*,*,#9422,.F.) ;
#13399=ORIENTED_EDGE('',*,*,#9423,.T.) ;
#13400=ORIENTED_EDGE('',*,*,#9065,.F.) ;
#13401=ORIENTED_EDGE('',*,*,#9424,.T.) ;
#13402=ORIENTED_EDGE('',*,*,#9425,.F.) ;
#13403=ORIENTED_EDGE('',*,*,#9062,.F.) ;
#13404=ORIENTED_EDGE('',*,*,#9426,.F.) ;
#13405=ORIENTED_EDGE('',*,*,#9427,.T.) ;
#13406=ORIENTED_EDGE('',*,*,#9059,.F.) ;
#13407=ORIENTED_EDGE('',*,*,#9428,.T.) ;
#13408=ORIENTED_EDGE('',*,*,#9429,.F.) ;
#13409=ORIENTED_EDGE('',*,*,#9056,.F.) ;
#13410=ORIENTED_EDGE('',*,*,#9430,.F.) ;
#13411=ORIENTED_EDGE('',*,*,#9431,.T.) ;
#13412=ORIENTED_EDGE('',*,*,#9053,.F.) ;
#13413=ORIENTED_EDGE('',*,*,#9432,.T.) ;
#13414=ORIENTED_EDGE('',*,*,#9433,.F.) ;
#13415=ORIENTED_EDGE('',*,*,#9050,.F.) ;
#13416=ORIENTED_EDGE('',*,*,#9434,.F.) ;
#13417=ORIENTED_EDGE('',*,*,#9435,.T.) ;
#13418=ORIENTED_EDGE('',*,*,#9047,.F.) ;
#13419=ORIENTED_EDGE('',*,*,#9436,.T.) ;
#13420=ORIENTED_EDGE('',*,*,#9437,.F.) ;
#13421=ORIENTED_EDGE('',*,*,#9044,.F.) ;
#13422=ORIENTED_EDGE('',*,*,#9438,.F.) ;
#13423=ORIENTED_EDGE('',*,*,#9439,.T.) ;
#13424=ORIENTED_EDGE('',*,*,#9041,.F.) ;
#13425=ORIENTED_EDGE('',*,*,#9440,.T.) ;
#13426=ORIENTED_EDGE('',*,*,#9441,.F.) ;
#13427=ORIENTED_EDGE('',*,*,#9038,.F.) ;
#13428=ORIENTED_EDGE('',*,*,#9442,.F.) ;
#13429=ORIENTED_EDGE('',*,*,#9443,.T.) ;
#13430=ORIENTED_EDGE('',*,*,#9035,.F.) ;
#13431=ORIENTED_EDGE('',*,*,#9444,.T.) ;
#13432=ORIENTED_EDGE('',*,*,#9445,.T.) ;
#13433=ORIENTED_EDGE('',*,*,#9444,.F.) ;
#13434=ORIENTED_EDGE('',*,*,#9446,.T.) ;
#13435=ORIENTED_EDGE('',*,*,#9447,.T.) ;
#13436=ORIENTED_EDGE('',*,*,#9448,.F.) ;
#13437=ORIENTED_EDGE('',*,*,#9447,.F.) ;
#13438=ORIENTED_EDGE('',*,*,#9449,.F.) ;
#13439=ORIENTED_EDGE('',*,*,#9450,.F.) ;
#13440=ORIENTED_EDGE('',*,*,#9451,.F.) ;
#13441=ORIENTED_EDGE('',*,*,#9452,.F.) ;
#13442=ORIENTED_EDGE('',*,*,#9453,.F.) ;
#13443=ORIENTED_EDGE('',*,*,#9454,.F.) ;
#13444=ORIENTED_EDGE('',*,*,#9455,.F.) ;
#13445=ORIENTED_EDGE('',*,*,#9456,.F.) ;
#13446=ORIENTED_EDGE('',*,*,#9457,.F.) ;
#13447=ORIENTED_EDGE('',*,*,#9458,.F.) ;
#13448=ORIENTED_EDGE('',*,*,#9459,.F.) ;
#13449=ORIENTED_EDGE('',*,*,#9460,.F.) ;
#13450=ORIENTED_EDGE('',*,*,#9461,.F.) ;
#13451=ORIENTED_EDGE('',*,*,#9462,.F.) ;
#13452=ORIENTED_EDGE('',*,*,#9463,.F.) ;
#13453=ORIENTED_EDGE('',*,*,#9464,.F.) ;
#13454=ORIENTED_EDGE('',*,*,#9465,.F.) ;
#13455=ORIENTED_EDGE('',*,*,#9466,.F.) ;
#13456=ORIENTED_EDGE('',*,*,#9467,.F.) ;
#13457=ORIENTED_EDGE('',*,*,#9468,.F.) ;
#13458=ORIENTED_EDGE('',*,*,#9469,.F.) ;
#13459=ORIENTED_EDGE('',*,*,#9470,.F.) ;
#13460=ORIENTED_EDGE('',*,*,#9471,.F.) ;
#13461=ORIENTED_EDGE('',*,*,#9472,.F.) ;
#13462=ORIENTED_EDGE('',*,*,#9473,.F.) ;
#13463=ORIENTED_EDGE('',*,*,#9474,.F.) ;
#13464=ORIENTED_EDGE('',*,*,#9475,.F.) ;
#13465=ORIENTED_EDGE('',*,*,#9476,.F.) ;
#13466=ORIENTED_EDGE('',*,*,#9477,.F.) ;
#13467=ORIENTED_EDGE('',*,*,#9478,.F.) ;
#13468=ORIENTED_EDGE('',*,*,#9479,.F.) ;
#13469=ORIENTED_EDGE('',*,*,#9480,.F.) ;
#13470=ORIENTED_EDGE('',*,*,#9481,.F.) ;
#13471=ORIENTED_EDGE('',*,*,#9482,.F.) ;
#13472=ORIENTED_EDGE('',*,*,#9483,.F.) ;
#13473=ORIENTED_EDGE('',*,*,#9484,.F.) ;
#13474=ORIENTED_EDGE('',*,*,#9485,.F.) ;
#13475=ORIENTED_EDGE('',*,*,#9486,.F.) ;
#13476=ORIENTED_EDGE('',*,*,#9487,.F.) ;
#13477=ORIENTED_EDGE('',*,*,#9488,.F.) ;
#13478=ORIENTED_EDGE('',*,*,#9489,.F.) ;
#13479=ORIENTED_EDGE('',*,*,#9490,.F.) ;
#13480=ORIENTED_EDGE('',*,*,#9491,.F.) ;
#13481=ORIENTED_EDGE('',*,*,#9492,.F.) ;
#13482=ORIENTED_EDGE('',*,*,#9493,.F.) ;
#13483=ORIENTED_EDGE('',*,*,#9494,.F.) ;
#13484=ORIENTED_EDGE('',*,*,#9495,.F.) ;
#13485=ORIENTED_EDGE('',*,*,#9496,.F.) ;
#13486=ORIENTED_EDGE('',*,*,#9497,.F.) ;
#13487=ORIENTED_EDGE('',*,*,#9498,.F.) ;
#13488=ORIENTED_EDGE('',*,*,#9499,.F.) ;
#13489=ORIENTED_EDGE('',*,*,#9500,.F.) ;
#13490=ORIENTED_EDGE('',*,*,#9501,.F.) ;
#13491=ORIENTED_EDGE('',*,*,#9502,.F.) ;
#13492=ORIENTED_EDGE('',*,*,#9503,.F.) ;
#13493=ORIENTED_EDGE('',*,*,#9504,.F.) ;
#13494=ORIENTED_EDGE('',*,*,#9505,.F.) ;
#13495=ORIENTED_EDGE('',*,*,#9506,.F.) ;
#13496=ORIENTED_EDGE('',*,*,#9507,.F.) ;
#13497=ORIENTED_EDGE('',*,*,#9508,.F.) ;
#13498=ORIENTED_EDGE('',*,*,#9509,.F.) ;
#13499=ORIENTED_EDGE('',*,*,#9510,.F.) ;
#13500=ORIENTED_EDGE('',*,*,#9511,.F.) ;
#13501=ORIENTED_EDGE('',*,*,#9512,.F.) ;
#13502=ORIENTED_EDGE('',*,*,#9513,.F.) ;
#13503=ORIENTED_EDGE('',*,*,#9514,.F.) ;
#13504=ORIENTED_EDGE('',*,*,#9515,.F.) ;
#13505=ORIENTED_EDGE('',*,*,#9516,.F.) ;
#13506=ORIENTED_EDGE('',*,*,#9517,.F.) ;
#13507=ORIENTED_EDGE('',*,*,#9518,.F.) ;
#13508=ORIENTED_EDGE('',*,*,#9519,.F.) ;
#13509=ORIENTED_EDGE('',*,*,#9520,.F.) ;
#13510=ORIENTED_EDGE('',*,*,#9521,.F.) ;
#13511=ORIENTED_EDGE('',*,*,#9522,.F.) ;
#13512=ORIENTED_EDGE('',*,*,#9523,.F.) ;
#13513=ORIENTED_EDGE('',*,*,#9524,.F.) ;
#13514=ORIENTED_EDGE('',*,*,#9525,.F.) ;
#13515=ORIENTED_EDGE('',*,*,#9526,.F.) ;
#13516=ORIENTED_EDGE('',*,*,#9527,.F.) ;
#13517=ORIENTED_EDGE('',*,*,#9528,.F.) ;
#13518=ORIENTED_EDGE('',*,*,#9529,.F.) ;
#13519=ORIENTED_EDGE('',*,*,#9530,.F.) ;
#13520=ORIENTED_EDGE('',*,*,#9531,.F.) ;
#13521=ORIENTED_EDGE('',*,*,#9532,.F.) ;
#13522=ORIENTED_EDGE('',*,*,#9533,.F.) ;
#13523=ORIENTED_EDGE('',*,*,#9534,.F.) ;
#13524=ORIENTED_EDGE('',*,*,#9535,.F.) ;
#13525=ORIENTED_EDGE('',*,*,#9536,.F.) ;
#13526=ORIENTED_EDGE('',*,*,#9537,.T.) ;
#13527=ORIENTED_EDGE('',*,*,#9538,.T.) ;
#13528=ORIENTED_EDGE('',*,*,#9537,.F.) ;
#13529=ORIENTED_EDGE('',*,*,#9539,.F.) ;
#13530=ORIENTED_EDGE('',*,*,#9540,.T.) ;
#13531=ORIENTED_EDGE('',*,*,#9541,.T.) ;
#13532=ORIENTED_EDGE('',*,*,#9540,.F.) ;
#13533=ORIENTED_EDGE('',*,*,#9542,.F.) ;
#13534=ORIENTED_EDGE('',*,*,#9543,.T.) ;
#13535=ORIENTED_EDGE('',*,*,#9544,.T.) ;
#13536=ORIENTED_EDGE('',*,*,#9543,.F.) ;
#13537=ORIENTED_EDGE('',*,*,#9545,.F.) ;
#13538=ORIENTED_EDGE('',*,*,#9546,.T.) ;
#13539=ORIENTED_EDGE('',*,*,#9547,.T.) ;
#13540=ORIENTED_EDGE('',*,*,#9546,.F.) ;
#13541=ORIENTED_EDGE('',*,*,#9541,.F.) ;
#13542=ORIENTED_EDGE('',*,*,#9548,.T.) ;
#13543=ORIENTED_EDGE('',*,*,#9549,.T.) ;
#13544=ORIENTED_EDGE('',*,*,#9548,.F.) ;
#13545=ORIENTED_EDGE('',*,*,#9549,.F.) ;
#13546=ORIENTED_EDGE('',*,*,#9550,.T.) ;
#13547=ORIENTED_EDGE('',*,*,#9551,.T.) ;
#13548=ORIENTED_EDGE('',*,*,#9550,.F.) ;
#13549=ORIENTED_EDGE('',*,*,#9544,.F.) ;
#13550=ORIENTED_EDGE('',*,*,#9552,.T.) ;
#13551=ORIENTED_EDGE('',*,*,#9545,.T.) ;
#13552=ORIENTED_EDGE('',*,*,#9552,.F.) ;
#13553=ORIENTED_EDGE('',*,*,#9536,.T.) ;
#13554=ORIENTED_EDGE('',*,*,#9551,.F.) ;
#13555=ORIENTED_EDGE('',*,*,#9547,.F.) ;
#13556=ORIENTED_EDGE('',*,*,#9448,.T.) ;
#13557=ORIENTED_EDGE('',*,*,#9542,.T.) ;
#13558=ORIENTED_EDGE('',*,*,#9446,.F.) ;
#13559=ORIENTED_EDGE('',*,*,#9553,.T.) ;
#13560=ORIENTED_EDGE('',*,*,#9554,.T.) ;
#13561=ORIENTED_EDGE('',*,*,#9555,.T.) ;
#13562=ORIENTED_EDGE('',*,*,#9556,.T.) ;
#13563=ORIENTED_EDGE('',*,*,#9557,.T.) ;
#13564=ORIENTED_EDGE('',*,*,#9558,.T.) ;
#13565=ORIENTED_EDGE('',*,*,#9559,.T.) ;
#13566=ORIENTED_EDGE('',*,*,#9560,.T.) ;
#13567=ORIENTED_EDGE('',*,*,#9561,.T.) ;
#13568=ORIENTED_EDGE('',*,*,#9562,.T.) ;
#13569=ORIENTED_EDGE('',*,*,#9563,.T.) ;
#13570=ORIENTED_EDGE('',*,*,#9564,.T.) ;
#13571=ORIENTED_EDGE('',*,*,#9565,.T.) ;
#13572=ORIENTED_EDGE('',*,*,#9566,.T.) ;
#13573=ORIENTED_EDGE('',*,*,#9567,.T.) ;
#13574=ORIENTED_EDGE('',*,*,#9568,.T.) ;
#13575=ORIENTED_EDGE('',*,*,#9569,.T.) ;
#13576=ORIENTED_EDGE('',*,*,#9570,.T.) ;
#13577=ORIENTED_EDGE('',*,*,#9571,.T.) ;
#13578=ORIENTED_EDGE('',*,*,#9572,.T.) ;
#13579=ORIENTED_EDGE('',*,*,#9573,.T.) ;
#13580=ORIENTED_EDGE('',*,*,#9574,.T.) ;
#13581=ORIENTED_EDGE('',*,*,#9575,.T.) ;
#13582=ORIENTED_EDGE('',*,*,#9576,.T.) ;
#13583=ORIENTED_EDGE('',*,*,#9577,.T.) ;
#13584=ORIENTED_EDGE('',*,*,#9578,.T.) ;
#13585=ORIENTED_EDGE('',*,*,#9579,.T.) ;
#13586=ORIENTED_EDGE('',*,*,#9580,.T.) ;
#13587=ORIENTED_EDGE('',*,*,#9581,.T.) ;
#13588=ORIENTED_EDGE('',*,*,#9582,.T.) ;
#13589=ORIENTED_EDGE('',*,*,#9583,.T.) ;
#13590=ORIENTED_EDGE('',*,*,#9584,.T.) ;
#13591=ORIENTED_EDGE('',*,*,#9585,.T.) ;
#13592=ORIENTED_EDGE('',*,*,#9586,.T.) ;
#13593=ORIENTED_EDGE('',*,*,#9587,.T.) ;
#13594=ORIENTED_EDGE('',*,*,#9588,.T.) ;
#13595=ORIENTED_EDGE('',*,*,#9589,.T.) ;
#13596=ORIENTED_EDGE('',*,*,#9590,.T.) ;
#13597=ORIENTED_EDGE('',*,*,#9591,.T.) ;
#13598=ORIENTED_EDGE('',*,*,#9592,.T.) ;
#13599=ORIENTED_EDGE('',*,*,#9593,.T.) ;
#13600=ORIENTED_EDGE('',*,*,#9594,.T.) ;
#13601=ORIENTED_EDGE('',*,*,#9595,.T.) ;
#13602=ORIENTED_EDGE('',*,*,#9596,.T.) ;
#13603=ORIENTED_EDGE('',*,*,#9597,.T.) ;
#13604=ORIENTED_EDGE('',*,*,#9598,.T.) ;
#13605=ORIENTED_EDGE('',*,*,#9599,.T.) ;
#13606=ORIENTED_EDGE('',*,*,#9600,.T.) ;
#13607=ORIENTED_EDGE('',*,*,#9601,.T.) ;
#13608=ORIENTED_EDGE('',*,*,#9602,.T.) ;
#13609=ORIENTED_EDGE('',*,*,#9603,.T.) ;
#13610=ORIENTED_EDGE('',*,*,#9604,.T.) ;
#13611=ORIENTED_EDGE('',*,*,#9605,.T.) ;
#13612=ORIENTED_EDGE('',*,*,#9606,.T.) ;
#13613=ORIENTED_EDGE('',*,*,#9607,.T.) ;
#13614=ORIENTED_EDGE('',*,*,#9608,.T.) ;
#13615=ORIENTED_EDGE('',*,*,#9445,.F.) ;
#13616=ORIENTED_EDGE('',*,*,#9539,.T.) ;
#13617=ORIENTED_EDGE('',*,*,#9609,.T.) ;
#13618=ORIENTED_EDGE('',*,*,#9610,.T.) ;
#13619=ORIENTED_EDGE('',*,*,#9538,.F.) ;
#13620=ORIENTED_EDGE('',*,*,#9611,.T.) ;
#13621=ORIENTED_EDGE('',*,*,#9321,.T.) ;
#13622=ORIENTED_EDGE('',*,*,#9317,.T.) ;
#13623=ORIENTED_EDGE('',*,*,#9313,.T.) ;
#13624=ORIENTED_EDGE('',*,*,#9309,.T.) ;
#13625=ORIENTED_EDGE('',*,*,#9305,.T.) ;
#13626=ORIENTED_EDGE('',*,*,#9301,.T.) ;
#13627=ORIENTED_EDGE('',*,*,#9297,.T.) ;
#13628=ORIENTED_EDGE('',*,*,#9293,.T.) ;
#13629=ORIENTED_EDGE('',*,*,#9289,.T.) ;
#13630=ORIENTED_EDGE('',*,*,#9285,.T.) ;
#13631=ORIENTED_EDGE('',*,*,#9281,.T.) ;
#13632=ORIENTED_EDGE('',*,*,#9277,.T.) ;
#13633=ORIENTED_EDGE('',*,*,#9273,.T.) ;
#13634=ORIENTED_EDGE('',*,*,#9269,.T.) ;
#13635=ORIENTED_EDGE('',*,*,#9265,.T.) ;
#13636=ORIENTED_EDGE('',*,*,#9261,.T.) ;
#13637=ORIENTED_EDGE('',*,*,#9260,.T.) ;
#13638=ORIENTED_EDGE('',*,*,#9256,.T.) ;
#13639=ORIENTED_EDGE('',*,*,#9252,.T.) ;
#13640=ORIENTED_EDGE('',*,*,#9248,.T.) ;
#13641=ORIENTED_EDGE('',*,*,#9244,.T.) ;
#13642=ORIENTED_EDGE('',*,*,#9243,.T.) ;
#13643=ORIENTED_EDGE('',*,*,#9239,.T.) ;
#13644=ORIENTED_EDGE('',*,*,#9235,.T.) ;
#13645=ORIENTED_EDGE('',*,*,#9231,.T.) ;
#13646=ORIENTED_EDGE('',*,*,#9227,.T.) ;
#13647=ORIENTED_EDGE('',*,*,#9223,.T.) ;
#13648=ORIENTED_EDGE('',*,*,#9219,.T.) ;
#13649=ORIENTED_EDGE('',*,*,#9215,.T.) ;
#13650=ORIENTED_EDGE('',*,*,#9211,.T.) ;
#13651=ORIENTED_EDGE('',*,*,#9611,.F.) ;
#13652=ORIENTED_EDGE('',*,*,#9124,.F.) ;
#13653=ORIENTED_EDGE('',*,*,#9612,.T.) ;
#13654=ORIENTED_EDGE('',*,*,#9262,.T.) ;
#13655=ORIENTED_EDGE('',*,*,#9553,.F.) ;
#13656=ORIENTED_EDGE('',*,*,#9451,.T.) ;
#13657=ORIENTED_EDGE('',*,*,#9613,.T.) ;
#13658=ORIENTED_EDGE('',*,*,#9384,.F.) ;
#13659=ORIENTED_EDGE('',*,*,#9121,.T.) ;
#13660=ORIENTED_EDGE('',*,*,#9614,.F.) ;
#13661=ORIENTED_EDGE('',*,*,#9263,.T.) ;
#13662=ORIENTED_EDGE('',*,*,#9612,.F.) ;
#13663=ORIENTED_EDGE('',*,*,#9123,.T.) ;
#13664=ORIENTED_EDGE('',*,*,#9385,.T.) ;
#13665=ORIENTED_EDGE('',*,*,#9613,.F.) ;
#13666=ORIENTED_EDGE('',*,*,#9450,.T.) ;
#13667=ORIENTED_EDGE('',*,*,#9615,.F.) ;
#13668=ORIENTED_EDGE('',*,*,#9386,.T.) ;
#13669=ORIENTED_EDGE('',*,*,#9120,.F.) ;
#13670=ORIENTED_EDGE('',*,*,#9387,.F.) ;
#13671=ORIENTED_EDGE('',*,*,#9615,.T.) ;
#13672=ORIENTED_EDGE('',*,*,#9449,.T.) ;
#13673=ORIENTED_EDGE('',*,*,#9554,.F.) ;
#13674=ORIENTED_EDGE('',*,*,#9264,.T.) ;
#13675=ORIENTED_EDGE('',*,*,#9614,.T.) ;
#13676=ORIENTED_EDGE('',*,*,#9118,.F.) ;
#13677=ORIENTED_EDGE('',*,*,#9616,.T.) ;
#13678=ORIENTED_EDGE('',*,*,#9266,.T.) ;
#13679=ORIENTED_EDGE('',*,*,#9555,.F.) ;
#13680=ORIENTED_EDGE('',*,*,#9534,.T.) ;
#13681=ORIENTED_EDGE('',*,*,#9617,.T.) ;
#13682=ORIENTED_EDGE('',*,*,#9388,.F.) ;
#13683=ORIENTED_EDGE('',*,*,#9115,.T.) ;
#13684=ORIENTED_EDGE('',*,*,#9618,.F.) ;
#13685=ORIENTED_EDGE('',*,*,#9267,.T.) ;
#13686=ORIENTED_EDGE('',*,*,#9616,.F.) ;
#13687=ORIENTED_EDGE('',*,*,#9117,.T.) ;
#13688=ORIENTED_EDGE('',*,*,#9389,.T.) ;
#13689=ORIENTED_EDGE('',*,*,#9617,.F.) ;
#13690=ORIENTED_EDGE('',*,*,#9533,.T.) ;
#13691=ORIENTED_EDGE('',*,*,#9619,.F.) ;
#13692=ORIENTED_EDGE('',*,*,#9390,.T.) ;
#13693=ORIENTED_EDGE('',*,*,#9114,.F.) ;
#13694=ORIENTED_EDGE('',*,*,#9391,.F.) ;
#13695=ORIENTED_EDGE('',*,*,#9619,.T.) ;
#13696=ORIENTED_EDGE('',*,*,#9535,.T.) ;
#13697=ORIENTED_EDGE('',*,*,#9556,.F.) ;
#13698=ORIENTED_EDGE('',*,*,#9268,.T.) ;
#13699=ORIENTED_EDGE('',*,*,#9618,.T.) ;
#13700=ORIENTED_EDGE('',*,*,#9112,.F.) ;
#13701=ORIENTED_EDGE('',*,*,#9620,.T.) ;
#13702=ORIENTED_EDGE('',*,*,#9270,.T.) ;
#13703=ORIENTED_EDGE('',*,*,#9557,.F.) ;
#13704=ORIENTED_EDGE('',*,*,#9495,.T.) ;
#13705=ORIENTED_EDGE('',*,*,#9621,.T.) ;
#13706=ORIENTED_EDGE('',*,*,#9392,.F.) ;
#13707=ORIENTED_EDGE('',*,*,#9109,.T.) ;
#13708=ORIENTED_EDGE('',*,*,#9622,.F.) ;
#13709=ORIENTED_EDGE('',*,*,#9271,.T.) ;
#13710=ORIENTED_EDGE('',*,*,#9620,.F.) ;
#13711=ORIENTED_EDGE('',*,*,#9111,.T.) ;
#13712=ORIENTED_EDGE('',*,*,#9393,.T.) ;
#13713=ORIENTED_EDGE('',*,*,#9621,.F.) ;
#13714=ORIENTED_EDGE('',*,*,#9494,.T.) ;
#13715=ORIENTED_EDGE('',*,*,#9623,.F.) ;
#13716=ORIENTED_EDGE('',*,*,#9394,.T.) ;
#13717=ORIENTED_EDGE('',*,*,#9108,.F.) ;
#13718=ORIENTED_EDGE('',*,*,#9395,.F.) ;
#13719=ORIENTED_EDGE('',*,*,#9623,.T.) ;
#13720=ORIENTED_EDGE('',*,*,#9496,.T.) ;
#13721=ORIENTED_EDGE('',*,*,#9558,.F.) ;
#13722=ORIENTED_EDGE('',*,*,#9272,.T.) ;
#13723=ORIENTED_EDGE('',*,*,#9622,.T.) ;
#13724=ORIENTED_EDGE('',*,*,#9106,.F.) ;
#13725=ORIENTED_EDGE('',*,*,#9624,.T.) ;
#13726=ORIENTED_EDGE('',*,*,#9274,.T.) ;
#13727=ORIENTED_EDGE('',*,*,#9559,.F.) ;
#13728=ORIENTED_EDGE('',*,*,#9531,.T.) ;
#13729=ORIENTED_EDGE('',*,*,#9625,.T.) ;
#13730=ORIENTED_EDGE('',*,*,#9396,.F.) ;
#13731=ORIENTED_EDGE('',*,*,#9103,.T.) ;
#13732=ORIENTED_EDGE('',*,*,#9626,.F.) ;
#13733=ORIENTED_EDGE('',*,*,#9275,.T.) ;
#13734=ORIENTED_EDGE('',*,*,#9624,.F.) ;
#13735=ORIENTED_EDGE('',*,*,#9105,.T.) ;
#13736=ORIENTED_EDGE('',*,*,#9397,.T.) ;
#13737=ORIENTED_EDGE('',*,*,#9625,.F.) ;
#13738=ORIENTED_EDGE('',*,*,#9530,.T.) ;
#13739=ORIENTED_EDGE('',*,*,#9627,.F.) ;
#13740=ORIENTED_EDGE('',*,*,#9398,.T.) ;
#13741=ORIENTED_EDGE('',*,*,#9102,.F.) ;
#13742=ORIENTED_EDGE('',*,*,#9399,.F.) ;
#13743=ORIENTED_EDGE('',*,*,#9627,.T.) ;
#13744=ORIENTED_EDGE('',*,*,#9532,.T.) ;
#13745=ORIENTED_EDGE('',*,*,#9560,.F.) ;
#13746=ORIENTED_EDGE('',*,*,#9276,.T.) ;
#13747=ORIENTED_EDGE('',*,*,#9626,.T.) ;
#13748=ORIENTED_EDGE('',*,*,#9100,.F.) ;
#13749=ORIENTED_EDGE('',*,*,#9628,.T.) ;
#13750=ORIENTED_EDGE('',*,*,#9278,.T.) ;
#13751=ORIENTED_EDGE('',*,*,#9561,.F.) ;
#13752=ORIENTED_EDGE('',*,*,#9498,.T.) ;
#13753=ORIENTED_EDGE('',*,*,#9629,.T.) ;
#13754=ORIENTED_EDGE('',*,*,#9400,.F.) ;
#13755=ORIENTED_EDGE('',*,*,#9097,.T.) ;
#13756=ORIENTED_EDGE('',*,*,#9630,.F.) ;
#13757=ORIENTED_EDGE('',*,*,#9279,.T.) ;
#13758=ORIENTED_EDGE('',*,*,#9628,.F.) ;
#13759=ORIENTED_EDGE('',*,*,#9099,.T.) ;
#13760=ORIENTED_EDGE('',*,*,#9401,.T.) ;
#13761=ORIENTED_EDGE('',*,*,#9629,.F.) ;
#13762=ORIENTED_EDGE('',*,*,#9497,.T.) ;
#13763=ORIENTED_EDGE('',*,*,#9631,.F.) ;
#13764=ORIENTED_EDGE('',*,*,#9402,.T.) ;
#13765=ORIENTED_EDGE('',*,*,#9096,.F.) ;
#13766=ORIENTED_EDGE('',*,*,#9403,.F.) ;
#13767=ORIENTED_EDGE('',*,*,#9631,.T.) ;
#13768=ORIENTED_EDGE('',*,*,#9499,.T.) ;
#13769=ORIENTED_EDGE('',*,*,#9562,.F.) ;
#13770=ORIENTED_EDGE('',*,*,#9280,.T.) ;
#13771=ORIENTED_EDGE('',*,*,#9630,.T.) ;
#13772=ORIENTED_EDGE('',*,*,#9094,.F.) ;
#13773=ORIENTED_EDGE('',*,*,#9632,.T.) ;
#13774=ORIENTED_EDGE('',*,*,#9282,.T.) ;
#13775=ORIENTED_EDGE('',*,*,#9563,.F.) ;
#13776=ORIENTED_EDGE('',*,*,#9528,.T.) ;
#13777=ORIENTED_EDGE('',*,*,#9633,.T.) ;
#13778=ORIENTED_EDGE('',*,*,#9404,.F.) ;
#13779=ORIENTED_EDGE('',*,*,#9091,.T.) ;
#13780=ORIENTED_EDGE('',*,*,#9634,.F.) ;
#13781=ORIENTED_EDGE('',*,*,#9283,.T.) ;
#13782=ORIENTED_EDGE('',*,*,#9632,.F.) ;
#13783=ORIENTED_EDGE('',*,*,#9093,.T.) ;
#13784=ORIENTED_EDGE('',*,*,#9405,.T.) ;
#13785=ORIENTED_EDGE('',*,*,#9633,.F.) ;
#13786=ORIENTED_EDGE('',*,*,#9527,.T.) ;
#13787=ORIENTED_EDGE('',*,*,#9635,.F.) ;
#13788=ORIENTED_EDGE('',*,*,#9406,.T.) ;
#13789=ORIENTED_EDGE('',*,*,#9090,.F.) ;
#13790=ORIENTED_EDGE('',*,*,#9407,.F.) ;
#13791=ORIENTED_EDGE('',*,*,#9635,.T.) ;
#13792=ORIENTED_EDGE('',*,*,#9529,.T.) ;
#13793=ORIENTED_EDGE('',*,*,#9564,.F.) ;
#13794=ORIENTED_EDGE('',*,*,#9284,.T.) ;
#13795=ORIENTED_EDGE('',*,*,#9634,.T.) ;
#13796=ORIENTED_EDGE('',*,*,#9088,.F.) ;
#13797=ORIENTED_EDGE('',*,*,#9636,.T.) ;
#13798=ORIENTED_EDGE('',*,*,#9286,.T.) ;
#13799=ORIENTED_EDGE('',*,*,#9565,.F.) ;
#13800=ORIENTED_EDGE('',*,*,#9501,.T.) ;
#13801=ORIENTED_EDGE('',*,*,#9637,.T.) ;
#13802=ORIENTED_EDGE('',*,*,#9408,.F.) ;
#13803=ORIENTED_EDGE('',*,*,#9085,.T.) ;
#13804=ORIENTED_EDGE('',*,*,#9638,.F.) ;
#13805=ORIENTED_EDGE('',*,*,#9287,.T.) ;
#13806=ORIENTED_EDGE('',*,*,#9636,.F.) ;
#13807=ORIENTED_EDGE('',*,*,#9087,.T.) ;
#13808=ORIENTED_EDGE('',*,*,#9409,.T.) ;
#13809=ORIENTED_EDGE('',*,*,#9637,.F.) ;
#13810=ORIENTED_EDGE('',*,*,#9500,.T.) ;
#13811=ORIENTED_EDGE('',*,*,#9639,.F.) ;
#13812=ORIENTED_EDGE('',*,*,#9410,.T.) ;
#13813=ORIENTED_EDGE('',*,*,#9084,.F.) ;
#13814=ORIENTED_EDGE('',*,*,#9411,.F.) ;
#13815=ORIENTED_EDGE('',*,*,#9639,.T.) ;
#13816=ORIENTED_EDGE('',*,*,#9502,.T.) ;
#13817=ORIENTED_EDGE('',*,*,#9566,.F.) ;
#13818=ORIENTED_EDGE('',*,*,#9288,.T.) ;
#13819=ORIENTED_EDGE('',*,*,#9638,.T.) ;
#13820=ORIENTED_EDGE('',*,*,#9082,.F.) ;
#13821=ORIENTED_EDGE('',*,*,#9640,.T.) ;
#13822=ORIENTED_EDGE('',*,*,#9290,.T.) ;
#13823=ORIENTED_EDGE('',*,*,#9567,.F.) ;
#13824=ORIENTED_EDGE('',*,*,#9525,.T.) ;
#13825=ORIENTED_EDGE('',*,*,#9641,.T.) ;
#13826=ORIENTED_EDGE('',*,*,#9412,.F.) ;
#13827=ORIENTED_EDGE('',*,*,#9079,.T.) ;
#13828=ORIENTED_EDGE('',*,*,#9642,.F.) ;
#13829=ORIENTED_EDGE('',*,*,#9291,.T.) ;
#13830=ORIENTED_EDGE('',*,*,#9640,.F.) ;
#13831=ORIENTED_EDGE('',*,*,#9081,.T.) ;
#13832=ORIENTED_EDGE('',*,*,#9413,.T.) ;
#13833=ORIENTED_EDGE('',*,*,#9641,.F.) ;
#13834=ORIENTED_EDGE('',*,*,#9524,.T.) ;
#13835=ORIENTED_EDGE('',*,*,#9643,.F.) ;
#13836=ORIENTED_EDGE('',*,*,#9414,.T.) ;
#13837=ORIENTED_EDGE('',*,*,#9078,.F.) ;
#13838=ORIENTED_EDGE('',*,*,#9415,.F.) ;
#13839=ORIENTED_EDGE('',*,*,#9643,.T.) ;
#13840=ORIENTED_EDGE('',*,*,#9526,.T.) ;
#13841=ORIENTED_EDGE('',*,*,#9568,.F.) ;
#13842=ORIENTED_EDGE('',*,*,#9292,.T.) ;
#13843=ORIENTED_EDGE('',*,*,#9642,.T.) ;
#13844=ORIENTED_EDGE('',*,*,#9076,.F.) ;
#13845=ORIENTED_EDGE('',*,*,#9644,.T.) ;
#13846=ORIENTED_EDGE('',*,*,#9294,.T.) ;
#13847=ORIENTED_EDGE('',*,*,#9569,.F.) ;
#13848=ORIENTED_EDGE('',*,*,#9504,.T.) ;
#13849=ORIENTED_EDGE('',*,*,#9645,.T.) ;
#13850=ORIENTED_EDGE('',*,*,#9416,.F.) ;
#13851=ORIENTED_EDGE('',*,*,#9075,.T.) ;
#13852=ORIENTED_EDGE('',*,*,#9417,.T.) ;
#13853=ORIENTED_EDGE('',*,*,#9645,.F.) ;
#13854=ORIENTED_EDGE('',*,*,#9503,.T.) ;
#13855=ORIENTED_EDGE('',*,*,#9646,.F.) ;
#13856=ORIENTED_EDGE('',*,*,#9418,.T.) ;
#13857=ORIENTED_EDGE('',*,*,#9073,.T.) ;
#13858=ORIENTED_EDGE('',*,*,#9647,.F.) ;
#13859=ORIENTED_EDGE('',*,*,#9295,.T.) ;
#13860=ORIENTED_EDGE('',*,*,#9644,.F.) ;
#13861=ORIENTED_EDGE('',*,*,#9072,.F.) ;
#13862=ORIENTED_EDGE('',*,*,#9419,.F.) ;
#13863=ORIENTED_EDGE('',*,*,#9646,.T.) ;
#13864=ORIENTED_EDGE('',*,*,#9505,.T.) ;
#13865=ORIENTED_EDGE('',*,*,#9570,.F.) ;
#13866=ORIENTED_EDGE('',*,*,#9296,.T.) ;
#13867=ORIENTED_EDGE('',*,*,#9647,.T.) ;
#13868=ORIENTED_EDGE('',*,*,#9070,.F.) ;
#13869=ORIENTED_EDGE('',*,*,#9648,.T.) ;
#13870=ORIENTED_EDGE('',*,*,#9298,.T.) ;
#13871=ORIENTED_EDGE('',*,*,#9571,.F.) ;
#13872=ORIENTED_EDGE('',*,*,#9522,.T.) ;
#13873=ORIENTED_EDGE('',*,*,#9649,.T.) ;
#13874=ORIENTED_EDGE('',*,*,#9420,.F.) ;
#13875=ORIENTED_EDGE('',*,*,#9069,.T.) ;
#13876=ORIENTED_EDGE('',*,*,#9421,.T.) ;
#13877=ORIENTED_EDGE('',*,*,#9649,.F.) ;
#13878=ORIENTED_EDGE('',*,*,#9521,.T.) ;
#13879=ORIENTED_EDGE('',*,*,#9650,.F.) ;
#13880=ORIENTED_EDGE('',*,*,#9422,.T.) ;
#13881=ORIENTED_EDGE('',*,*,#9067,.T.) ;
#13882=ORIENTED_EDGE('',*,*,#9651,.F.) ;
#13883=ORIENTED_EDGE('',*,*,#9299,.T.) ;
#13884=ORIENTED_EDGE('',*,*,#9648,.F.) ;
#13885=ORIENTED_EDGE('',*,*,#9066,.F.) ;
#13886=ORIENTED_EDGE('',*,*,#9423,.F.) ;
#13887=ORIENTED_EDGE('',*,*,#9650,.T.) ;
#13888=ORIENTED_EDGE('',*,*,#9523,.T.) ;
#13889=ORIENTED_EDGE('',*,*,#9572,.F.) ;
#13890=ORIENTED_EDGE('',*,*,#9300,.T.) ;
#13891=ORIENTED_EDGE('',*,*,#9651,.T.) ;
#13892=ORIENTED_EDGE('',*,*,#9064,.F.) ;
#13893=ORIENTED_EDGE('',*,*,#9652,.T.) ;
#13894=ORIENTED_EDGE('',*,*,#9302,.T.) ;
#13895=ORIENTED_EDGE('',*,*,#9573,.F.) ;
#13896=ORIENTED_EDGE('',*,*,#9507,.T.) ;
#13897=ORIENTED_EDGE('',*,*,#9653,.T.) ;
#13898=ORIENTED_EDGE('',*,*,#9424,.F.) ;
#13899=ORIENTED_EDGE('',*,*,#9063,.T.) ;
#13900=ORIENTED_EDGE('',*,*,#9425,.T.) ;
#13901=ORIENTED_EDGE('',*,*,#9653,.F.) ;
#13902=ORIENTED_EDGE('',*,*,#9506,.T.) ;
#13903=ORIENTED_EDGE('',*,*,#9654,.F.) ;
#13904=ORIENTED_EDGE('',*,*,#9426,.T.) ;
#13905=ORIENTED_EDGE('',*,*,#9061,.T.) ;
#13906=ORIENTED_EDGE('',*,*,#9655,.F.) ;
#13907=ORIENTED_EDGE('',*,*,#9303,.T.) ;
#13908=ORIENTED_EDGE('',*,*,#9652,.F.) ;
#13909=ORIENTED_EDGE('',*,*,#9060,.F.) ;
#13910=ORIENTED_EDGE('',*,*,#9427,.F.) ;
#13911=ORIENTED_EDGE('',*,*,#9654,.T.) ;
#13912=ORIENTED_EDGE('',*,*,#9508,.T.) ;
#13913=ORIENTED_EDGE('',*,*,#9574,.F.) ;
#13914=ORIENTED_EDGE('',*,*,#9304,.T.) ;
#13915=ORIENTED_EDGE('',*,*,#9655,.T.) ;
#13916=ORIENTED_EDGE('',*,*,#9058,.F.) ;
#13917=ORIENTED_EDGE('',*,*,#9656,.T.) ;
#13918=ORIENTED_EDGE('',*,*,#9306,.T.) ;
#13919=ORIENTED_EDGE('',*,*,#9575,.F.) ;
#13920=ORIENTED_EDGE('',*,*,#9519,.T.) ;
#13921=ORIENTED_EDGE('',*,*,#9657,.T.) ;
#13922=ORIENTED_EDGE('',*,*,#9428,.F.) ;
#13923=ORIENTED_EDGE('',*,*,#9057,.T.) ;
#13924=ORIENTED_EDGE('',*,*,#9429,.T.) ;
#13925=ORIENTED_EDGE('',*,*,#9657,.F.) ;
#13926=ORIENTED_EDGE('',*,*,#9518,.T.) ;
#13927=ORIENTED_EDGE('',*,*,#9658,.F.) ;
#13928=ORIENTED_EDGE('',*,*,#9430,.T.) ;
#13929=ORIENTED_EDGE('',*,*,#9055,.T.) ;
#13930=ORIENTED_EDGE('',*,*,#9659,.F.) ;
#13931=ORIENTED_EDGE('',*,*,#9307,.T.) ;
#13932=ORIENTED_EDGE('',*,*,#9656,.F.) ;
#13933=ORIENTED_EDGE('',*,*,#9054,.F.) ;
#13934=ORIENTED_EDGE('',*,*,#9431,.F.) ;
#13935=ORIENTED_EDGE('',*,*,#9658,.T.) ;
#13936=ORIENTED_EDGE('',*,*,#9520,.T.) ;
#13937=ORIENTED_EDGE('',*,*,#9576,.F.) ;
#13938=ORIENTED_EDGE('',*,*,#9308,.T.) ;
#13939=ORIENTED_EDGE('',*,*,#9659,.T.) ;
#13940=ORIENTED_EDGE('',*,*,#9052,.F.) ;
#13941=ORIENTED_EDGE('',*,*,#9660,.T.) ;
#13942=ORIENTED_EDGE('',*,*,#9310,.T.) ;
#13943=ORIENTED_EDGE('',*,*,#9577,.F.) ;
#13944=ORIENTED_EDGE('',*,*,#9510,.T.) ;
#13945=ORIENTED_EDGE('',*,*,#9661,.T.) ;
#13946=ORIENTED_EDGE('',*,*,#9432,.F.) ;
#13947=ORIENTED_EDGE('',*,*,#9051,.T.) ;
#13948=ORIENTED_EDGE('',*,*,#9433,.T.) ;
#13949=ORIENTED_EDGE('',*,*,#9661,.F.) ;
#13950=ORIENTED_EDGE('',*,*,#9509,.T.) ;
#13951=ORIENTED_EDGE('',*,*,#9662,.F.) ;
#13952=ORIENTED_EDGE('',*,*,#9434,.T.) ;
#13953=ORIENTED_EDGE('',*,*,#9049,.T.) ;
#13954=ORIENTED_EDGE('',*,*,#9663,.F.) ;
#13955=ORIENTED_EDGE('',*,*,#9311,.T.) ;
#13956=ORIENTED_EDGE('',*,*,#9660,.F.) ;
#13957=ORIENTED_EDGE('',*,*,#9048,.F.) ;
#13958=ORIENTED_EDGE('',*,*,#9435,.F.) ;
#13959=ORIENTED_EDGE('',*,*,#9662,.T.) ;
#13960=ORIENTED_EDGE('',*,*,#9511,.T.) ;
#13961=ORIENTED_EDGE('',*,*,#9578,.F.) ;
#13962=ORIENTED_EDGE('',*,*,#9312,.T.) ;
#13963=ORIENTED_EDGE('',*,*,#9663,.T.) ;
#13964=ORIENTED_EDGE('',*,*,#9046,.F.) ;
#13965=ORIENTED_EDGE('',*,*,#9664,.T.) ;
#13966=ORIENTED_EDGE('',*,*,#9314,.T.) ;
#13967=ORIENTED_EDGE('',*,*,#9579,.F.) ;
#13968=ORIENTED_EDGE('',*,*,#9516,.T.) ;
#13969=ORIENTED_EDGE('',*,*,#9665,.T.) ;
#13970=ORIENTED_EDGE('',*,*,#9436,.F.) ;
#13971=ORIENTED_EDGE('',*,*,#9045,.T.) ;
#13972=ORIENTED_EDGE('',*,*,#9437,.T.) ;
#13973=ORIENTED_EDGE('',*,*,#9665,.F.) ;
#13974=ORIENTED_EDGE('',*,*,#9515,.T.) ;
#13975=ORIENTED_EDGE('',*,*,#9666,.F.) ;
#13976=ORIENTED_EDGE('',*,*,#9438,.T.) ;
#13977=ORIENTED_EDGE('',*,*,#9043,.T.) ;
#13978=ORIENTED_EDGE('',*,*,#9667,.F.) ;
#13979=ORIENTED_EDGE('',*,*,#9315,.T.) ;
#13980=ORIENTED_EDGE('',*,*,#9664,.F.) ;
#13981=ORIENTED_EDGE('',*,*,#9042,.F.) ;
#13982=ORIENTED_EDGE('',*,*,#9439,.F.) ;
#13983=ORIENTED_EDGE('',*,*,#9666,.T.) ;
#13984=ORIENTED_EDGE('',*,*,#9517,.T.) ;
#13985=ORIENTED_EDGE('',*,*,#9580,.F.) ;
#13986=ORIENTED_EDGE('',*,*,#9316,.T.) ;
#13987=ORIENTED_EDGE('',*,*,#9667,.T.) ;
#13988=ORIENTED_EDGE('',*,*,#9040,.F.) ;
#13989=ORIENTED_EDGE('',*,*,#9668,.T.) ;
#13990=ORIENTED_EDGE('',*,*,#9318,.T.) ;
#13991=ORIENTED_EDGE('',*,*,#9581,.F.) ;
#13992=ORIENTED_EDGE('',*,*,#9513,.T.) ;
#13993=ORIENTED_EDGE('',*,*,#9669,.T.) ;
#13994=ORIENTED_EDGE('',*,*,#9440,.F.) ;
#13995=ORIENTED_EDGE('',*,*,#9039,.T.) ;
#13996=ORIENTED_EDGE('',*,*,#9441,.T.) ;
#13997=ORIENTED_EDGE('',*,*,#9669,.F.) ;
#13998=ORIENTED_EDGE('',*,*,#9512,.T.) ;
#13999=ORIENTED_EDGE('',*,*,#9670,.F.) ;
#14000=ORIENTED_EDGE('',*,*,#9442,.T.) ;
#14001=ORIENTED_EDGE('',*,*,#9037,.T.) ;
#14002=ORIENTED_EDGE('',*,*,#9671,.F.) ;
#14003=ORIENTED_EDGE('',*,*,#9319,.T.) ;
#14004=ORIENTED_EDGE('',*,*,#9668,.F.) ;
#14005=ORIENTED_EDGE('',*,*,#9036,.F.) ;
#14006=ORIENTED_EDGE('',*,*,#9443,.F.) ;
#14007=ORIENTED_EDGE('',*,*,#9670,.T.) ;
#14008=ORIENTED_EDGE('',*,*,#9514,.T.) ;
#14009=ORIENTED_EDGE('',*,*,#9582,.F.) ;
#14010=ORIENTED_EDGE('',*,*,#9320,.T.) ;
#14011=ORIENTED_EDGE('',*,*,#9671,.T.) ;
#14012=ORIENTED_EDGE('',*,*,#9208,.F.) ;
#14013=ORIENTED_EDGE('',*,*,#9672,.T.) ;
#14014=ORIENTED_EDGE('',*,*,#9212,.T.) ;
#14015=ORIENTED_EDGE('',*,*,#9583,.F.) ;
#14016=ORIENTED_EDGE('',*,*,#9471,.T.) ;
#14017=ORIENTED_EDGE('',*,*,#9673,.T.) ;
#14018=ORIENTED_EDGE('',*,*,#9328,.F.) ;
#14019=ORIENTED_EDGE('',*,*,#9207,.T.) ;
#14020=ORIENTED_EDGE('',*,*,#9329,.T.) ;
#14021=ORIENTED_EDGE('',*,*,#9673,.F.) ;
#14022=ORIENTED_EDGE('',*,*,#9470,.T.) ;
#14023=ORIENTED_EDGE('',*,*,#9674,.F.) ;
#14024=ORIENTED_EDGE('',*,*,#9330,.T.) ;
#14025=ORIENTED_EDGE('',*,*,#9205,.T.) ;
#14026=ORIENTED_EDGE('',*,*,#9675,.F.) ;
#14027=ORIENTED_EDGE('',*,*,#9213,.T.) ;
#14028=ORIENTED_EDGE('',*,*,#9672,.F.) ;
#14029=ORIENTED_EDGE('',*,*,#9204,.F.) ;
#14030=ORIENTED_EDGE('',*,*,#9331,.F.) ;
#14031=ORIENTED_EDGE('',*,*,#9674,.T.) ;
#14032=ORIENTED_EDGE('',*,*,#9472,.T.) ;
#14033=ORIENTED_EDGE('',*,*,#9584,.F.) ;
#14034=ORIENTED_EDGE('',*,*,#9214,.T.) ;
#14035=ORIENTED_EDGE('',*,*,#9675,.T.) ;
#14036=ORIENTED_EDGE('',*,*,#9202,.F.) ;
#14037=ORIENTED_EDGE('',*,*,#9676,.T.) ;
#14038=ORIENTED_EDGE('',*,*,#9216,.T.) ;
#14039=ORIENTED_EDGE('',*,*,#9585,.F.) ;
#14040=ORIENTED_EDGE('',*,*,#9474,.T.) ;
#14041=ORIENTED_EDGE('',*,*,#9677,.T.) ;
#14042=ORIENTED_EDGE('',*,*,#9332,.F.) ;
#14043=ORIENTED_EDGE('',*,*,#9201,.T.) ;
#14044=ORIENTED_EDGE('',*,*,#9333,.T.) ;
#14045=ORIENTED_EDGE('',*,*,#9677,.F.) ;
#14046=ORIENTED_EDGE('',*,*,#9473,.T.) ;
#14047=ORIENTED_EDGE('',*,*,#9678,.F.) ;
#14048=ORIENTED_EDGE('',*,*,#9334,.T.) ;
#14049=ORIENTED_EDGE('',*,*,#9199,.T.) ;
#14050=ORIENTED_EDGE('',*,*,#9679,.F.) ;
#14051=ORIENTED_EDGE('',*,*,#9217,.T.) ;
#14052=ORIENTED_EDGE('',*,*,#9676,.F.) ;
#14053=ORIENTED_EDGE('',*,*,#9198,.F.) ;
#14054=ORIENTED_EDGE('',*,*,#9335,.F.) ;
#14055=ORIENTED_EDGE('',*,*,#9678,.T.) ;
#14056=ORIENTED_EDGE('',*,*,#9475,.T.) ;
#14057=ORIENTED_EDGE('',*,*,#9586,.F.) ;
#14058=ORIENTED_EDGE('',*,*,#9218,.T.) ;
#14059=ORIENTED_EDGE('',*,*,#9679,.T.) ;
#14060=ORIENTED_EDGE('',*,*,#9196,.F.) ;
#14061=ORIENTED_EDGE('',*,*,#9680,.T.) ;
#14062=ORIENTED_EDGE('',*,*,#9220,.T.) ;
#14063=ORIENTED_EDGE('',*,*,#9587,.F.) ;
#14064=ORIENTED_EDGE('',*,*,#9468,.T.) ;
#14065=ORIENTED_EDGE('',*,*,#9681,.T.) ;
#14066=ORIENTED_EDGE('',*,*,#9336,.F.) ;
#14067=ORIENTED_EDGE('',*,*,#9195,.T.) ;
#14068=ORIENTED_EDGE('',*,*,#9337,.T.) ;
#14069=ORIENTED_EDGE('',*,*,#9681,.F.) ;
#14070=ORIENTED_EDGE('',*,*,#9467,.T.) ;
#14071=ORIENTED_EDGE('',*,*,#9682,.F.) ;
#14072=ORIENTED_EDGE('',*,*,#9338,.T.) ;
#14073=ORIENTED_EDGE('',*,*,#9193,.T.) ;
#14074=ORIENTED_EDGE('',*,*,#9683,.F.) ;
#14075=ORIENTED_EDGE('',*,*,#9221,.T.) ;
#14076=ORIENTED_EDGE('',*,*,#9680,.F.) ;
#14077=ORIENTED_EDGE('',*,*,#9192,.F.) ;
#14078=ORIENTED_EDGE('',*,*,#9339,.F.) ;
#14079=ORIENTED_EDGE('',*,*,#9682,.T.) ;
#14080=ORIENTED_EDGE('',*,*,#9469,.T.) ;
#14081=ORIENTED_EDGE('',*,*,#9588,.F.) ;
#14082=ORIENTED_EDGE('',*,*,#9222,.T.) ;
#14083=ORIENTED_EDGE('',*,*,#9683,.T.) ;
#14084=ORIENTED_EDGE('',*,*,#9190,.F.) ;
#14085=ORIENTED_EDGE('',*,*,#9684,.T.) ;
#14086=ORIENTED_EDGE('',*,*,#9224,.T.) ;
#14087=ORIENTED_EDGE('',*,*,#9589,.F.) ;
#14088=ORIENTED_EDGE('',*,*,#9477,.T.) ;
#14089=ORIENTED_EDGE('',*,*,#9685,.T.) ;
#14090=ORIENTED_EDGE('',*,*,#9340,.F.) ;
#14091=ORIENTED_EDGE('',*,*,#9189,.T.) ;
#14092=ORIENTED_EDGE('',*,*,#9341,.T.) ;
#14093=ORIENTED_EDGE('',*,*,#9685,.F.) ;
#14094=ORIENTED_EDGE('',*,*,#9476,.T.) ;
#14095=ORIENTED_EDGE('',*,*,#9686,.F.) ;
#14096=ORIENTED_EDGE('',*,*,#9342,.T.) ;
#14097=ORIENTED_EDGE('',*,*,#9187,.T.) ;
#14098=ORIENTED_EDGE('',*,*,#9687,.F.) ;
#14099=ORIENTED_EDGE('',*,*,#9225,.T.) ;
#14100=ORIENTED_EDGE('',*,*,#9684,.F.) ;
#14101=ORIENTED_EDGE('',*,*,#9186,.F.) ;
#14102=ORIENTED_EDGE('',*,*,#9343,.F.) ;
#14103=ORIENTED_EDGE('',*,*,#9686,.T.) ;
#14104=ORIENTED_EDGE('',*,*,#9478,.T.) ;
#14105=ORIENTED_EDGE('',*,*,#9590,.F.) ;
#14106=ORIENTED_EDGE('',*,*,#9226,.T.) ;
#14107=ORIENTED_EDGE('',*,*,#9687,.T.) ;
#14108=ORIENTED_EDGE('',*,*,#9184,.F.) ;
#14109=ORIENTED_EDGE('',*,*,#9688,.T.) ;
#14110=ORIENTED_EDGE('',*,*,#9228,.T.) ;
#14111=ORIENTED_EDGE('',*,*,#9591,.F.) ;
#14112=ORIENTED_EDGE('',*,*,#9465,.T.) ;
#14113=ORIENTED_EDGE('',*,*,#9689,.T.) ;
#14114=ORIENTED_EDGE('',*,*,#9344,.F.) ;
#14115=ORIENTED_EDGE('',*,*,#9183,.T.) ;
#14116=ORIENTED_EDGE('',*,*,#9345,.T.) ;
#14117=ORIENTED_EDGE('',*,*,#9689,.F.) ;
#14118=ORIENTED_EDGE('',*,*,#9464,.T.) ;
#14119=ORIENTED_EDGE('',*,*,#9690,.F.) ;
#14120=ORIENTED_EDGE('',*,*,#9346,.T.) ;
#14121=ORIENTED_EDGE('',*,*,#9181,.T.) ;
#14122=ORIENTED_EDGE('',*,*,#9691,.F.) ;
#14123=ORIENTED_EDGE('',*,*,#9229,.T.) ;
#14124=ORIENTED_EDGE('',*,*,#9688,.F.) ;
#14125=ORIENTED_EDGE('',*,*,#9180,.F.) ;
#14126=ORIENTED_EDGE('',*,*,#9347,.F.) ;
#14127=ORIENTED_EDGE('',*,*,#9690,.T.) ;
#14128=ORIENTED_EDGE('',*,*,#9466,.T.) ;
#14129=ORIENTED_EDGE('',*,*,#9592,.F.) ;
#14130=ORIENTED_EDGE('',*,*,#9230,.T.) ;
#14131=ORIENTED_EDGE('',*,*,#9691,.T.) ;
#14132=ORIENTED_EDGE('',*,*,#9178,.F.) ;
#14133=ORIENTED_EDGE('',*,*,#9692,.T.) ;
#14134=ORIENTED_EDGE('',*,*,#9232,.T.) ;
#14135=ORIENTED_EDGE('',*,*,#9593,.F.) ;
#14136=ORIENTED_EDGE('',*,*,#9480,.T.) ;
#14137=ORIENTED_EDGE('',*,*,#9693,.T.) ;
#14138=ORIENTED_EDGE('',*,*,#9348,.F.) ;
#14139=ORIENTED_EDGE('',*,*,#9177,.T.) ;
#14140=ORIENTED_EDGE('',*,*,#9349,.T.) ;
#14141=ORIENTED_EDGE('',*,*,#9693,.F.) ;
#14142=ORIENTED_EDGE('',*,*,#9479,.T.) ;
#14143=ORIENTED_EDGE('',*,*,#9694,.F.) ;
#14144=ORIENTED_EDGE('',*,*,#9350,.T.) ;
#14145=ORIENTED_EDGE('',*,*,#9175,.T.) ;
#14146=ORIENTED_EDGE('',*,*,#9695,.F.) ;
#14147=ORIENTED_EDGE('',*,*,#9233,.T.) ;
#14148=ORIENTED_EDGE('',*,*,#9692,.F.) ;
#14149=ORIENTED_EDGE('',*,*,#9174,.F.) ;
#14150=ORIENTED_EDGE('',*,*,#9351,.F.) ;
#14151=ORIENTED_EDGE('',*,*,#9694,.T.) ;
#14152=ORIENTED_EDGE('',*,*,#9481,.T.) ;
#14153=ORIENTED_EDGE('',*,*,#9594,.F.) ;
#14154=ORIENTED_EDGE('',*,*,#9234,.T.) ;
#14155=ORIENTED_EDGE('',*,*,#9695,.T.) ;
#14156=ORIENTED_EDGE('',*,*,#9172,.F.) ;
#14157=ORIENTED_EDGE('',*,*,#9696,.T.) ;
#14158=ORIENTED_EDGE('',*,*,#9236,.T.) ;
#14159=ORIENTED_EDGE('',*,*,#9595,.F.) ;
#14160=ORIENTED_EDGE('',*,*,#9462,.T.) ;
#14161=ORIENTED_EDGE('',*,*,#9697,.T.) ;
#14162=ORIENTED_EDGE('',*,*,#9352,.F.) ;
#14163=ORIENTED_EDGE('',*,*,#9171,.T.) ;
#14164=ORIENTED_EDGE('',*,*,#9353,.T.) ;
#14165=ORIENTED_EDGE('',*,*,#9697,.F.) ;
#14166=ORIENTED_EDGE('',*,*,#9461,.T.) ;
#14167=ORIENTED_EDGE('',*,*,#9698,.F.) ;
#14168=ORIENTED_EDGE('',*,*,#9354,.T.) ;
#14169=ORIENTED_EDGE('',*,*,#9169,.T.) ;
#14170=ORIENTED_EDGE('',*,*,#9699,.F.) ;
#14171=ORIENTED_EDGE('',*,*,#9237,.T.) ;
#14172=ORIENTED_EDGE('',*,*,#9696,.F.) ;
#14173=ORIENTED_EDGE('',*,*,#9168,.F.) ;
#14174=ORIENTED_EDGE('',*,*,#9355,.F.) ;
#14175=ORIENTED_EDGE('',*,*,#9698,.T.) ;
#14176=ORIENTED_EDGE('',*,*,#9463,.T.) ;
#14177=ORIENTED_EDGE('',*,*,#9596,.F.) ;
#14178=ORIENTED_EDGE('',*,*,#9238,.T.) ;
#14179=ORIENTED_EDGE('',*,*,#9699,.T.) ;
#14180=ORIENTED_EDGE('',*,*,#9166,.F.) ;
#14181=ORIENTED_EDGE('',*,*,#9700,.T.) ;
#14182=ORIENTED_EDGE('',*,*,#9240,.T.) ;
#14183=ORIENTED_EDGE('',*,*,#9597,.F.) ;
#14184=ORIENTED_EDGE('',*,*,#9483,.T.) ;
#14185=ORIENTED_EDGE('',*,*,#9701,.T.) ;
#14186=ORIENTED_EDGE('',*,*,#9356,.F.) ;
#14187=ORIENTED_EDGE('',*,*,#9163,.T.) ;
#14188=ORIENTED_EDGE('',*,*,#9702,.F.) ;
#14189=ORIENTED_EDGE('',*,*,#9241,.T.) ;
#14190=ORIENTED_EDGE('',*,*,#9700,.F.) ;
#14191=ORIENTED_EDGE('',*,*,#9165,.T.) ;
#14192=ORIENTED_EDGE('',*,*,#9357,.T.) ;
#14193=ORIENTED_EDGE('',*,*,#9701,.F.) ;
#14194=ORIENTED_EDGE('',*,*,#9482,.T.) ;
#14195=ORIENTED_EDGE('',*,*,#9703,.F.) ;
#14196=ORIENTED_EDGE('',*,*,#9358,.T.) ;
#14197=ORIENTED_EDGE('',*,*,#9162,.F.) ;
#14198=ORIENTED_EDGE('',*,*,#9359,.F.) ;
#14199=ORIENTED_EDGE('',*,*,#9703,.T.) ;
#14200=ORIENTED_EDGE('',*,*,#9484,.T.) ;
#14201=ORIENTED_EDGE('',*,*,#9598,.F.) ;
#14202=ORIENTED_EDGE('',*,*,#9242,.T.) ;
#14203=ORIENTED_EDGE('',*,*,#9702,.T.) ;
#14204=ORIENTED_EDGE('',*,*,#9160,.F.) ;
#14205=ORIENTED_EDGE('',*,*,#9704,.T.) ;
#14206=ORIENTED_EDGE('',*,*,#9322,.T.) ;
#14207=ORIENTED_EDGE('',*,*,#9599,.F.) ;
#14208=ORIENTED_EDGE('',*,*,#9459,.T.) ;
#14209=ORIENTED_EDGE('',*,*,#9705,.T.) ;
#14210=ORIENTED_EDGE('',*,*,#9360,.F.) ;
#14211=ORIENTED_EDGE('',*,*,#9157,.T.) ;
#14212=ORIENTED_EDGE('',*,*,#9706,.F.) ;
#14213=ORIENTED_EDGE('',*,*,#9323,.T.) ;
#14214=ORIENTED_EDGE('',*,*,#9704,.F.) ;
#14215=ORIENTED_EDGE('',*,*,#9159,.T.) ;
#14216=ORIENTED_EDGE('',*,*,#9361,.T.) ;
#14217=ORIENTED_EDGE('',*,*,#9705,.F.) ;
#14218=ORIENTED_EDGE('',*,*,#9458,.T.) ;
#14219=ORIENTED_EDGE('',*,*,#9707,.F.) ;
#14220=ORIENTED_EDGE('',*,*,#9362,.T.) ;
#14221=ORIENTED_EDGE('',*,*,#9156,.F.) ;
#14222=ORIENTED_EDGE('',*,*,#9363,.F.) ;
#14223=ORIENTED_EDGE('',*,*,#9707,.T.) ;
#14224=ORIENTED_EDGE('',*,*,#9460,.T.) ;
#14225=ORIENTED_EDGE('',*,*,#9600,.F.) ;
#14226=ORIENTED_EDGE('',*,*,#9324,.T.) ;
#14227=ORIENTED_EDGE('',*,*,#9706,.T.) ;
#14228=ORIENTED_EDGE('',*,*,#9154,.F.) ;
#14229=ORIENTED_EDGE('',*,*,#9708,.T.) ;
#14230=ORIENTED_EDGE('',*,*,#9245,.T.) ;
#14231=ORIENTED_EDGE('',*,*,#9601,.F.) ;
#14232=ORIENTED_EDGE('',*,*,#9486,.T.) ;
#14233=ORIENTED_EDGE('',*,*,#9709,.T.) ;
#14234=ORIENTED_EDGE('',*,*,#9364,.F.) ;
#14235=ORIENTED_EDGE('',*,*,#9151,.T.) ;
#14236=ORIENTED_EDGE('',*,*,#9710,.F.) ;
#14237=ORIENTED_EDGE('',*,*,#9246,.T.) ;
#14238=ORIENTED_EDGE('',*,*,#9708,.F.) ;
#14239=ORIENTED_EDGE('',*,*,#9153,.T.) ;
#14240=ORIENTED_EDGE('',*,*,#9365,.T.) ;
#14241=ORIENTED_EDGE('',*,*,#9709,.F.) ;
#14242=ORIENTED_EDGE('',*,*,#9485,.T.) ;
#14243=ORIENTED_EDGE('',*,*,#9711,.F.) ;
#14244=ORIENTED_EDGE('',*,*,#9366,.T.) ;
#14245=ORIENTED_EDGE('',*,*,#9150,.F.) ;
#14246=ORIENTED_EDGE('',*,*,#9367,.F.) ;
#14247=ORIENTED_EDGE('',*,*,#9711,.T.) ;
#14248=ORIENTED_EDGE('',*,*,#9487,.T.) ;
#14249=ORIENTED_EDGE('',*,*,#9602,.F.) ;
#14250=ORIENTED_EDGE('',*,*,#9247,.T.) ;
#14251=ORIENTED_EDGE('',*,*,#9710,.T.) ;
#14252=ORIENTED_EDGE('',*,*,#9148,.F.) ;
#14253=ORIENTED_EDGE('',*,*,#9712,.T.) ;
#14254=ORIENTED_EDGE('',*,*,#9249,.T.) ;
#14255=ORIENTED_EDGE('',*,*,#9603,.F.) ;
#14256=ORIENTED_EDGE('',*,*,#9456,.T.) ;
#14257=ORIENTED_EDGE('',*,*,#9713,.T.) ;
#14258=ORIENTED_EDGE('',*,*,#9368,.F.) ;
#14259=ORIENTED_EDGE('',*,*,#9145,.T.) ;
#14260=ORIENTED_EDGE('',*,*,#9714,.F.) ;
#14261=ORIENTED_EDGE('',*,*,#9250,.T.) ;
#14262=ORIENTED_EDGE('',*,*,#9712,.F.) ;
#14263=ORIENTED_EDGE('',*,*,#9147,.T.) ;
#14264=ORIENTED_EDGE('',*,*,#9369,.T.) ;
#14265=ORIENTED_EDGE('',*,*,#9713,.F.) ;
#14266=ORIENTED_EDGE('',*,*,#9455,.T.) ;
#14267=ORIENTED_EDGE('',*,*,#9715,.F.) ;
#14268=ORIENTED_EDGE('',*,*,#9370,.T.) ;
#14269=ORIENTED_EDGE('',*,*,#9144,.F.) ;
#14270=ORIENTED_EDGE('',*,*,#9371,.F.) ;
#14271=ORIENTED_EDGE('',*,*,#9715,.T.) ;
#14272=ORIENTED_EDGE('',*,*,#9457,.T.) ;
#14273=ORIENTED_EDGE('',*,*,#9604,.F.) ;
#14274=ORIENTED_EDGE('',*,*,#9251,.T.) ;
#14275=ORIENTED_EDGE('',*,*,#9714,.T.) ;
#14276=ORIENTED_EDGE('',*,*,#9142,.F.) ;
#14277=ORIENTED_EDGE('',*,*,#9716,.T.) ;
#14278=ORIENTED_EDGE('',*,*,#9253,.T.) ;
#14279=ORIENTED_EDGE('',*,*,#9605,.F.) ;
#14280=ORIENTED_EDGE('',*,*,#9489,.T.) ;
#14281=ORIENTED_EDGE('',*,*,#9717,.T.) ;
#14282=ORIENTED_EDGE('',*,*,#9372,.F.) ;
#14283=ORIENTED_EDGE('',*,*,#9139,.T.) ;
#14284=ORIENTED_EDGE('',*,*,#9718,.F.) ;
#14285=ORIENTED_EDGE('',*,*,#9254,.T.) ;
#14286=ORIENTED_EDGE('',*,*,#9716,.F.) ;
#14287=ORIENTED_EDGE('',*,*,#9141,.T.) ;
#14288=ORIENTED_EDGE('',*,*,#9373,.T.) ;
#14289=ORIENTED_EDGE('',*,*,#9717,.F.) ;
#14290=ORIENTED_EDGE('',*,*,#9488,.T.) ;
#14291=ORIENTED_EDGE('',*,*,#9719,.F.) ;
#14292=ORIENTED_EDGE('',*,*,#9374,.T.) ;
#14293=ORIENTED_EDGE('',*,*,#9138,.F.) ;
#14294=ORIENTED_EDGE('',*,*,#9375,.F.) ;
#14295=ORIENTED_EDGE('',*,*,#9719,.T.) ;
#14296=ORIENTED_EDGE('',*,*,#9490,.T.) ;
#14297=ORIENTED_EDGE('',*,*,#9606,.F.) ;
#14298=ORIENTED_EDGE('',*,*,#9255,.T.) ;
#14299=ORIENTED_EDGE('',*,*,#9718,.T.) ;
#14300=ORIENTED_EDGE('',*,*,#9136,.F.) ;
#14301=ORIENTED_EDGE('',*,*,#9720,.T.) ;
#14302=ORIENTED_EDGE('',*,*,#9257,.T.) ;
#14303=ORIENTED_EDGE('',*,*,#9607,.F.) ;
#14304=ORIENTED_EDGE('',*,*,#9453,.T.) ;
#14305=ORIENTED_EDGE('',*,*,#9721,.T.) ;
#14306=ORIENTED_EDGE('',*,*,#9376,.F.) ;
#14307=ORIENTED_EDGE('',*,*,#9133,.T.) ;
#14308=ORIENTED_EDGE('',*,*,#9722,.F.) ;
#14309=ORIENTED_EDGE('',*,*,#9258,.T.) ;
#14310=ORIENTED_EDGE('',*,*,#9720,.F.) ;
#14311=ORIENTED_EDGE('',*,*,#9135,.T.) ;
#14312=ORIENTED_EDGE('',*,*,#9377,.T.) ;
#14313=ORIENTED_EDGE('',*,*,#9721,.F.) ;
#14314=ORIENTED_EDGE('',*,*,#9452,.T.) ;
#14315=ORIENTED_EDGE('',*,*,#9723,.F.) ;
#14316=ORIENTED_EDGE('',*,*,#9378,.T.) ;
#14317=ORIENTED_EDGE('',*,*,#9132,.F.) ;
#14318=ORIENTED_EDGE('',*,*,#9379,.F.) ;
#14319=ORIENTED_EDGE('',*,*,#9723,.T.) ;
#14320=ORIENTED_EDGE('',*,*,#9454,.T.) ;
#14321=ORIENTED_EDGE('',*,*,#9608,.F.) ;
#14322=ORIENTED_EDGE('',*,*,#9259,.T.) ;
#14323=ORIENTED_EDGE('',*,*,#9722,.T.) ;
#14324=ORIENTED_EDGE('',*,*,#9130,.F.) ;
#14325=ORIENTED_EDGE('',*,*,#9724,.T.) ;
#14326=ORIENTED_EDGE('',*,*,#9325,.T.) ;
#14327=ORIENTED_EDGE('',*,*,#9609,.F.) ;
#14328=ORIENTED_EDGE('',*,*,#9492,.T.) ;
#14329=ORIENTED_EDGE('',*,*,#9725,.T.) ;
#14330=ORIENTED_EDGE('',*,*,#9380,.F.) ;
#14331=ORIENTED_EDGE('',*,*,#9127,.T.) ;
#14332=ORIENTED_EDGE('',*,*,#9726,.F.) ;
#14333=ORIENTED_EDGE('',*,*,#9326,.T.) ;
#14334=ORIENTED_EDGE('',*,*,#9724,.F.) ;
#14335=ORIENTED_EDGE('',*,*,#9129,.T.) ;
#14336=ORIENTED_EDGE('',*,*,#9381,.T.) ;
#14337=ORIENTED_EDGE('',*,*,#9725,.F.) ;
#14338=ORIENTED_EDGE('',*,*,#9491,.T.) ;
#14339=ORIENTED_EDGE('',*,*,#9727,.F.) ;
#14340=ORIENTED_EDGE('',*,*,#9382,.T.) ;
#14341=ORIENTED_EDGE('',*,*,#9126,.F.) ;
#14342=ORIENTED_EDGE('',*,*,#9383,.F.) ;
#14343=ORIENTED_EDGE('',*,*,#9727,.T.) ;
#14344=ORIENTED_EDGE('',*,*,#9493,.T.) ;
#14345=ORIENTED_EDGE('',*,*,#9610,.F.) ;
#14346=ORIENTED_EDGE('',*,*,#9327,.T.) ;
#14347=ORIENTED_EDGE('',*,*,#9726,.T.) ;
#14567=CONICAL_SURFACE('',#17273,28.523658167371,1.38589614583862) ;
#14568=CONICAL_SURFACE('',#17334,26.6311750163962,0.166009849666151) ;
#14569=CONICAL_SURFACE('',#17454,32.4669335366504,0.203790512246407) ;
#14570=CONICAL_SURFACE('',#17598,26.3029085923563,1.38589614583862) ;
#14571=CONICAL_SURFACE('',#17599,3.04415568548155,0.0188926771603406) ;
#14572=CONICAL_SURFACE('',#17605,3.04415568548155,0.0188926771603406) ;
#14573=CONICAL_SURFACE('',#17606,3.04415568548155,0.0188926771603406) ;
#14574=CONICAL_SURFACE('',#17612,3.04415568548155,0.0188926771603406) ;
#14575=CONICAL_SURFACE('',#17613,3.04415568548155,0.0188926771603406) ;
#14576=CONICAL_SURFACE('',#17619,3.04415568548155,0.0188926771603406) ;
#14577=CONICAL_SURFACE('',#17620,3.04415568548155,0.0188926771603406) ;
#14578=CONICAL_SURFACE('',#17626,3.04415568548155,0.0188926771603406) ;
#14579=CONICAL_SURFACE('',#17627,3.04415568548155,0.0188926771603406) ;
#14580=CONICAL_SURFACE('',#17633,3.04415568548155,0.0188926771603406) ;
#14581=CONICAL_SURFACE('',#17634,3.04415568548155,0.0188926771603406) ;
#14582=CONICAL_SURFACE('',#17640,3.04415568548155,0.0188926771603406) ;
#14583=CONICAL_SURFACE('',#17641,3.04415568548155,0.0188926771603406) ;
#14584=CONICAL_SURFACE('',#17647,3.04415568548155,0.0188926771603406) ;
#14585=CONICAL_SURFACE('',#17648,3.04415568548155,0.0188926771603406) ;
#14586=CONICAL_SURFACE('',#17654,3.04415568548155,0.0188926771603406) ;
#14587=CONICAL_SURFACE('',#17655,3.04415568548155,0.0188926771603406) ;
#14588=CONICAL_SURFACE('',#17661,3.04415568548155,0.0188926771603406) ;
#14589=CONICAL_SURFACE('',#17662,3.04415568548155,0.0188926771603406) ;
#14590=CONICAL_SURFACE('',#17668,3.04415568548155,0.0188926771603406) ;
#14591=CONICAL_SURFACE('',#17669,3.04415568548155,0.0188926771603406) ;
#14592=CONICAL_SURFACE('',#17675,3.04415568548155,0.0188926771603406) ;
#14593=CONICAL_SURFACE('',#17676,3.04415568548155,0.0188926771603406) ;
#14594=CONICAL_SURFACE('',#17682,3.04415568548155,0.0188926771603406) ;
#14595=CONICAL_SURFACE('',#17683,3.04415568548155,0.0188926771603406) ;
#14596=CONICAL_SURFACE('',#17689,3.04415568548155,0.0188926771603406) ;
#14597=CONICAL_SURFACE('',#17690,3.04415568548155,0.0188926771603406) ;
#14598=CONICAL_SURFACE('',#17696,3.04415568548155,0.0188926771603406) ;
#14599=CONICAL_SURFACE('',#17697,3.04415568548155,0.0188926771603406) ;
#14600=CONICAL_SURFACE('',#17703,3.04415568548155,0.0188926771603406) ;
#14601=CONICAL_SURFACE('',#17704,3.04415568548155,0.0188926771603406) ;
#14602=CONICAL_SURFACE('',#17710,3.04415568548155,0.0188926771603406) ;
#14603=CONICAL_SURFACE('',#17711,3.04415568548155,0.0188926771603406) ;
#14604=CONICAL_SURFACE('',#17717,3.04415568548155,0.0188926771603406) ;
#14605=CONICAL_SURFACE('',#17718,3.04415568548155,0.0188926771603406) ;
#14606=CONICAL_SURFACE('',#17724,3.04415568548155,0.0188926771603406) ;
#14607=CONICAL_SURFACE('',#17725,3.04415568548155,0.0188926771603406) ;
#14608=CONICAL_SURFACE('',#17731,3.04415568548155,0.0188926771603406) ;
#14609=CONICAL_SURFACE('',#17732,3.04415568548155,0.0188926771603406) ;
#14610=CONICAL_SURFACE('',#17738,3.04415568548155,0.0188926771603406) ;
#14611=CONICAL_SURFACE('',#17739,3.04415568548155,0.0188926771603406) ;
#14612=CONICAL_SURFACE('',#17745,3.04415568548155,0.0188926771603406) ;
#14613=CONICAL_SURFACE('',#17746,3.04415568548155,0.0188926771603406) ;
#14614=CONICAL_SURFACE('',#17752,3.04415568548155,0.0188926771603406) ;
#14615=CONICAL_SURFACE('',#17753,3.04415568548155,0.0188926771603406) ;
#14616=CONICAL_SURFACE('',#17759,3.04415568548155,0.0188926771603406) ;
#14617=CONICAL_SURFACE('',#17760,3.04415568548155,0.0188926771603406) ;
#14618=CONICAL_SURFACE('',#17766,3.04415568548155,0.0188926771603406) ;
#14619=CONICAL_SURFACE('',#17767,3.04415568548155,0.0188926771603406) ;
#14620=CONICAL_SURFACE('',#17773,3.04415568548155,0.0188926771603406) ;
#14621=CONICAL_SURFACE('',#17774,3.04415568548155,0.0188926771603406) ;
#14622=CONICAL_SURFACE('',#17780,3.04415568548155,0.0188926771603406) ;
#14623=CONICAL_SURFACE('',#17781,3.04415568548155,0.0188926771603406) ;
#14624=CONICAL_SURFACE('',#17787,3.04415568548155,0.0188926771603406) ;
#14625=CONICAL_SURFACE('',#17788,3.04415568548155,0.0188926771603406) ;
#14626=CONICAL_SURFACE('',#17794,3.04415568548155,0.0188926771603406) ;
#14627=CONICAL_SURFACE('',#17795,3.04415568548155,0.0188926771603406) ;
#14628=CONICAL_SURFACE('',#17801,3.04415568548155,0.0188926771603406) ;
#15330=ADVANCED_FACE('',(#2242),#14567,.F.) ;
#15331=ADVANCED_FACE('',(#2243,#759,#760),#14568,.T.) ;
#15332=ADVANCED_FACE('',(#2244),#1519,.T.) ;
#15333=ADVANCED_FACE('',(#2245,#761,#762,#763,#764,#765,#766,#767,#768,
#769,#770,#771,#772,#773,#774,#775,#776,#777,#778,#779,#780,#781,#782,#783,
#784,#785,#786,#787,#788,#789),#14569,.F.) ;
#15334=ADVANCED_FACE('',(#2246),#1520,.T.) ;
#15335=ADVANCED_FACE('',(#2247),#79,.T.) ;
#15336=ADVANCED_FACE('',(#2248),#80,.T.) ;
#15337=ADVANCED_FACE('',(#2249),#81,.T.) ;
#15338=ADVANCED_FACE('',(#2250),#1521,.F.) ;
#15339=ADVANCED_FACE('',(#2251),#82,.T.) ;
#15340=ADVANCED_FACE('',(#2252),#1522,.T.) ;
#15341=ADVANCED_FACE('',(#2253,#790),#1048,.T.) ;
#15342=ADVANCED_FACE('',(#2254,#791),#1049,.T.) ;
#15343=ADVANCED_FACE('',(#2255,#792),#1050,.T.) ;
#15344=ADVANCED_FACE('',(#2256),#1051,.T.) ;
#15345=ADVANCED_FACE('',(#2257),#1052,.T.) ;
#15346=ADVANCED_FACE('',(#2258),#1053,.T.) ;
#15347=ADVANCED_FACE('',(#2259),#1054,.T.) ;
#15348=ADVANCED_FACE('',(#2260),#1055,.T.) ;
#15349=ADVANCED_FACE('',(#2261),#1056,.T.) ;
#15350=ADVANCED_FACE('',(#2262),#1057,.T.) ;
#15351=ADVANCED_FACE('',(#2263),#1058,.T.) ;
#15352=ADVANCED_FACE('',(#2264),#1059,.T.) ;
#15353=ADVANCED_FACE('',(#2265),#1060,.T.) ;
#15354=ADVANCED_FACE('',(#2266),#1061,.T.) ;
#15355=ADVANCED_FACE('',(#2267),#1062,.T.) ;
#15356=ADVANCED_FACE('',(#2268),#1063,.T.) ;
#15357=ADVANCED_FACE('',(#2269),#1064,.T.) ;
#15358=ADVANCED_FACE('',(#2270),#1065,.T.) ;
#15359=ADVANCED_FACE('',(#2271),#1066,.T.) ;
#15360=ADVANCED_FACE('',(#2272),#1067,.T.) ;
#15361=ADVANCED_FACE('',(#2273),#1068,.T.) ;
#15362=ADVANCED_FACE('',(#2274),#1069,.T.) ;
#15363=ADVANCED_FACE('',(#2275),#1070,.T.) ;
#15364=ADVANCED_FACE('',(#2276),#1071,.T.) ;
#15365=ADVANCED_FACE('',(#2277),#1072,.T.) ;
#15366=ADVANCED_FACE('',(#2278),#1073,.T.) ;
#15367=ADVANCED_FACE('',(#2279),#1074,.T.) ;
#15368=ADVANCED_FACE('',(#2280),#1075,.T.) ;
#15369=ADVANCED_FACE('',(#2281),#1076,.T.) ;
#15370=ADVANCED_FACE('',(#2282),#1077,.T.) ;
#15371=ADVANCED_FACE('',(#2283),#1078,.T.) ;
#15372=ADVANCED_FACE('',(#2284,#793),#1079,.T.) ;
#15373=ADVANCED_FACE('',(#2285),#1080,.T.) ;
#15374=ADVANCED_FACE('',(#2286),#14570,.T.) ;
#15375=ADVANCED_FACE('',(#2287),#14571,.T.) ;
#15376=ADVANCED_FACE('',(#2288),#1081,.T.) ;
#15377=ADVANCED_FACE('',(#2289),#14572,.T.) ;
#15378=ADVANCED_FACE('',(#2290),#14573,.T.) ;
#15379=ADVANCED_FACE('',(#2291),#1082,.T.) ;
#15380=ADVANCED_FACE('',(#2292),#14574,.T.) ;
#15381=ADVANCED_FACE('',(#2293),#14575,.T.) ;
#15382=ADVANCED_FACE('',(#2294),#1083,.T.) ;
#15383=ADVANCED_FACE('',(#2295),#14576,.T.) ;
#15384=ADVANCED_FACE('',(#2296),#14577,.T.) ;
#15385=ADVANCED_FACE('',(#2297),#1084,.T.) ;
#15386=ADVANCED_FACE('',(#2298),#14578,.T.) ;
#15387=ADVANCED_FACE('',(#2299),#14579,.T.) ;
#15388=ADVANCED_FACE('',(#2300),#1085,.T.) ;
#15389=ADVANCED_FACE('',(#2301),#14580,.T.) ;
#15390=ADVANCED_FACE('',(#2302),#14581,.T.) ;
#15391=ADVANCED_FACE('',(#2303),#1086,.T.) ;
#15392=ADVANCED_FACE('',(#2304),#14582,.T.) ;
#15393=ADVANCED_FACE('',(#2305),#14583,.T.) ;
#15394=ADVANCED_FACE('',(#2306),#1087,.T.) ;
#15395=ADVANCED_FACE('',(#2307),#14584,.T.) ;
#15396=ADVANCED_FACE('',(#2308),#14585,.T.) ;
#15397=ADVANCED_FACE('',(#2309),#1088,.T.) ;
#15398=ADVANCED_FACE('',(#2310),#14586,.T.) ;
#15399=ADVANCED_FACE('',(#2311),#14587,.T.) ;
#15400=ADVANCED_FACE('',(#2312),#1089,.T.) ;
#15401=ADVANCED_FACE('',(#2313),#14588,.T.) ;
#15402=ADVANCED_FACE('',(#2314),#14589,.T.) ;
#15403=ADVANCED_FACE('',(#2315),#1090,.T.) ;
#15404=ADVANCED_FACE('',(#2316),#14590,.T.) ;
#15405=ADVANCED_FACE('',(#2317),#14591,.T.) ;
#15406=ADVANCED_FACE('',(#2318),#1091,.T.) ;
#15407=ADVANCED_FACE('',(#2319),#14592,.T.) ;
#15408=ADVANCED_FACE('',(#2320),#14593,.T.) ;
#15409=ADVANCED_FACE('',(#2321),#1092,.T.) ;
#15410=ADVANCED_FACE('',(#2322),#14594,.T.) ;
#15411=ADVANCED_FACE('',(#2323),#14595,.T.) ;
#15412=ADVANCED_FACE('',(#2324),#1093,.T.) ;
#15413=ADVANCED_FACE('',(#2325),#14596,.T.) ;
#15414=ADVANCED_FACE('',(#2326),#14597,.T.) ;
#15415=ADVANCED_FACE('',(#2327),#1094,.T.) ;
#15416=ADVANCED_FACE('',(#2328),#14598,.T.) ;
#15417=ADVANCED_FACE('',(#2329),#14599,.T.) ;
#15418=ADVANCED_FACE('',(#2330),#1095,.T.) ;
#15419=ADVANCED_FACE('',(#2331),#14600,.T.) ;
#15420=ADVANCED_FACE('',(#2332),#14601,.T.) ;
#15421=ADVANCED_FACE('',(#2333),#1096,.T.) ;
#15422=ADVANCED_FACE('',(#2334),#14602,.T.) ;
#15423=ADVANCED_FACE('',(#2335),#14603,.T.) ;
#15424=ADVANCED_FACE('',(#2336),#1097,.T.) ;
#15425=ADVANCED_FACE('',(#2337),#14604,.T.) ;
#15426=ADVANCED_FACE('',(#2338),#14605,.T.) ;
#15427=ADVANCED_FACE('',(#2339),#1098,.T.) ;
#15428=ADVANCED_FACE('',(#2340),#14606,.T.) ;
#15429=ADVANCED_FACE('',(#2341),#14607,.T.) ;
#15430=ADVANCED_FACE('',(#2342),#1099,.T.) ;
#15431=ADVANCED_FACE('',(#2343),#14608,.T.) ;
#15432=ADVANCED_FACE('',(#2344),#14609,.T.) ;
#15433=ADVANCED_FACE('',(#2345),#1100,.T.) ;
#15434=ADVANCED_FACE('',(#2346),#14610,.T.) ;
#15435=ADVANCED_FACE('',(#2347),#14611,.T.) ;
#15436=ADVANCED_FACE('',(#2348),#1101,.T.) ;
#15437=ADVANCED_FACE('',(#2349),#14612,.T.) ;
#15438=ADVANCED_FACE('',(#2350),#14613,.T.) ;
#15439=ADVANCED_FACE('',(#2351),#1102,.T.) ;
#15440=ADVANCED_FACE('',(#2352),#14614,.T.) ;
#15441=ADVANCED_FACE('',(#2353),#14615,.T.) ;
#15442=ADVANCED_FACE('',(#2354),#1103,.T.) ;
#15443=ADVANCED_FACE('',(#2355),#14616,.T.) ;
#15444=ADVANCED_FACE('',(#2356),#14617,.T.) ;
#15445=ADVANCED_FACE('',(#2357),#1104,.T.) ;
#15446=ADVANCED_FACE('',(#2358),#14618,.T.) ;
#15447=ADVANCED_FACE('',(#2359),#14619,.T.) ;
#15448=ADVANCED_FACE('',(#2360),#1105,.T.) ;
#15449=ADVANCED_FACE('',(#2361),#14620,.T.) ;
#15450=ADVANCED_FACE('',(#2362),#14621,.T.) ;
#15451=ADVANCED_FACE('',(#2363),#1106,.T.) ;
#15452=ADVANCED_FACE('',(#2364),#14622,.T.) ;
#15453=ADVANCED_FACE('',(#2365),#14623,.T.) ;
#15454=ADVANCED_FACE('',(#2366),#1107,.T.) ;
#15455=ADVANCED_FACE('',(#2367),#14624,.T.) ;
#15456=ADVANCED_FACE('',(#2368),#14625,.T.) ;
#15457=ADVANCED_FACE('',(#2369),#1108,.T.) ;
#15458=ADVANCED_FACE('',(#2370),#14626,.T.) ;
#15459=ADVANCED_FACE('',(#2371),#14627,.T.) ;
#15460=ADVANCED_FACE('',(#2372),#1109,.T.) ;
#15461=ADVANCED_FACE('',(#2373),#14628,.T.) ;
#15505=CLOSED_SHELL('',(#15330,#15331,#15332,#15333,#15334,#15335,#15336,
#15337,#15338,#15339,#15340,#15341,#15342,#15343,#15344,#15345,#15346,#15347,
#15348,#15349,#15350,#15351,#15352,#15353,#15354,#15355,#15356,#15357,#15358,
#15359,#15360,#15361,#15362,#15363,#15364,#15365,#15366,#15367,#15368,#15369,
#15370,#15371,#15372,#15373,#15374,#15375,#15376,#15377,#15378,#15379,#15380,
#15381,#15382,#15383,#15384,#15385,#15386,#15387,#15388,#15389,#15390,#15391,
#15392,#15393,#15394,#15395,#15396,#15397,#15398,#15399,#15400,#15401,#15402,
#15403,#15404,#15405,#15406,#15407,#15408,#15409,#15410,#15411,#15412,#15413,
#15414,#15415,#15416,#15417,#15418,#15419,#15420,#15421,#15422,#15423,#15424,
#15425,#15426,#15427,#15428,#15429,#15430,#15431,#15432,#15433,#15434,#15435,
#15436,#15437,#15438,#15439,#15440,#15441,#15442,#15443,#15444,#15445,#15446,
#15447,#15448,#15449,#15450,#15451,#15452,#15453,#15454,#15455,#15456,#15457,
#15458,#15459,#15460,#15461)) ;
#17272=AXIS2_PLACEMENT_3D('',#53877,#21660,#21661) ;
#17273=AXIS2_PLACEMENT_3D('',#53878,#21662,#21663) ;
#17274=AXIS2_PLACEMENT_3D('',#53880,#21664,#21665) ;
#17275=AXIS2_PLACEMENT_3D('',#53884,#21667,#21668) ;
#17276=AXIS2_PLACEMENT_3D('',#53931,#21669,#21670) ;
#17277=AXIS2_PLACEMENT_3D('',#53978,#21671,#21672) ;
#17278=AXIS2_PLACEMENT_3D('',#54025,#21673,#21674) ;
#17279=AXIS2_PLACEMENT_3D('',#54072,#21675,#21676) ;
#17280=AXIS2_PLACEMENT_3D('',#54119,#21677,#21678) ;
#17281=AXIS2_PLACEMENT_3D('',#54166,#21679,#21680) ;
#17282=AXIS2_PLACEMENT_3D('',#54213,#21681,#21682) ;
#17283=AXIS2_PLACEMENT_3D('',#54260,#21683,#21684) ;
#17284=AXIS2_PLACEMENT_3D('',#54307,#21685,#21686) ;
#17285=AXIS2_PLACEMENT_3D('',#54354,#21687,#21688) ;
#17286=AXIS2_PLACEMENT_3D('',#54401,#21689,#21690) ;
#17287=AXIS2_PLACEMENT_3D('',#54448,#21691,#21692) ;
#17288=AXIS2_PLACEMENT_3D('',#54495,#21693,#21694) ;
#17289=AXIS2_PLACEMENT_3D('',#54542,#21695,#21696) ;
#17290=AXIS2_PLACEMENT_3D('',#54589,#21697,#21698) ;
#17291=AXIS2_PLACEMENT_3D('',#54636,#21699,#21700) ;
#17292=AXIS2_PLACEMENT_3D('',#54683,#21701,#21702) ;
#17293=AXIS2_PLACEMENT_3D('',#54730,#21703,#21704) ;
#17294=AXIS2_PLACEMENT_3D('',#54777,#21705,#21706) ;
#17295=AXIS2_PLACEMENT_3D('',#54824,#21707,#21708) ;
#17296=AXIS2_PLACEMENT_3D('',#54871,#21709,#21710) ;
#17297=AXIS2_PLACEMENT_3D('',#54918,#21711,#21712) ;
#17298=AXIS2_PLACEMENT_3D('',#54965,#21713,#21714) ;
#17299=AXIS2_PLACEMENT_3D('',#55012,#21715,#21716) ;
#17300=AXIS2_PLACEMENT_3D('',#55059,#21717,#21718) ;
#17301=AXIS2_PLACEMENT_3D('',#55106,#21719,#21720) ;
#17302=AXIS2_PLACEMENT_3D('',#55153,#21721,#21722) ;
#17303=AXIS2_PLACEMENT_3D('',#55200,#21723,#21724) ;
#17304=AXIS2_PLACEMENT_3D('',#55247,#21725,#21726) ;
#17305=AXIS2_PLACEMENT_3D('',#55294,#21727,#21728) ;
#17306=AXIS2_PLACEMENT_3D('',#55341,#21729,#21730) ;
#17307=AXIS2_PLACEMENT_3D('',#55388,#21731,#21732) ;
#17308=AXIS2_PLACEMENT_3D('',#55435,#21733,#21734) ;
#17309=AXIS2_PLACEMENT_3D('',#55482,#21735,#21736) ;
#17310=AXIS2_PLACEMENT_3D('',#55529,#21737,#21738) ;
#17311=AXIS2_PLACEMENT_3D('',#55576,#21739,#21740) ;
#17312=AXIS2_PLACEMENT_3D('',#55623,#21741,#21742) ;
#17313=AXIS2_PLACEMENT_3D('',#55670,#21743,#21744) ;
#17314=AXIS2_PLACEMENT_3D('',#55717,#21745,#21746) ;
#17315=AXIS2_PLACEMENT_3D('',#55764,#21747,#21748) ;
#17316=AXIS2_PLACEMENT_3D('',#55811,#21749,#21750) ;
#17317=AXIS2_PLACEMENT_3D('',#55858,#21751,#21752) ;
#17318=AXIS2_PLACEMENT_3D('',#55905,#21753,#21754) ;
#17319=AXIS2_PLACEMENT_3D('',#55952,#21755,#21756) ;
#17320=AXIS2_PLACEMENT_3D('',#55999,#21757,#21758) ;
#17321=AXIS2_PLACEMENT_3D('',#56046,#21759,#21760) ;
#17322=AXIS2_PLACEMENT_3D('',#56093,#21761,#21762) ;
#17323=AXIS2_PLACEMENT_3D('',#56140,#21763,#21764) ;
#17324=AXIS2_PLACEMENT_3D('',#56187,#21765,#21766) ;
#17325=AXIS2_PLACEMENT_3D('',#56234,#21767,#21768) ;
#17326=AXIS2_PLACEMENT_3D('',#56281,#21769,#21770) ;
#17327=AXIS2_PLACEMENT_3D('',#56328,#21771,#21772) ;
#17328=AXIS2_PLACEMENT_3D('',#56375,#21773,#21774) ;
#17329=AXIS2_PLACEMENT_3D('',#56422,#21775,#21776) ;
#17330=AXIS2_PLACEMENT_3D('',#56469,#21777,#21778) ;
#17331=AXIS2_PLACEMENT_3D('',#56516,#21779,#21780) ;
#17332=AXIS2_PLACEMENT_3D('',#56563,#21781,#21782) ;
#17333=AXIS2_PLACEMENT_3D('',#56609,#21783,#21784) ;
#17334=AXIS2_PLACEMENT_3D('',#56610,#21785,#21786) ;
#17335=AXIS2_PLACEMENT_3D('',#56614,#21788,#21789) ;
#17336=AXIS2_PLACEMENT_3D('',#56639,#21790,#21791) ;
#17337=AXIS2_PLACEMENT_3D('',#56651,#21792,#21793) ;
#17338=AXIS2_PLACEMENT_3D('',#56676,#21794,#21795) ;
#17339=AXIS2_PLACEMENT_3D('',#56690,#21796,#21797) ;
#17340=AXIS2_PLACEMENT_3D('',#56715,#21798,#21799) ;
#17341=AXIS2_PLACEMENT_3D('',#56727,#21800,#21801) ;
#17342=AXIS2_PLACEMENT_3D('',#56752,#21802,#21803) ;
#17343=AXIS2_PLACEMENT_3D('',#56766,#21804,#21805) ;
#17344=AXIS2_PLACEMENT_3D('',#56791,#21806,#21807) ;
#17345=AXIS2_PLACEMENT_3D('',#56803,#21808,#21809) ;
#17346=AXIS2_PLACEMENT_3D('',#56828,#21810,#21811) ;
#17347=AXIS2_PLACEMENT_3D('',#56858,#21812,#21813) ;
#17348=AXIS2_PLACEMENT_3D('',#56883,#21814,#21815) ;
#17349=AXIS2_PLACEMENT_3D('',#56895,#21816,#21817) ;
#17350=AXIS2_PLACEMENT_3D('',#56920,#21818,#21819) ;
#17351=AXIS2_PLACEMENT_3D('',#56934,#21820,#21821) ;
#17352=AXIS2_PLACEMENT_3D('',#56936,#21822,#21823) ;
#17353=AXIS2_PLACEMENT_3D('',#56961,#21824,#21825) ;
#17354=AXIS2_PLACEMENT_3D('',#56973,#21826,#21827) ;
#17355=AXIS2_PLACEMENT_3D('',#56998,#21828,#21829) ;
#17356=AXIS2_PLACEMENT_3D('',#57016,#21830,#21831) ;
#17357=AXIS2_PLACEMENT_3D('',#57041,#21832,#21833) ;
#17358=AXIS2_PLACEMENT_3D('',#57055,#21834,#21835) ;
#17359=AXIS2_PLACEMENT_3D('',#57080,#21836,#21837) ;
#17360=AXIS2_PLACEMENT_3D('',#57092,#21838,#21839) ;
#17361=AXIS2_PLACEMENT_3D('',#57094,#21840,#21841) ;
#17362=AXIS2_PLACEMENT_3D('',#57119,#21842,#21843) ;
#17363=AXIS2_PLACEMENT_3D('',#57133,#21844,#21845) ;
#17364=AXIS2_PLACEMENT_3D('',#57162,#21846,#21847) ;
#17365=AXIS2_PLACEMENT_3D('',#57184,#21848,#21849) ;
#17366=AXIS2_PLACEMENT_3D('',#57209,#21850,#21851) ;
#17367=AXIS2_PLACEMENT_3D('',#57221,#21852,#21853) ;
#17368=AXIS2_PLACEMENT_3D('',#57246,#21854,#21855) ;
#17369=AXIS2_PLACEMENT_3D('',#57260,#21856,#21857) ;
#17370=AXIS2_PLACEMENT_3D('',#57285,#21858,#21859) ;
#17371=AXIS2_PLACEMENT_3D('',#57299,#21860,#21861) ;
#17372=AXIS2_PLACEMENT_3D('',#57324,#21862,#21863) ;
#17373=AXIS2_PLACEMENT_3D('',#57344,#21864,#21865) ;
#17374=AXIS2_PLACEMENT_3D('',#57375,#21866,#21867) ;
#17375=AXIS2_PLACEMENT_3D('',#57395,#21868,#21869) ;
#17376=AXIS2_PLACEMENT_3D('',#57420,#21870,#21871) ;
#17377=AXIS2_PLACEMENT_3D('',#57434,#21872,#21873) ;
#17378=AXIS2_PLACEMENT_3D('',#57459,#21874,#21875) ;
#17379=AXIS2_PLACEMENT_3D('',#57471,#21876,#21877) ;
#17380=AXIS2_PLACEMENT_3D('',#57496,#21878,#21879) ;
#17381=AXIS2_PLACEMENT_3D('',#57510,#21880,#21881) ;
#17382=AXIS2_PLACEMENT_3D('',#57535,#21882,#21883) ;
#17383=AXIS2_PLACEMENT_3D('',#57547,#21884,#21885) ;
#17384=AXIS2_PLACEMENT_3D('',#57572,#21886,#21887) ;
#17385=AXIS2_PLACEMENT_3D('',#57586,#21888,#21889) ;
#17386=AXIS2_PLACEMENT_3D('',#57611,#21890,#21891) ;
#17387=AXIS2_PLACEMENT_3D('',#57623,#21892,#21893) ;
#17388=AXIS2_PLACEMENT_3D('',#57648,#21894,#21895) ;
#17389=AXIS2_PLACEMENT_3D('',#57662,#21896,#21897) ;
#17390=AXIS2_PLACEMENT_3D('',#57687,#21898,#21899) ;
#17391=AXIS2_PLACEMENT_3D('',#57700,#21900,#21901) ;
#17392=AXIS2_PLACEMENT_3D('',#57729,#21902,#21903) ;
#17393=AXIS2_PLACEMENT_3D('',#57780,#21904,#21905) ;
#17394=AXIS2_PLACEMENT_3D('',#57801,#21906,#21907) ;
#17395=AXIS2_PLACEMENT_3D('',#57804,#21909,#21910) ;
#17396=AXIS2_PLACEMENT_3D('',#57806,#21911,#21912) ;
#17397=AXIS2_PLACEMENT_3D('',#57810,#21915,#21916) ;
#17398=AXIS2_PLACEMENT_3D('',#57812,#21917,#21918) ;
#17399=AXIS2_PLACEMENT_3D('',#57816,#21921,#21922) ;
#17400=AXIS2_PLACEMENT_3D('',#57818,#21923,#21924) ;
#17401=AXIS2_PLACEMENT_3D('',#57822,#21927,#21928) ;
#17402=AXIS2_PLACEMENT_3D('',#57824,#21929,#21930) ;
#17403=AXIS2_PLACEMENT_3D('',#57828,#21933,#21934) ;
#17404=AXIS2_PLACEMENT_3D('',#57830,#21935,#21936) ;
#17405=AXIS2_PLACEMENT_3D('',#57834,#21939,#21940) ;
#17406=AXIS2_PLACEMENT_3D('',#57836,#21941,#21942) ;
#17407=AXIS2_PLACEMENT_3D('',#57840,#21945,#21946) ;
#17408=AXIS2_PLACEMENT_3D('',#57842,#21947,#21948) ;
#17409=AXIS2_PLACEMENT_3D('',#57846,#21951,#21952) ;
#17410=AXIS2_PLACEMENT_3D('',#57848,#21953,#21954) ;
#17411=AXIS2_PLACEMENT_3D('',#57852,#21957,#21958) ;
#17412=AXIS2_PLACEMENT_3D('',#57854,#21959,#21960) ;
#17413=AXIS2_PLACEMENT_3D('',#57858,#21963,#21964) ;
#17414=AXIS2_PLACEMENT_3D('',#57860,#21965,#21966) ;
#17415=AXIS2_PLACEMENT_3D('',#57864,#21969,#21970) ;
#17416=AXIS2_PLACEMENT_3D('',#57866,#21971,#21972) ;
#17417=AXIS2_PLACEMENT_3D('',#57870,#21975,#21976) ;
#17418=AXIS2_PLACEMENT_3D('',#57872,#21977,#21978) ;
#17419=AXIS2_PLACEMENT_3D('',#57876,#21981,#21982) ;
#17420=AXIS2_PLACEMENT_3D('',#57878,#21983,#21984) ;
#17421=AXIS2_PLACEMENT_3D('',#57882,#21987,#21988) ;
#17422=AXIS2_PLACEMENT_3D('',#57884,#21989,#21990) ;
#17423=AXIS2_PLACEMENT_3D('',#57888,#21993,#21994) ;
#17424=AXIS2_PLACEMENT_3D('',#57890,#21995,#21996) ;
#17425=AXIS2_PLACEMENT_3D('',#57894,#21999,#22000) ;
#17426=AXIS2_PLACEMENT_3D('',#57896,#22001,#22002) ;
#17427=AXIS2_PLACEMENT_3D('',#57900,#22005,#22006) ;
#17428=AXIS2_PLACEMENT_3D('',#57902,#22007,#22008) ;
#17429=AXIS2_PLACEMENT_3D('',#57906,#22011,#22012) ;
#17430=AXIS2_PLACEMENT_3D('',#57908,#22013,#22014) ;
#17431=AXIS2_PLACEMENT_3D('',#57912,#22017,#22018) ;
#17432=AXIS2_PLACEMENT_3D('',#57914,#22019,#22020) ;
#17433=AXIS2_PLACEMENT_3D('',#57918,#22023,#22024) ;
#17434=AXIS2_PLACEMENT_3D('',#57920,#22025,#22026) ;
#17435=AXIS2_PLACEMENT_3D('',#57924,#22029,#22030) ;
#17436=AXIS2_PLACEMENT_3D('',#57926,#22031,#22032) ;
#17437=AXIS2_PLACEMENT_3D('',#57930,#22035,#22036) ;
#17438=AXIS2_PLACEMENT_3D('',#57932,#22037,#22038) ;
#17439=AXIS2_PLACEMENT_3D('',#57936,#22041,#22042) ;
#17440=AXIS2_PLACEMENT_3D('',#57938,#22043,#22044) ;
#17441=AXIS2_PLACEMENT_3D('',#57942,#22047,#22048) ;
#17442=AXIS2_PLACEMENT_3D('',#57944,#22049,#22050) ;
#17443=AXIS2_PLACEMENT_3D('',#57948,#22053,#22054) ;
#17444=AXIS2_PLACEMENT_3D('',#57950,#22055,#22056) ;
#17445=AXIS2_PLACEMENT_3D('',#57954,#22059,#22060) ;
#17446=AXIS2_PLACEMENT_3D('',#57956,#22061,#22062) ;
#17447=AXIS2_PLACEMENT_3D('',#57960,#22065,#22066) ;
#17448=AXIS2_PLACEMENT_3D('',#57962,#22067,#22068) ;
#17449=AXIS2_PLACEMENT_3D('',#57966,#22071,#22072) ;
#17450=AXIS2_PLACEMENT_3D('',#57968,#22073,#22074) ;
#17451=AXIS2_PLACEMENT_3D('',#57972,#22077,#22078) ;
#17452=AXIS2_PLACEMENT_3D('',#57974,#22079,#22080) ;
#17453=AXIS2_PLACEMENT_3D('',#57978,#22083,#22084) ;
#17454=AXIS2_PLACEMENT_3D('',#57979,#22085,#22086) ;
#17455=AXIS2_PLACEMENT_3D('',#57981,#22087,#22088) ;
#17456=AXIS2_PLACEMENT_3D('',#57984,#22090,#22091) ;
#17457=AXIS2_PLACEMENT_3D('',#58078,#22092,#22093) ;
#17458=AXIS2_PLACEMENT_3D('',#58171,#22094,#22095) ;
#17459=AXIS2_PLACEMENT_3D('',#58353,#22096,#22097) ;
#17460=AXIS2_PLACEMENT_3D('',#58535,#22098,#22099) ;
#17461=AXIS2_PLACEMENT_3D('',#58718,#22100,#22101) ;
#17462=AXIS2_PLACEMENT_3D('',#58902,#22102,#22103) ;
#17463=AXIS2_PLACEMENT_3D('',#59084,#22104,#22105) ;
#17464=AXIS2_PLACEMENT_3D('',#59266,#22106,#22107) ;
#17465=AXIS2_PLACEMENT_3D('',#59450,#22108,#22109) ;
#17466=AXIS2_PLACEMENT_3D('',#59633,#22110,#22111) ;
#17467=AXIS2_PLACEMENT_3D('',#59815,#22112,#22113) ;
#17468=AXIS2_PLACEMENT_3D('',#59998,#22114,#22115) ;
#17469=AXIS2_PLACEMENT_3D('',#60182,#22116,#22117) ;
#17470=AXIS2_PLACEMENT_3D('',#60364,#22118,#22119) ;
#17471=AXIS2_PLACEMENT_3D('',#60546,#22120,#22121) ;
#17472=AXIS2_PLACEMENT_3D('',#60730,#22122,#22123) ;
#17473=AXIS2_PLACEMENT_3D('',#60912,#22124,#22125) ;
#17474=AXIS2_PLACEMENT_3D('',#61094,#22126,#22127) ;
#17475=AXIS2_PLACEMENT_3D('',#61277,#22128,#22129) ;
#17476=AXIS2_PLACEMENT_3D('',#61461,#22130,#22131) ;
#17477=AXIS2_PLACEMENT_3D('',#61643,#22132,#22133) ;
#17478=AXIS2_PLACEMENT_3D('',#61825,#22134,#22135) ;
#17479=AXIS2_PLACEMENT_3D('',#62009,#22136,#22137) ;
#17480=AXIS2_PLACEMENT_3D('',#62192,#22138,#22139) ;
#17481=AXIS2_PLACEMENT_3D('',#62374,#22140,#22141) ;
#17482=AXIS2_PLACEMENT_3D('',#62557,#22142,#22143) ;
#17483=AXIS2_PLACEMENT_3D('',#62741,#22144,#22145) ;
#17484=AXIS2_PLACEMENT_3D('',#62923,#22146,#22147) ;
#17485=AXIS2_PLACEMENT_3D('',#63105,#22148,#22149) ;
#17486=AXIS2_PLACEMENT_3D('',#63287,#22150,#22151) ;
#17487=AXIS2_PLACEMENT_3D('',#63289,#22152,#22153) ;
#17488=AXIS2_PLACEMENT_3D('',#63292,#22155,#22156) ;
#17489=AXIS2_PLACEMENT_3D('',#63293,#22157,#22158) ;
#17490=AXIS2_PLACEMENT_3D('',#63295,#22159,#22160) ;
#17491=AXIS2_PLACEMENT_3D('',#63297,#22161,#22162) ;
#17492=AXIS2_PLACEMENT_3D('',#63298,#22163,#22164) ;
#17493=AXIS2_PLACEMENT_3D('',#63299,#22165,#22166) ;
#17494=AXIS2_PLACEMENT_3D('',#63301,#22167,#22168) ;
#17495=AXIS2_PLACEMENT_3D('',#63303,#22169,#22170) ;
#17496=AXIS2_PLACEMENT_3D('',#63304,#22171,#22172) ;
#17497=AXIS2_PLACEMENT_3D('',#63305,#22173,#22174) ;
#17498=AXIS2_PLACEMENT_3D('',#63307,#22175,#22176) ;
#17499=AXIS2_PLACEMENT_3D('',#63309,#22177,#22178) ;
#17500=AXIS2_PLACEMENT_3D('',#63310,#22179,#22180) ;
#17501=AXIS2_PLACEMENT_3D('',#63311,#22181,#22182) ;
#17502=AXIS2_PLACEMENT_3D('',#63314,#22184,#22185) ;
#17503=AXIS2_PLACEMENT_3D('',#63315,#22186,#22187) ;
#17504=AXIS2_PLACEMENT_3D('',#63317,#22188,#22189) ;
#17505=AXIS2_PLACEMENT_3D('',#63318,#22190,#22191) ;
#17506=AXIS2_PLACEMENT_3D('',#63319,#22192,#22193) ;
#17507=AXIS2_PLACEMENT_3D('',#63321,#22195,#22196) ;
#17508=AXIS2_PLACEMENT_3D('',#63322,#22197,#22198) ;
#17509=AXIS2_PLACEMENT_3D('',#63323,#22199,#22200) ;
#17510=AXIS2_PLACEMENT_3D('',#63324,#22201,#22202) ;
#17511=AXIS2_PLACEMENT_3D('',#63325,#22203,#22204) ;
#17512=AXIS2_PLACEMENT_3D('',#63326,#22205,#22206) ;
#17513=AXIS2_PLACEMENT_3D('',#63327,#22207,#22208) ;
#17514=AXIS2_PLACEMENT_3D('',#63328,#22209,#22210) ;
#17515=AXIS2_PLACEMENT_3D('',#63329,#22211,#22212) ;
#17516=AXIS2_PLACEMENT_3D('',#63330,#22213,#22214) ;
#17517=AXIS2_PLACEMENT_3D('',#63331,#22215,#22216) ;
#17518=AXIS2_PLACEMENT_3D('',#63332,#22217,#22218) ;
#17519=AXIS2_PLACEMENT_3D('',#63333,#22219,#22220) ;
#17520=AXIS2_PLACEMENT_3D('',#63334,#22221,#22222) ;
#17521=AXIS2_PLACEMENT_3D('',#63335,#22223,#22224) ;
#17522=AXIS2_PLACEMENT_3D('',#63336,#22225,#22226) ;
#17523=AXIS2_PLACEMENT_3D('',#63337,#22227,#22228) ;
#17524=AXIS2_PLACEMENT_3D('',#63338,#22229,#22230) ;
#17525=AXIS2_PLACEMENT_3D('',#63339,#22231,#22232) ;
#17526=AXIS2_PLACEMENT_3D('',#63340,#22233,#22234) ;
#17527=AXIS2_PLACEMENT_3D('',#63341,#22235,#22236) ;
#17528=AXIS2_PLACEMENT_3D('',#63342,#22237,#22238) ;
#17529=AXIS2_PLACEMENT_3D('',#63343,#22239,#22240) ;
#17530=AXIS2_PLACEMENT_3D('',#63344,#22241,#22242) ;
#17531=AXIS2_PLACEMENT_3D('',#63345,#22243,#22244) ;
#17532=AXIS2_PLACEMENT_3D('',#63346,#22245,#22246) ;
#17533=AXIS2_PLACEMENT_3D('',#63347,#22247,#22248) ;
#17534=AXIS2_PLACEMENT_3D('',#63348,#22249,#22250) ;
#17535=AXIS2_PLACEMENT_3D('',#63349,#22251,#22252) ;
#17536=AXIS2_PLACEMENT_3D('',#63350,#22253,#22254) ;
#17537=AXIS2_PLACEMENT_3D('',#63351,#22255,#22256) ;
#17538=AXIS2_PLACEMENT_3D('',#63352,#22257,#22258) ;
#17539=AXIS2_PLACEMENT_3D('',#63353,#22259,#22260) ;
#17540=AXIS2_PLACEMENT_3D('',#63354,#22261,#22262) ;
#17541=AXIS2_PLACEMENT_3D('',#63355,#22263,#22264) ;
#17542=AXIS2_PLACEMENT_3D('',#63356,#22265,#22266) ;
#17543=AXIS2_PLACEMENT_3D('',#63357,#22267,#22268) ;
#17544=AXIS2_PLACEMENT_3D('',#63358,#22269,#22270) ;
#17545=AXIS2_PLACEMENT_3D('',#63359,#22271,#22272) ;
#17546=AXIS2_PLACEMENT_3D('',#63360,#22273,#22274) ;
#17547=AXIS2_PLACEMENT_3D('',#63361,#22275,#22276) ;
#17548=AXIS2_PLACEMENT_3D('',#63362,#22277,#22278) ;
#17549=AXIS2_PLACEMENT_3D('',#63363,#22279,#22280) ;
#17550=AXIS2_PLACEMENT_3D('',#63364,#22281,#22282) ;
#17551=AXIS2_PLACEMENT_3D('',#63365,#22283,#22284) ;
#17552=AXIS2_PLACEMENT_3D('',#63366,#22285,#22286) ;
#17553=AXIS2_PLACEMENT_3D('',#63367,#22287,#22288) ;
#17554=AXIS2_PLACEMENT_3D('',#63368,#22289,#22290) ;
#17555=AXIS2_PLACEMENT_3D('',#63369,#22291,#22292) ;
#17556=AXIS2_PLACEMENT_3D('',#63370,#22293,#22294) ;
#17557=AXIS2_PLACEMENT_3D('',#63371,#22295,#22296) ;
#17558=AXIS2_PLACEMENT_3D('',#63372,#22297,#22298) ;
#17559=AXIS2_PLACEMENT_3D('',#63373,#22299,#22300) ;
#17560=AXIS2_PLACEMENT_3D('',#63374,#22301,#22302) ;
#17561=AXIS2_PLACEMENT_3D('',#63375,#22303,#22304) ;
#17562=AXIS2_PLACEMENT_3D('',#63376,#22305,#22306) ;
#17563=AXIS2_PLACEMENT_3D('',#63377,#22307,#22308) ;
#17564=AXIS2_PLACEMENT_3D('',#63378,#22309,#22310) ;
#17565=AXIS2_PLACEMENT_3D('',#63379,#22311,#22312) ;
#17566=AXIS2_PLACEMENT_3D('',#63380,#22313,#22314) ;
#17567=AXIS2_PLACEMENT_3D('',#63381,#22315,#22316) ;
#17568=AXIS2_PLACEMENT_3D('',#63382,#22317,#22318) ;
#17569=AXIS2_PLACEMENT_3D('',#63383,#22319,#22320) ;
#17570=AXIS2_PLACEMENT_3D('',#63384,#22321,#22322) ;
#17571=AXIS2_PLACEMENT_3D('',#63385,#22323,#22324) ;
#17572=AXIS2_PLACEMENT_3D('',#63386,#22325,#22326) ;
#17573=AXIS2_PLACEMENT_3D('',#63387,#22327,#22328) ;
#17574=AXIS2_PLACEMENT_3D('',#63388,#22329,#22330) ;
#17575=AXIS2_PLACEMENT_3D('',#63389,#22331,#22332) ;
#17576=AXIS2_PLACEMENT_3D('',#63390,#22333,#22334) ;
#17577=AXIS2_PLACEMENT_3D('',#63391,#22335,#22336) ;
#17578=AXIS2_PLACEMENT_3D('',#63392,#22337,#22338) ;
#17579=AXIS2_PLACEMENT_3D('',#63393,#22339,#22340) ;
#17580=AXIS2_PLACEMENT_3D('',#63394,#22341,#22342) ;
#17581=AXIS2_PLACEMENT_3D('',#63395,#22343,#22344) ;
#17582=AXIS2_PLACEMENT_3D('',#63396,#22345,#22346) ;
#17583=AXIS2_PLACEMENT_3D('',#63397,#22347,#22348) ;
#17584=AXIS2_PLACEMENT_3D('',#63398,#22349,#22350) ;
#17585=AXIS2_PLACEMENT_3D('',#63399,#22351,#22352) ;
#17586=AXIS2_PLACEMENT_3D('',#63400,#22353,#22354) ;
#17587=AXIS2_PLACEMENT_3D('',#63401,#22355,#22356) ;
#17588=AXIS2_PLACEMENT_3D('',#63402,#22357,#22358) ;
#17589=AXIS2_PLACEMENT_3D('',#63403,#22359,#22360) ;
#17590=AXIS2_PLACEMENT_3D('',#63404,#22361,#22362) ;
#17591=AXIS2_PLACEMENT_3D('',#63405,#22363,#22364) ;
#17592=AXIS2_PLACEMENT_3D('',#63406,#22365,#22366) ;
#17593=AXIS2_PLACEMENT_3D('',#63407,#22367,#22368) ;
#17594=AXIS2_PLACEMENT_3D('',#63408,#22369,#22370) ;
#17595=AXIS2_PLACEMENT_3D('',#63409,#22371,#22372) ;
#17596=AXIS2_PLACEMENT_3D('',#63410,#22373,#22374) ;
#17597=AXIS2_PLACEMENT_3D('',#63411,#22375,#22376) ;
#17598=AXIS2_PLACEMENT_3D('',#63412,#22377,#22378) ;
#17599=AXIS2_PLACEMENT_3D('',#63414,#22380,#22381) ;
#17600=AXIS2_PLACEMENT_3D('',#63415,#22382,#22383) ;
#17601=AXIS2_PLACEMENT_3D('',#63416,#22384,#22385) ;
#17602=AXIS2_PLACEMENT_3D('',#63417,#22386,#22387) ;
#17603=AXIS2_PLACEMENT_3D('',#63418,#22388,#22389) ;
#17604=AXIS2_PLACEMENT_3D('',#63419,#22390,#22391) ;
#17605=AXIS2_PLACEMENT_3D('',#63420,#22392,#22393) ;
#17606=AXIS2_PLACEMENT_3D('',#63421,#22394,#22395) ;
#17607=AXIS2_PLACEMENT_3D('',#63422,#22396,#22397) ;
#17608=AXIS2_PLACEMENT_3D('',#63423,#22398,#22399) ;
#17609=AXIS2_PLACEMENT_3D('',#63424,#22400,#22401) ;
#17610=AXIS2_PLACEMENT_3D('',#63425,#22402,#22403) ;
#17611=AXIS2_PLACEMENT_3D('',#63426,#22404,#22405) ;
#17612=AXIS2_PLACEMENT_3D('',#63427,#22406,#22407) ;
#17613=AXIS2_PLACEMENT_3D('',#63428,#22408,#22409) ;
#17614=AXIS2_PLACEMENT_3D('',#63429,#22410,#22411) ;
#17615=AXIS2_PLACEMENT_3D('',#63430,#22412,#22413) ;
#17616=AXIS2_PLACEMENT_3D('',#63431,#22414,#22415) ;
#17617=AXIS2_PLACEMENT_3D('',#63432,#22416,#22417) ;
#17618=AXIS2_PLACEMENT_3D('',#63433,#22418,#22419) ;
#17619=AXIS2_PLACEMENT_3D('',#63434,#22420,#22421) ;
#17620=AXIS2_PLACEMENT_3D('',#63435,#22422,#22423) ;
#17621=AXIS2_PLACEMENT_3D('',#63436,#22424,#22425) ;
#17622=AXIS2_PLACEMENT_3D('',#63437,#22426,#22427) ;
#17623=AXIS2_PLACEMENT_3D('',#63438,#22428,#22429) ;
#17624=AXIS2_PLACEMENT_3D('',#63439,#22430,#22431) ;
#17625=AXIS2_PLACEMENT_3D('',#63440,#22432,#22433) ;
#17626=AXIS2_PLACEMENT_3D('',#63441,#22434,#22435) ;
#17627=AXIS2_PLACEMENT_3D('',#63442,#22436,#22437) ;
#17628=AXIS2_PLACEMENT_3D('',#63443,#22438,#22439) ;
#17629=AXIS2_PLACEMENT_3D('',#63444,#22440,#22441) ;
#17630=AXIS2_PLACEMENT_3D('',#63445,#22442,#22443) ;
#17631=AXIS2_PLACEMENT_3D('',#63446,#22444,#22445) ;
#17632=AXIS2_PLACEMENT_3D('',#63447,#22446,#22447) ;
#17633=AXIS2_PLACEMENT_3D('',#63448,#22448,#22449) ;
#17634=AXIS2_PLACEMENT_3D('',#63449,#22450,#22451) ;
#17635=AXIS2_PLACEMENT_3D('',#63450,#22452,#22453) ;
#17636=AXIS2_PLACEMENT_3D('',#63451,#22454,#22455) ;
#17637=AXIS2_PLACEMENT_3D('',#63452,#22456,#22457) ;
#17638=AXIS2_PLACEMENT_3D('',#63453,#22458,#22459) ;
#17639=AXIS2_PLACEMENT_3D('',#63454,#22460,#22461) ;
#17640=AXIS2_PLACEMENT_3D('',#63455,#22462,#22463) ;
#17641=AXIS2_PLACEMENT_3D('',#63456,#22464,#22465) ;
#17642=AXIS2_PLACEMENT_3D('',#63457,#22466,#22467) ;
#17643=AXIS2_PLACEMENT_3D('',#63458,#22468,#22469) ;
#17644=AXIS2_PLACEMENT_3D('',#63459,#22470,#22471) ;
#17645=AXIS2_PLACEMENT_3D('',#63460,#22472,#22473) ;
#17646=AXIS2_PLACEMENT_3D('',#63461,#22474,#22475) ;
#17647=AXIS2_PLACEMENT_3D('',#63462,#22476,#22477) ;
#17648=AXIS2_PLACEMENT_3D('',#63463,#22478,#22479) ;
#17649=AXIS2_PLACEMENT_3D('',#63464,#22480,#22481) ;
#17650=AXIS2_PLACEMENT_3D('',#63465,#22482,#22483) ;
#17651=AXIS2_PLACEMENT_3D('',#63466,#22484,#22485) ;
#17652=AXIS2_PLACEMENT_3D('',#63467,#22486,#22487) ;
#17653=AXIS2_PLACEMENT_3D('',#63468,#22488,#22489) ;
#17654=AXIS2_PLACEMENT_3D('',#63469,#22490,#22491) ;
#17655=AXIS2_PLACEMENT_3D('',#63470,#22492,#22493) ;
#17656=AXIS2_PLACEMENT_3D('',#63471,#22494,#22495) ;
#17657=AXIS2_PLACEMENT_3D('',#63472,#22496,#22497) ;
#17658=AXIS2_PLACEMENT_3D('',#63473,#22498,#22499) ;
#17659=AXIS2_PLACEMENT_3D('',#63474,#22500,#22501) ;
#17660=AXIS2_PLACEMENT_3D('',#63475,#22502,#22503) ;
#17661=AXIS2_PLACEMENT_3D('',#63476,#22504,#22505) ;
#17662=AXIS2_PLACEMENT_3D('',#63477,#22506,#22507) ;
#17663=AXIS2_PLACEMENT_3D('',#63478,#22508,#22509) ;
#17664=AXIS2_PLACEMENT_3D('',#63479,#22510,#22511) ;
#17665=AXIS2_PLACEMENT_3D('',#63480,#22512,#22513) ;
#17666=AXIS2_PLACEMENT_3D('',#63481,#22514,#22515) ;
#17667=AXIS2_PLACEMENT_3D('',#63482,#22516,#22517) ;
#17668=AXIS2_PLACEMENT_3D('',#63483,#22518,#22519) ;
#17669=AXIS2_PLACEMENT_3D('',#63484,#22520,#22521) ;
#17670=AXIS2_PLACEMENT_3D('',#63485,#22522,#22523) ;
#17671=AXIS2_PLACEMENT_3D('',#63486,#22524,#22525) ;
#17672=AXIS2_PLACEMENT_3D('',#63487,#22526,#22527) ;
#17673=AXIS2_PLACEMENT_3D('',#63488,#22528,#22529) ;
#17674=AXIS2_PLACEMENT_3D('',#63489,#22530,#22531) ;
#17675=AXIS2_PLACEMENT_3D('',#63490,#22532,#22533) ;
#17676=AXIS2_PLACEMENT_3D('',#63491,#22534,#22535) ;
#17677=AXIS2_PLACEMENT_3D('',#63492,#22536,#22537) ;
#17678=AXIS2_PLACEMENT_3D('',#63493,#22538,#22539) ;
#17679=AXIS2_PLACEMENT_3D('',#63494,#22540,#22541) ;
#17680=AXIS2_PLACEMENT_3D('',#63495,#22542,#22543) ;
#17681=AXIS2_PLACEMENT_3D('',#63496,#22544,#22545) ;
#17682=AXIS2_PLACEMENT_3D('',#63497,#22546,#22547) ;
#17683=AXIS2_PLACEMENT_3D('',#63498,#22548,#22549) ;
#17684=AXIS2_PLACEMENT_3D('',#63499,#22550,#22551) ;
#17685=AXIS2_PLACEMENT_3D('',#63500,#22552,#22553) ;
#17686=AXIS2_PLACEMENT_3D('',#63501,#22554,#22555) ;
#17687=AXIS2_PLACEMENT_3D('',#63502,#22556,#22557) ;
#17688=AXIS2_PLACEMENT_3D('',#63503,#22558,#22559) ;
#17689=AXIS2_PLACEMENT_3D('',#63504,#22560,#22561) ;
#17690=AXIS2_PLACEMENT_3D('',#63505,#22562,#22563) ;
#17691=AXIS2_PLACEMENT_3D('',#63506,#22564,#22565) ;
#17692=AXIS2_PLACEMENT_3D('',#63507,#22566,#22567) ;
#17693=AXIS2_PLACEMENT_3D('',#63508,#22568,#22569) ;
#17694=AXIS2_PLACEMENT_3D('',#63509,#22570,#22571) ;
#17695=AXIS2_PLACEMENT_3D('',#63510,#22572,#22573) ;
#17696=AXIS2_PLACEMENT_3D('',#63511,#22574,#22575) ;
#17697=AXIS2_PLACEMENT_3D('',#63512,#22576,#22577) ;
#17698=AXIS2_PLACEMENT_3D('',#63513,#22578,#22579) ;
#17699=AXIS2_PLACEMENT_3D('',#63514,#22580,#22581) ;
#17700=AXIS2_PLACEMENT_3D('',#63515,#22582,#22583) ;
#17701=AXIS2_PLACEMENT_3D('',#63516,#22584,#22585) ;
#17702=AXIS2_PLACEMENT_3D('',#63517,#22586,#22587) ;
#17703=AXIS2_PLACEMENT_3D('',#63518,#22588,#22589) ;
#17704=AXIS2_PLACEMENT_3D('',#63519,#22590,#22591) ;
#17705=AXIS2_PLACEMENT_3D('',#63520,#22592,#22593) ;
#17706=AXIS2_PLACEMENT_3D('',#63521,#22594,#22595) ;
#17707=AXIS2_PLACEMENT_3D('',#63522,#22596,#22597) ;
#17708=AXIS2_PLACEMENT_3D('',#63523,#22598,#22599) ;
#17709=AXIS2_PLACEMENT_3D('',#63524,#22600,#22601) ;
#17710=AXIS2_PLACEMENT_3D('',#63525,#22602,#22603) ;
#17711=AXIS2_PLACEMENT_3D('',#63526,#22604,#22605) ;
#17712=AXIS2_PLACEMENT_3D('',#63527,#22606,#22607) ;
#17713=AXIS2_PLACEMENT_3D('',#63528,#22608,#22609) ;
#17714=AXIS2_PLACEMENT_3D('',#63529,#22610,#22611) ;
#17715=AXIS2_PLACEMENT_3D('',#63530,#22612,#22613) ;
#17716=AXIS2_PLACEMENT_3D('',#63531,#22614,#22615) ;
#17717=AXIS2_PLACEMENT_3D('',#63532,#22616,#22617) ;
#17718=AXIS2_PLACEMENT_3D('',#63533,#22618,#22619) ;
#17719=AXIS2_PLACEMENT_3D('',#63534,#22620,#22621) ;
#17720=AXIS2_PLACEMENT_3D('',#63535,#22622,#22623) ;
#17721=AXIS2_PLACEMENT_3D('',#63536,#22624,#22625) ;
#17722=AXIS2_PLACEMENT_3D('',#63537,#22626,#22627) ;
#17723=AXIS2_PLACEMENT_3D('',#63538,#22628,#22629) ;
#17724=AXIS2_PLACEMENT_3D('',#63539,#22630,#22631) ;
#17725=AXIS2_PLACEMENT_3D('',#63540,#22632,#22633) ;
#17726=AXIS2_PLACEMENT_3D('',#63541,#22634,#22635) ;
#17727=AXIS2_PLACEMENT_3D('',#63542,#22636,#22637) ;
#17728=AXIS2_PLACEMENT_3D('',#63543,#22638,#22639) ;
#17729=AXIS2_PLACEMENT_3D('',#63544,#22640,#22641) ;
#17730=AXIS2_PLACEMENT_3D('',#63545,#22642,#22643) ;
#17731=AXIS2_PLACEMENT_3D('',#63546,#22644,#22645) ;
#17732=AXIS2_PLACEMENT_3D('',#63547,#22646,#22647) ;
#17733=AXIS2_PLACEMENT_3D('',#63548,#22648,#22649) ;
#17734=AXIS2_PLACEMENT_3D('',#63549,#22650,#22651) ;
#17735=AXIS2_PLACEMENT_3D('',#63550,#22652,#22653) ;
#17736=AXIS2_PLACEMENT_3D('',#63551,#22654,#22655) ;
#17737=AXIS2_PLACEMENT_3D('',#63552,#22656,#22657) ;
#17738=AXIS2_PLACEMENT_3D('',#63553,#22658,#22659) ;
#17739=AXIS2_PLACEMENT_3D('',#63554,#22660,#22661) ;
#17740=AXIS2_PLACEMENT_3D('',#63555,#22662,#22663) ;
#17741=AXIS2_PLACEMENT_3D('',#63556,#22664,#22665) ;
#17742=AXIS2_PLACEMENT_3D('',#63557,#22666,#22667) ;
#17743=AXIS2_PLACEMENT_3D('',#63558,#22668,#22669) ;
#17744=AXIS2_PLACEMENT_3D('',#63559,#22670,#22671) ;
#17745=AXIS2_PLACEMENT_3D('',#63560,#22672,#22673) ;
#17746=AXIS2_PLACEMENT_3D('',#63561,#22674,#22675) ;
#17747=AXIS2_PLACEMENT_3D('',#63562,#22676,#22677) ;
#17748=AXIS2_PLACEMENT_3D('',#63563,#22678,#22679) ;
#17749=AXIS2_PLACEMENT_3D('',#63564,#22680,#22681) ;
#17750=AXIS2_PLACEMENT_3D('',#63565,#22682,#22683) ;
#17751=AXIS2_PLACEMENT_3D('',#63566,#22684,#22685) ;
#17752=AXIS2_PLACEMENT_3D('',#63567,#22686,#22687) ;
#17753=AXIS2_PLACEMENT_3D('',#63568,#22688,#22689) ;
#17754=AXIS2_PLACEMENT_3D('',#63569,#22690,#22691) ;
#17755=AXIS2_PLACEMENT_3D('',#63570,#22692,#22693) ;
#17756=AXIS2_PLACEMENT_3D('',#63571,#22694,#22695) ;
#17757=AXIS2_PLACEMENT_3D('',#63572,#22696,#22697) ;
#17758=AXIS2_PLACEMENT_3D('',#63573,#22698,#22699) ;
#17759=AXIS2_PLACEMENT_3D('',#63574,#22700,#22701) ;
#17760=AXIS2_PLACEMENT_3D('',#63575,#22702,#22703) ;
#17761=AXIS2_PLACEMENT_3D('',#63576,#22704,#22705) ;
#17762=AXIS2_PLACEMENT_3D('',#63577,#22706,#22707) ;
#17763=AXIS2_PLACEMENT_3D('',#63578,#22708,#22709) ;
#17764=AXIS2_PLACEMENT_3D('',#63579,#22710,#22711) ;
#17765=AXIS2_PLACEMENT_3D('',#63580,#22712,#22713) ;
#17766=AXIS2_PLACEMENT_3D('',#63581,#22714,#22715) ;
#17767=AXIS2_PLACEMENT_3D('',#63582,#22716,#22717) ;
#17768=AXIS2_PLACEMENT_3D('',#63583,#22718,#22719) ;
#17769=AXIS2_PLACEMENT_3D('',#63584,#22720,#22721) ;
#17770=AXIS2_PLACEMENT_3D('',#63585,#22722,#22723) ;
#17771=AXIS2_PLACEMENT_3D('',#63586,#22724,#22725) ;
#17772=AXIS2_PLACEMENT_3D('',#63587,#22726,#22727) ;
#17773=AXIS2_PLACEMENT_3D('',#63588,#22728,#22729) ;
#17774=AXIS2_PLACEMENT_3D('',#63589,#22730,#22731) ;
#17775=AXIS2_PLACEMENT_3D('',#63590,#22732,#22733) ;
#17776=AXIS2_PLACEMENT_3D('',#63591,#22734,#22735) ;
#17777=AXIS2_PLACEMENT_3D('',#63592,#22736,#22737) ;
#17778=AXIS2_PLACEMENT_3D('',#63593,#22738,#22739) ;
#17779=AXIS2_PLACEMENT_3D('',#63594,#22740,#22741) ;
#17780=AXIS2_PLACEMENT_3D('',#63595,#22742,#22743) ;
#17781=AXIS2_PLACEMENT_3D('',#63596,#22744,#22745) ;
#17782=AXIS2_PLACEMENT_3D('',#63597,#22746,#22747) ;
#17783=AXIS2_PLACEMENT_3D('',#63598,#22748,#22749) ;
#17784=AXIS2_PLACEMENT_3D('',#63599,#22750,#22751) ;
#17785=AXIS2_PLACEMENT_3D('',#63600,#22752,#22753) ;
#17786=AXIS2_PLACEMENT_3D('',#63601,#22754,#22755) ;
#17787=AXIS2_PLACEMENT_3D('',#63602,#22756,#22757) ;
#17788=AXIS2_PLACEMENT_3D('',#63603,#22758,#22759) ;
#17789=AXIS2_PLACEMENT_3D('',#63604,#22760,#22761) ;
#17790=AXIS2_PLACEMENT_3D('',#63605,#22762,#22763) ;
#17791=AXIS2_PLACEMENT_3D('',#63606,#22764,#22765) ;
#17792=AXIS2_PLACEMENT_3D('',#63607,#22766,#22767) ;
#17793=AXIS2_PLACEMENT_3D('',#63608,#22768,#22769) ;
#17794=AXIS2_PLACEMENT_3D('',#63609,#22770,#22771) ;
#17795=AXIS2_PLACEMENT_3D('',#63610,#22772,#22773) ;
#17796=AXIS2_PLACEMENT_3D('',#63611,#22774,#22775) ;
#17797=AXIS2_PLACEMENT_3D('',#63612,#22776,#22777) ;
#17798=AXIS2_PLACEMENT_3D('',#63613,#22778,#22779) ;
#17799=AXIS2_PLACEMENT_3D('',#63614,#22780,#22781) ;
#17800=AXIS2_PLACEMENT_3D('',#63615,#22782,#22783) ;
#17801=AXIS2_PLACEMENT_3D('',#63616,#22784,#22785) ;
#21660=DIRECTION('axis',(0.,0.,1.)) ;
#21661=DIRECTION('refdir',(1.,0.,0.)) ;
#21662=DIRECTION('center_axis',(1.83697019872103E-16,1.,0.)) ;
#21663=DIRECTION('ref_axis',(6.12323399573677E-17,-1.12481983699639E-32,
1.)) ;
#21664=DIRECTION('center_axis',(1.83697019872103E-16,1.,1.82109527525433E-48)) ;
#21665=DIRECTION('ref_axis',(6.12323399573677E-17,-1.12481983699639E-32,
1.)) ;
#21666=DIRECTION('',(-1.46793425709383E-16,0.183848416855218,-0.982954607100364)) ;
#21667=DIRECTION('center_axis',(1.83697019872103E-16,1.,0.)) ;
#21668=DIRECTION('ref_axis',(6.12323399573677E-17,-1.12481983699639E-32,
1.)) ;
#21669=DIRECTION('center_axis',(1.83697019872103E-16,1.,0.)) ;
#21670=DIRECTION('ref_axis',(6.12323399573677E-17,-1.12481983699639E-32,
1.)) ;
#21671=DIRECTION('center_axis',(1.83697019872103E-16,1.,0.)) ;
#21672=DIRECTION('ref_axis',(6.12323399573677E-17,-1.12481983699639E-32,
1.)) ;
#21673=DIRECTION('center_axis',(1.83697019872103E-16,1.,0.)) ;
#21674=DIRECTION('ref_axis',(6.12323399573677E-17,-1.12481983699639E-32,
1.)) ;
#21675=DIRECTION('center_axis',(1.83697019872103E-16,1.,0.)) ;
#21676=DIRECTION('ref_axis',(6.12323399573677E-17,-1.12481983699639E-32,
1.)) ;
#21677=DIRECTION('center_axis',(1.83697019872103E-16,1.,0.)) ;
#21678=DIRECTION('ref_axis',(6.12323399573677E-17,-1.12481983699639E-32,
1.)) ;
#21679=DIRECTION('center_axis',(1.83697019872103E-16,1.,0.)) ;
#21680=DIRECTION('ref_axis',(6.12323399573677E-17,-1.12481983699639E-32,
1.)) ;
#21681=DIRECTION('center_axis',(1.83697019872103E-16,1.,0.)) ;
#21682=DIRECTION('ref_axis',(6.12323399573677E-17,-1.12481983699639E-32,
1.)) ;
#21683=DIRECTION('center_axis',(1.83697019872103E-16,1.,0.)) ;
#21684=DIRECTION('ref_axis',(6.12323399573677E-17,-1.12481983699639E-32,
1.)) ;
#21685=DIRECTION('center_axis',(1.83697019872103E-16,1.,0.)) ;
#21686=DIRECTION('ref_axis',(6.12323399573677E-17,-1.12481983699639E-32,
1.)) ;
#21687=DIRECTION('center_axis',(1.83697019872103E-16,1.,0.)) ;
#21688=DIRECTION('ref_axis',(6.12323399573677E-17,-1.12481983699639E-32,
1.)) ;
#21689=DIRECTION('center_axis',(1.83697019872103E-16,1.,0.)) ;
#21690=DIRECTION('ref_axis',(6.12323399573677E-17,-1.12481983699639E-32,
1.)) ;
#21691=DIRECTION('center_axis',(1.83697019872103E-16,1.,0.)) ;
#21692=DIRECTION('ref_axis',(6.12323399573677E-17,-1.12481983699639E-32,
1.)) ;
#21693=DIRECTION('center_axis',(1.83697019872103E-16,1.,0.)) ;
#21694=DIRECTION('ref_axis',(6.12323399573677E-17,-1.12481983699639E-32,
1.)) ;
#21695=DIRECTION('center_axis',(1.83697019872103E-16,1.,0.)) ;
#21696=DIRECTION('ref_axis',(6.12323399573677E-17,-1.12481983699639E-32,
1.)) ;
#21697=DIRECTION('center_axis',(1.83697019872103E-16,1.,0.)) ;
#21698=DIRECTION('ref_axis',(6.12323399573677E-17,-1.12481983699639E-32,
1.)) ;
#21699=DIRECTION('center_axis',(1.83697019872103E-16,1.,0.)) ;
#21700=DIRECTION('ref_axis',(6.12323399573677E-17,-1.12481983699639E-32,
1.)) ;
#21701=DIRECTION('center_axis',(1.83697019872103E-16,1.,0.)) ;
#21702=DIRECTION('ref_axis',(6.12323399573677E-17,-1.12481983699639E-32,
1.)) ;
#21703=DIRECTION('center_axis',(1.83697019872103E-16,1.,0.)) ;
#21704=DIRECTION('ref_axis',(6.12323399573677E-17,-1.12481983699639E-32,
1.)) ;
#21705=DIRECTION('center_axis',(1.83697019872103E-16,1.,0.)) ;
#21706=DIRECTION('ref_axis',(6.12323399573677E-17,-1.12481983699639E-32,
1.)) ;
#21707=DIRECTION('center_axis',(1.83697019872103E-16,1.,0.)) ;
#21708=DIRECTION('ref_axis',(6.12323399573677E-17,-1.12481983699639E-32,
1.)) ;
#21709=DIRECTION('center_axis',(1.83697019872103E-16,1.,0.)) ;
#21710=DIRECTION('ref_axis',(6.12323399573677E-17,-1.12481983699639E-32,
1.)) ;
#21711=DIRECTION('center_axis',(1.83697019872103E-16,1.,0.)) ;
#21712=DIRECTION('ref_axis',(6.12323399573677E-17,-1.12481983699639E-32,
1.)) ;
#21713=DIRECTION('center_axis',(1.83697019872103E-16,1.,0.)) ;
#21714=DIRECTION('ref_axis',(6.12323399573677E-17,-1.12481983699639E-32,
1.)) ;
#21715=DIRECTION('center_axis',(1.83697019872103E-16,1.,0.)) ;
#21716=DIRECTION('ref_axis',(6.12323399573677E-17,-1.12481983699639E-32,
1.)) ;
#21717=DIRECTION('center_axis',(1.83697019872103E-16,1.,0.)) ;
#21718=DIRECTION('ref_axis',(6.12323399573677E-17,-1.12481983699639E-32,
1.)) ;
#21719=DIRECTION('center_axis',(1.83697019872103E-16,1.,0.)) ;
#21720=DIRECTION('ref_axis',(6.12323399573677E-17,-1.12481983699639E-32,
1.)) ;
#21721=DIRECTION('center_axis',(1.83697019872103E-16,1.,0.)) ;
#21722=DIRECTION('ref_axis',(6.12323399573677E-17,-1.12481983699639E-32,
1.)) ;
#21723=DIRECTION('center_axis',(1.83697019872103E-16,1.,0.)) ;
#21724=DIRECTION('ref_axis',(6.12323399573677E-17,-1.12481983699639E-32,
1.)) ;
#21725=DIRECTION('center_axis',(1.83697019872103E-16,1.,0.)) ;
#21726=DIRECTION('ref_axis',(6.12323399573677E-17,-1.12481983699639E-32,
1.)) ;
#21727=DIRECTION('center_axis',(1.83697019872103E-16,1.,0.)) ;
#21728=DIRECTION('ref_axis',(6.12323399573677E-17,-1.12481983699639E-32,
1.)) ;
#21729=DIRECTION('center_axis',(1.83697019872103E-16,1.,0.)) ;
#21730=DIRECTION('ref_axis',(6.12323399573677E-17,-1.12481983699639E-32,
1.)) ;
#21731=DIRECTION('center_axis',(1.83697019872103E-16,1.,0.)) ;
#21732=DIRECTION('ref_axis',(6.12323399573677E-17,-1.12481983699639E-32,
1.)) ;
#21733=DIRECTION('center_axis',(1.83697019872103E-16,1.,0.)) ;
#21734=DIRECTION('ref_axis',(6.12323399573677E-17,-1.12481983699639E-32,
1.)) ;
#21735=DIRECTION('center_axis',(1.83697019872103E-16,1.,0.)) ;
#21736=DIRECTION('ref_axis',(6.12323399573677E-17,-1.12481983699639E-32,
1.)) ;
#21737=DIRECTION('center_axis',(1.83697019872103E-16,1.,0.)) ;
#21738=DIRECTION('ref_axis',(6.12323399573677E-17,-1.12481983699639E-32,
1.)) ;
#21739=DIRECTION('center_axis',(1.83697019872103E-16,1.,0.)) ;
#21740=DIRECTION('ref_axis',(6.12323399573677E-17,-1.12481983699639E-32,
1.)) ;
#21741=DIRECTION('center_axis',(1.83697019872103E-16,1.,0.)) ;
#21742=DIRECTION('ref_axis',(6.12323399573677E-17,-1.12481983699639E-32,
1.)) ;
#21743=DIRECTION('center_axis',(1.83697019872103E-16,1.,0.)) ;
#21744=DIRECTION('ref_axis',(6.12323399573677E-17,-1.12481983699639E-32,
1.)) ;
#21745=DIRECTION('center_axis',(1.83697019872103E-16,1.,0.)) ;
#21746=DIRECTION('ref_axis',(6.12323399573677E-17,-1.12481983699639E-32,
1.)) ;
#21747=DIRECTION('center_axis',(1.83697019872103E-16,1.,0.)) ;
#21748=DIRECTION('ref_axis',(6.12323399573677E-17,-1.12481983699639E-32,
1.)) ;
#21749=DIRECTION('center_axis',(1.83697019872103E-16,1.,0.)) ;
#21750=DIRECTION('ref_axis',(6.12323399573677E-17,-1.12481983699639E-32,
1.)) ;
#21751=DIRECTION('center_axis',(1.83697019872103E-16,1.,0.)) ;
#21752=DIRECTION('ref_axis',(6.12323399573677E-17,-1.12481983699639E-32,
1.)) ;
#21753=DIRECTION('center_axis',(1.83697019872103E-16,1.,0.)) ;
#21754=DIRECTION('ref_axis',(6.12323399573677E-17,-1.12481983699639E-32,
1.)) ;
#21755=DIRECTION('center_axis',(1.83697019872103E-16,1.,0.)) ;
#21756=DIRECTION('ref_axis',(6.12323399573677E-17,-1.12481983699639E-32,
1.)) ;
#21757=DIRECTION('center_axis',(1.83697019872103E-16,1.,0.)) ;
#21758=DIRECTION('ref_axis',(6.12323399573677E-17,-1.12481983699639E-32,
1.)) ;
#21759=DIRECTION('center_axis',(1.83697019872103E-16,1.,0.)) ;
#21760=DIRECTION('ref_axis',(6.12323399573677E-17,-1.12481983699639E-32,
1.)) ;
#21761=DIRECTION('center_axis',(1.83697019872103E-16,1.,0.)) ;
#21762=DIRECTION('ref_axis',(6.12323399573677E-17,-1.12481983699639E-32,
1.)) ;
#21763=DIRECTION('center_axis',(1.83697019872103E-16,1.,0.)) ;
#21764=DIRECTION('ref_axis',(6.12323399573677E-17,-1.12481983699639E-32,
1.)) ;
#21765=DIRECTION('center_axis',(1.83697019872103E-16,1.,0.)) ;
#21766=DIRECTION('ref_axis',(6.12323399573677E-17,-1.12481983699639E-32,
1.)) ;
#21767=DIRECTION('center_axis',(1.83697019872103E-16,1.,0.)) ;
#21768=DIRECTION('ref_axis',(6.12323399573677E-17,-1.12481983699639E-32,
1.)) ;
#21769=DIRECTION('center_axis',(1.83697019872103E-16,1.,0.)) ;
#21770=DIRECTION('ref_axis',(6.12323399573677E-17,-1.12481983699639E-32,
1.)) ;
#21771=DIRECTION('center_axis',(1.83697019872103E-16,1.,0.)) ;
#21772=DIRECTION('ref_axis',(6.12323399573677E-17,-1.12481983699639E-32,
1.)) ;
#21773=DIRECTION('center_axis',(1.83697019872103E-16,1.,0.)) ;
#21774=DIRECTION('ref_axis',(6.12323399573677E-17,-1.12481983699639E-32,
1.)) ;
#21775=DIRECTION('center_axis',(1.83697019872103E-16,1.,0.)) ;
#21776=DIRECTION('ref_axis',(6.12323399573677E-17,-1.12481983699639E-32,
1.)) ;
#21777=DIRECTION('center_axis',(1.83697019872103E-16,1.,0.)) ;
#21778=DIRECTION('ref_axis',(6.12323399573677E-17,-1.12481983699639E-32,
1.)) ;
#21779=DIRECTION('center_axis',(1.83697019872103E-16,1.,0.)) ;
#21780=DIRECTION('ref_axis',(6.12323399573677E-17,-1.12481983699639E-32,
1.)) ;
#21781=DIRECTION('center_axis',(1.83697019872103E-16,1.,0.)) ;
#21782=DIRECTION('ref_axis',(6.12323399573677E-17,-1.12481983699639E-32,
1.)) ;
#21783=DIRECTION('center_axis',(1.83697019872103E-16,1.,0.)) ;
#21784=DIRECTION('ref_axis',(6.12323399573677E-17,-1.12481983699639E-32,
1.)) ;
#21785=DIRECTION('center_axis',(-1.83697019872103E-16,-1.,0.)) ;
#21786=DIRECTION('ref_axis',(6.12323399573677E-17,-1.12481983699639E-32,
1.)) ;
#21787=DIRECTION('',(1.71053004918302E-16,0.986251982240049,0.165248381316047)) ;
#21788=DIRECTION('center_axis',(1.83697019872103E-16,1.,0.)) ;
#21789=DIRECTION('ref_axis',(6.12323399573677E-17,-1.12481983699639E-32,
1.)) ;
#21790=DIRECTION('center_axis',(-0.0198775103691821,0.982954607100363,0.182770689558513)) ;
#21791=DIRECTION('ref_axis',(0.106276087274991,0.183848416855221,-0.97719248507822)) ;
#21792=DIRECTION('center_axis',(1.83697019872103E-16,1.,0.)) ;
#21793=DIRECTION('ref_axis',(6.12323399573677E-17,-1.12481983699639E-32,
1.)) ;
#21794=DIRECTION('center_axis',(-0.0587030808149488,0.982954607100363,0.174224535249788)) ;
#21795=DIRECTION('ref_axis',(0.313858910101312,0.183848416855221,-0.93150005054742)) ;
#21796=DIRECTION('center_axis',(1.83697019872103E-16,1.,0.)) ;
#21797=DIRECTION('ref_axis',(6.12323399573677E-17,-1.12481983699639E-32,
1.)) ;
#21798=DIRECTION('center_axis',(-0.0947837604455976,0.982954607100363,0.157531835309445)) ;
#21799=DIRECTION('ref_axis',(0.506766039120339,0.183848416855219,-0.842251708941046)) ;
#21800=DIRECTION('center_axis',(1.83697019872103E-16,1.,0.)) ;
#21801=DIRECTION('ref_axis',(6.12323399573677E-17,-1.12481983699639E-32,
1.)) ;
#21802=DIRECTION('center_axis',(-0.126432456782393,0.982954607100363,0.133473121834093)) ;
#21803=DIRECTION('ref_axis',(0.675977351380336,0.183848416855219,-0.713620613519996)) ;
#21804=DIRECTION('center_axis',(1.83697019872103E-16,1.,0.)) ;
#21805=DIRECTION('ref_axis',(6.12323399573677E-17,-1.12481983699639E-32,
1.)) ;
#21806=DIRECTION('center_axis',(-0.152169311959628,0.982954607100363,0.1031733535265)) ;
#21807=DIRECTION('ref_axis',(-0.813580713984576,-0.18384841685522,0.55162141134312)) ;
#21808=DIRECTION('center_axis',(1.83697019872103E-16,1.,0.)) ;
#21809=DIRECTION('ref_axis',(6.12323399573677E-17,-1.12481983699639E-32,
1.)) ;
#21810=DIRECTION('center_axis',(-0.170790899233672,0.982954607100363,0.0680493138769549)) ;
#21811=DIRECTION('ref_axis',(-0.913141946632867,-0.18384841685522,0.363829005055077)) ;
#21812=DIRECTION('center_axis',(1.83697019872103E-16,1.,0.)) ;
#21813=DIRECTION('ref_axis',(6.12323399573677E-17,-1.12481983699639E-32,
1.)) ;
#21814=DIRECTION('center_axis',(-0.181426493880004,0.982954607100363,0.0297433639419022)) ;
#21815=DIRECTION('ref_axis',(-0.970005676741035,-0.183848416855222,0.159024358857364)) ;
#21816=DIRECTION('center_axis',(1.83697019872103E-16,1.,0.)) ;
#21817=DIRECTION('ref_axis',(6.12323399573677E-17,-1.12481983699639E-32,
1.)) ;
#21818=DIRECTION('center_axis',(-0.183578787313568,0.982954607100363,-0.00995335263369878)) ;
#21819=DIRECTION('ref_axis',(-0.981513019488615,-0.183848416855221,-0.0532160896174334)) ;
#21820=DIRECTION('center_axis',(1.83697019872103E-16,1.,0.)) ;
#21821=DIRECTION('ref_axis',(6.12323399573677E-17,-1.12481983699639E-32,
1.)) ;
#21822=DIRECTION('center_axis',(1.83697019872103E-16,1.,0.)) ;
#21823=DIRECTION('ref_axis',(6.12323399573677E-17,-1.12481983699639E-32,
1.)) ;
#21824=DIRECTION('center_axis',(-0.16243229064392,0.982954607100363,-0.0861161502642797)) ;
#21825=DIRECTION('ref_axis',(-0.868452234516904,-0.18384841685522,-0.460424234790508)) ;
#21826=DIRECTION('center_axis',(1.83697019872103E-16,1.,0.)) ;
#21827=DIRECTION('ref_axis',(6.12323399573677E-17,-1.12481983699639E-32,
1.)) ;
#21828=DIRECTION('center_axis',(-0.140122287222336,0.982954607100363,-0.119020943550922)) ;
#21829=DIRECTION('ref_axis',(-0.749170703444705,-0.18384841685522,-0.636351331199986)) ;
#21830=DIRECTION('center_axis',(1.83697019872103E-16,1.,0.)) ;
#21831=DIRECTION('ref_axis',(6.12323399573677E-17,-1.12481983699639E-32,
1.)) ;
#21832=DIRECTION('center_axis',(-0.111260321384975,0.982954607100363,-0.146360449799402)) ;
#21833=DIRECTION('ref_axis',(-0.594858782923343,-0.183848416855221,-0.782523346615798)) ;
#21834=DIRECTION('center_axis',(1.83697019872103E-16,1.,0.)) ;
#21835=DIRECTION('ref_axis',(6.12323399573677E-17,-1.12481983699639E-32,
1.)) ;
#21836=DIRECTION('center_axis',(-0.0771959465766158,0.982954607100363,-0.166856304083218)) ;
#21837=DIRECTION('ref_axis',(-0.412731926849916,-0.183848416855221,-0.892105440056603)) ;
#21838=DIRECTION('center_axis',(1.83697019872103E-16,1.,0.)) ;
#21839=DIRECTION('ref_axis',(6.12323399573677E-17,-1.12481983699639E-32,
1.)) ;
#21840=DIRECTION('center_axis',(1.83697019872103E-16,1.,0.)) ;
#21841=DIRECTION('ref_axis',(6.12323399573677E-17,-1.12481983699639E-32,
1.)) ;
#21842=DIRECTION('center_axis',(1.80565831993891E-16,0.982954607100363,
-0.18384841685522)) ;
#21843=DIRECTION('ref_axis',(4.87486550750718E-15,-0.18384841685522,-0.982954607100363)) ;
#21844=DIRECTION('center_axis',(1.83697019872103E-16,1.,0.)) ;
#21845=DIRECTION('ref_axis',(6.12323399573677E-17,-1.12481983699639E-32,
1.)) ;
#21846=DIRECTION('center_axis',(0.039521975103467,0.982954607100363,-0.179550143035566)) ;
#21847=DIRECTION('ref_axis',(0.211306184595842,-0.183848416855221,-0.959973674624141)) ;
#21848=DIRECTION('center_axis',(1.83697019872103E-16,1.,0.)) ;
#21849=DIRECTION('ref_axis',(6.12323399573677E-17,-1.12481983699639E-32,
1.)) ;
#21850=DIRECTION('center_axis',(0.0771959465766158,0.982954607100363,-0.166856304083218)) ;
#21851=DIRECTION('ref_axis',(0.412731926849801,-0.183848416855221,-0.892105440056656)) ;
#21852=DIRECTION('center_axis',(1.83697019872103E-16,1.,0.)) ;
#21853=DIRECTION('ref_axis',(6.12323399573677E-17,-1.12481983699639E-32,
1.)) ;
#21854=DIRECTION('center_axis',(0.111260321384975,0.982954607100363,-0.146360449799403)) ;
#21855=DIRECTION('ref_axis',(0.594858782923056,-0.183848416855222,-0.782523346616016)) ;
#21856=DIRECTION('center_axis',(1.83697019872103E-16,1.,0.)) ;
#21857=DIRECTION('ref_axis',(6.12323399573677E-17,-1.12481983699639E-32,
1.)) ;
#21858=DIRECTION('center_axis',(0.140122287222336,0.982954607100363,-0.119020943550922)) ;
#21859=DIRECTION('ref_axis',(-0.749170703444731,0.18384841685522,0.636351331199956)) ;
#21860=DIRECTION('center_axis',(1.83697019872103E-16,1.,0.)) ;
#21861=DIRECTION('ref_axis',(6.12323399573677E-17,-1.12481983699639E-32,
1.)) ;
#21862=DIRECTION('center_axis',(0.16243229064392,0.982954607100363,-0.0861161502642797)) ;
#21863=DIRECTION('ref_axis',(-0.868452234516886,0.18384841685522,0.460424234790542)) ;
#21864=DIRECTION('center_axis',(1.83697019872103E-16,1.,0.)) ;
#21865=DIRECTION('ref_axis',(6.12323399573677E-17,-1.12481983699639E-32,
1.)) ;
#21866=DIRECTION('center_axis',(0.17714714068552,0.982954607100363,-0.0491846615025046)) ;
#21867=DIRECTION('ref_axis',(-0.947125904318293,0.183848416855222,0.262968212887193)) ;
#21868=DIRECTION('center_axis',(1.83697019872103E-16,1.,0.)) ;
#21869=DIRECTION('ref_axis',(6.12323399573677E-17,-1.12481983699639E-32,
1.)) ;
#21870=DIRECTION('center_axis',(0.183578787313568,0.982954607100363,-0.00995335263369856)) ;
#21871=DIRECTION('ref_axis',(-0.981513019488616,0.183848416855221,0.0532160896174185)) ;
#21872=DIRECTION('center_axis',(1.83697019872103E-16,1.,0.)) ;
#21873=DIRECTION('ref_axis',(6.12323399573677E-17,-1.12481983699639E-32,
1.)) ;
#21874=DIRECTION('center_axis',(0.181426493880004,0.982954607100363,0.0297433639419022)) ;
#21875=DIRECTION('ref_axis',(-0.97000567674103,0.183848416855222,-0.159024358857395)) ;
#21876=DIRECTION('center_axis',(1.83697019872103E-16,1.,0.)) ;
#21877=DIRECTION('ref_axis',(6.12323399573677E-17,-1.12481983699639E-32,
1.)) ;
#21878=DIRECTION('center_axis',(0.170790899233673,0.982954607100363,0.0680493138769549)) ;
#21879=DIRECTION('ref_axis',(-0.913141946632915,0.183848416855221,-0.363829005054957)) ;
#21880=DIRECTION('center_axis',(1.83697019872103E-16,1.,0.)) ;
#21881=DIRECTION('ref_axis',(6.12323399573677E-17,-1.12481983699639E-32,
1.)) ;
#21882=DIRECTION('center_axis',(0.152169311959628,0.982954607100363,0.1031733535265)) ;
#21883=DIRECTION('ref_axis',(-0.813580713984593,0.18384841685522,-0.551621411343096)) ;
#21884=DIRECTION('center_axis',(1.83697019872103E-16,1.,0.)) ;
#21885=DIRECTION('ref_axis',(6.12323399573677E-17,-1.12481983699639E-32,
1.)) ;
#21886=DIRECTION('center_axis',(0.126432456782393,0.982954607100363,0.133473121834093)) ;
#21887=DIRECTION('ref_axis',(-0.675977351380349,0.183848416855219,-0.713620613519984)) ;
#21888=DIRECTION('center_axis',(1.83697019872103E-16,1.,0.)) ;
#21889=DIRECTION('ref_axis',(6.12323399573677E-17,-1.12481983699639E-32,
1.)) ;
#21890=DIRECTION('center_axis',(0.0947837604455976,0.982954607100363,0.157531835309445)) ;
#21891=DIRECTION('ref_axis',(-0.506766039120492,0.18384841685522,-0.842251708940954)) ;
#21892=DIRECTION('center_axis',(1.83697019872103E-16,1.,0.)) ;
#21893=DIRECTION('ref_axis',(6.12323399573677E-17,-1.12481983699639E-32,
1.)) ;
#21894=DIRECTION('center_axis',(0.0587030808149488,0.982954607100363,0.174224535249788)) ;
#21895=DIRECTION('ref_axis',(-0.313858910101348,0.183848416855221,-0.931500050547408)) ;
#21896=DIRECTION('center_axis',(1.83697019872103E-16,1.,0.)) ;
#21897=DIRECTION('ref_axis',(6.12323399573677E-17,-1.12481983699639E-32,
1.)) ;
#21898=DIRECTION('center_axis',(0.0198775103691822,0.982954607100363,0.182770689558513)) ;
#21899=DIRECTION('ref_axis',(-0.10627608727498,0.183848416855221,-0.977192485078221)) ;
#21900=DIRECTION('center_axis',(1.83697019872103E-16,1.,0.)) ;
#21901=DIRECTION('ref_axis',(6.12323399573677E-17,-1.12481983699639E-32,
1.)) ;
#21902=DIRECTION('center_axis',(-0.17714714068552,0.982954607100363,-0.0491846615025055)) ;
#21903=DIRECTION('ref_axis',(-0.947125904318291,-0.183848416855222,-0.262968212887199)) ;
#21904=DIRECTION('center_axis',(-0.0395219751034661,0.982954607100363,-0.179550143035566)) ;
#21905=DIRECTION('ref_axis',(-0.211306184595852,-0.183848416855221,-0.959973674624139)) ;
#21906=DIRECTION('center_axis',(1.83697019872103E-16,1.,0.)) ;
#21907=DIRECTION('ref_axis',(6.12323399573677E-17,-1.12481983699639E-32,
1.)) ;
#21908=DIRECTION('',(0.0894326665084245,-0.995991732165632,0.00150586151291223)) ;
#21909=DIRECTION('center_axis',(-0.0198775103691822,0.982954607100363,0.182770689558513)) ;
#21910=DIRECTION('ref_axis',(-0.106276087274983,-0.183848416855221,0.977192485078221)) ;
#21911=DIRECTION('center_axis',(-0.0198775103691822,0.982954607100363,0.182770689558513)) ;
#21912=DIRECTION('ref_axis',(-0.106276087274983,-0.183848416855221,0.977192485078221)) ;
#21913=DIRECTION('',(0.0876654961771864,0.9959917321656,0.0177547243790319)) ;
#21914=DIRECTION('',(0.0870195460927401,-0.995991472747943,0.0207022899988359)) ;
#21915=DIRECTION('center_axis',(-0.0587030808149488,0.982954607100363,0.174224535249788)) ;
#21916=DIRECTION('ref_axis',(-0.313858910101354,-0.183848416855221,0.931500050547405)) ;
#21917=DIRECTION('center_axis',(-0.0587030808149488,0.982954607100363,0.174224535249788)) ;
#21918=DIRECTION('ref_axis',(-0.313858910101354,-0.183848416855221,0.931500050547405)) ;
#21919=DIRECTION('',(0.0818041493280548,0.995991472747942,0.0361810360009097)) ;
#21920=DIRECTION('',(0.0805345699739786,-0.995991874626499,0.0389148906859529)) ;
#21921=DIRECTION('center_axis',(-0.0947837604455976,0.982954607100363,0.157531835309445)) ;
#21922=DIRECTION('ref_axis',(-0.506766039120519,-0.183848416855219,0.842251708940938)) ;
#21923=DIRECTION('center_axis',(-0.0947837604455976,0.982954607100363,0.157531835309445)) ;
#21924=DIRECTION('ref_axis',(-0.506766039120519,-0.183848416855219,0.842251708940938)) ;
#21925=DIRECTION('',(0.0721048469731237,0.995991874626519,0.0529251992999018)) ;
#21926=DIRECTION('',(0.070286008728264,-0.995991843748342,0.055318389020542)) ;
#21927=DIRECTION('center_axis',(-0.126432456782393,0.982954607100363,0.133473121834093)) ;
#21928=DIRECTION('ref_axis',(-0.675977351380399,-0.183848416855219,0.713620613519936)) ;
#21929=DIRECTION('center_axis',(-0.126432456782393,0.982954607100363,0.133473121834093)) ;
#21930=DIRECTION('ref_axis',(-0.675977351380399,-0.183848416855219,0.713620613519936)) ;
#21931=DIRECTION('',(0.0590424676389299,0.995991843748325,0.0671880510352708)) ;
#21932=DIRECTION('',(0.0567510610610272,-0.995991855108921,0.0691342290413218)) ;
#21933=DIRECTION('center_axis',(-0.152169311959628,0.982954607100363,0.1031733535265)) ;
#21934=DIRECTION('ref_axis',(-0.813580713984602,-0.18384841685522,0.551621411343083)) ;
#21935=DIRECTION('center_axis',(-0.152169311959628,0.982954607100363,0.1031733535265)) ;
#21936=DIRECTION('ref_axis',(-0.813580713984602,-0.18384841685522,0.551621411343083)) ;
#21937=DIRECTION('',(0.0432183562672333,0.995991855108916,0.0783096305588247)) ;
#21938=DIRECTION('',(0.0405615702551079,-0.995991800293961,0.0797188357017008)) ;
#21939=DIRECTION('center_axis',(-0.170790899233673,0.982954607100363,0.0680493138769549)) ;
#21940=DIRECTION('ref_axis',(-0.913141946632898,-0.183848416855221,0.363829005054999)) ;
#21941=DIRECTION('center_axis',(-0.170790899233673,0.982954607100363,0.0680493138769549)) ;
#21942=DIRECTION('ref_axis',(-0.913141946632898,-0.183848416855221,0.363829005054999)) ;
#21943=DIRECTION('',(0.0253750830217403,0.99599180029395,0.0857696852556677)) ;
#21944=DIRECTION('',(0.0224747998305547,-0.995991732165588,0.0865757057745833)) ;
#21945=DIRECTION('center_axis',(-0.181426493880003,0.982954607100363,0.0297433639419022)) ;
#21946=DIRECTION('ref_axis',(-0.970005676741024,-0.183848416855221,0.159024358857432)) ;
#21947=DIRECTION('center_axis',(-0.181426493880003,0.982954607100363,0.0297433639419022)) ;
#21948=DIRECTION('ref_axis',(-0.970005676741024,-0.183848416855221,0.159024358857432)) ;
#21949=DIRECTION('',(0.00634543999453282,0.995991732165633,0.0892199800996225)) ;
#21950=DIRECTION('',(0.00333813391881096,-0.995991732165608,0.0893830314975548)) ;
#21951=DIRECTION('center_axis',(-0.183578787313568,0.982954607100363,-0.00995335263369877)) ;
#21952=DIRECTION('ref_axis',(0.981513019488616,0.183848416855221,0.0532160896174231)) ;
#21953=DIRECTION('center_axis',(-0.183578787313568,0.982954607100363,-0.00995335263369877)) ;
#21954=DIRECTION('ref_axis',(0.981513019488616,0.183848416855221,0.0532160896174231)) ;
#21955=DIRECTION('',(-0.0129825712619722,0.995991732165591,0.0884981485750611)) ;
#21956=DIRECTION('',(-0.0159729881663253,-0.995990956174831,0.0880163556788385)) ;
#21957=DIRECTION('center_axis',(-0.17714714068552,0.982954607100363,-0.0491846615025055)) ;
#21958=DIRECTION('ref_axis',(0.947125904318289,0.183848416855222,0.262968212887207)) ;
#21959=DIRECTION('center_axis',(-0.17714714068552,0.982954607100363,-0.0491846615025055)) ;
#21960=DIRECTION('ref_axis',(0.947125904318289,0.183848416855222,0.262968212887207)) ;
#21961=DIRECTION('',(-0.0316906021296052,0.995990956174818,0.0836523816435276)) ;
#21962=DIRECTION('',(-0.0344972257280317,-0.995991897161699,0.0825232222184031)) ;
#21963=DIRECTION('center_axis',(-0.16243229064392,0.982954607100363,-0.0861161502642797)) ;
#21964=DIRECTION('ref_axis',(0.868452234516877,0.18384841685522,0.460424234790559)) ;
#21965=DIRECTION('center_axis',(-0.16243229064392,0.982954607100363,-0.0861161502642797)) ;
#21966=DIRECTION('ref_axis',(0.868452234516877,0.18384841685522,0.460424234790559)) ;
#21967=DIRECTION('',(-0.0489441662534316,0.995991897161676,0.0748639391031554)) ;
#21968=DIRECTION('',(-0.0514320044770238,-0.995991845655882,0.0731778129111852)) ;
#21969=DIRECTION('center_axis',(-0.140122287222336,0.982954607100363,-0.119020943550922)) ;
#21970=DIRECTION('ref_axis',(0.749170703444789,0.18384841685522,0.636351331199888)) ;
#21971=DIRECTION('center_axis',(-0.140122287222336,0.982954607100363,-0.119020943550922)) ;
#21972=DIRECTION('ref_axis',(0.749170703444789,0.18384841685522,0.636351331199888)) ;
#21973=DIRECTION('',(-0.0638930342713704,0.995991845655898,0.06259331880126)) ;
#21974=DIRECTION('',(-0.0659605301635769,-0.995991849453985,0.0604106305361067)) ;
#21975=DIRECTION('center_axis',(-0.111260321384975,0.982954607100363,-0.146360449799403)) ;
#21976=DIRECTION('ref_axis',(0.594858782923059,0.183848416855222,0.782523346616013)) ;
#21977=DIRECTION('center_axis',(-0.111260321384975,0.982954607100363,-0.146360449799403)) ;
#21978=DIRECTION('ref_axis',(0.594858782923059,0.183848416855222,0.782523346616013)) ;
#21979=DIRECTION('',(-0.0758549736440145,0.995991849454008,0.0473947127288519)) ;
#21980=DIRECTION('',(-0.0774044203990348,-0.995991874113701,0.044818995996865)) ;
#21981=DIRECTION('center_axis',(-0.0771959465766158,0.982954607100363,-0.166856304083218)) ;
#21982=DIRECTION('ref_axis',(0.412731926849895,0.183848416855221,0.892105440056612)) ;
#21983=DIRECTION('center_axis',(-0.0771959465766158,0.982954607100363,-0.166856304083218)) ;
#21984=DIRECTION('ref_axis',(0.412731926849895,0.183848416855221,0.892105440056612)) ;
#21985=DIRECTION('',(-0.0842698982455389,0.995991874113698,0.0299795088213562)) ;
#21986=DIRECTION('',(-0.085251590350561,-0.995990596094747,0.0271090175685372)) ;
#21987=DIRECTION('center_axis',(-0.0395219751034661,0.982954607100363,-0.179550143035566)) ;
#21988=DIRECTION('ref_axis',(0.211306184595816,0.183848416855221,0.959973674624147)) ;
#21989=DIRECTION('center_axis',(-0.0395219751034661,0.982954607100363,-0.179550143035566)) ;
#21990=DIRECTION('ref_axis',(0.211306184595816,0.183848416855221,0.959973674624147)) ;
#21991=DIRECTION('',(-0.0887550289210553,0.995990596094745,0.0111927356824723)) ;
#21992=DIRECTION('',(-0.0890712206546686,-0.995991732165598,0.00817233802896422)) ;
#21993=DIRECTION('center_axis',(1.80565831993891E-16,0.982954607100363,
-0.18384841685522)) ;
#21994=DIRECTION('ref_axis',(9.39610169491382E-17,0.18384841685522,0.982954607100363)) ;
#21995=DIRECTION('center_axis',(1.80565831993891E-16,0.982954607100363,
-0.18384841685522)) ;
#21996=DIRECTION('ref_axis',(9.39610169491382E-17,0.18384841685522,0.982954607100363)) ;
#21997=DIRECTION('',(-0.0890712206546686,0.995991732165598,-0.00817233802896422)) ;
#21998=DIRECTION('',(-0.0887550289209964,-0.995990596094752,-0.0111927356822663)) ;
#21999=DIRECTION('center_axis',(0.039521975103467,0.982954607100363,-0.179550143035566)) ;
#22000=DIRECTION('ref_axis',(-0.211306184595819,0.183848416855221,0.959973674624146)) ;
#22001=DIRECTION('center_axis',(0.039521975103467,0.982954607100363,-0.179550143035566)) ;
#22002=DIRECTION('ref_axis',(-0.211306184595819,0.183848416855221,0.959973674624146)) ;
#22003=DIRECTION('',(-0.0852515903504576,0.995990596094755,-0.0271090175685374)) ;
#22004=DIRECTION('',(-0.0842698982454947,-0.995991874113696,-0.0299795088215489)) ;
#22005=DIRECTION('center_axis',(0.0771959465766158,0.982954607100363,-0.166856304083218)) ;
#22006=DIRECTION('ref_axis',(-0.412731926849894,0.183848416855221,0.892105440056613)) ;
#22007=DIRECTION('center_axis',(0.0771959465766158,0.982954607100363,-0.166856304083218)) ;
#22008=DIRECTION('ref_axis',(-0.412731926849894,0.183848416855221,0.892105440056613)) ;
#22009=DIRECTION('',(-0.0774044203992267,0.995991874113696,-0.0448189959966469)) ;
#22010=DIRECTION('',(-0.0758549736442256,-0.995991849454001,-0.0473947127286581)) ;
#22011=DIRECTION('center_axis',(0.111260321384975,0.982954607100363,-0.146360449799403)) ;
#22012=DIRECTION('ref_axis',(-0.594858782923059,0.183848416855222,0.782523346616014)) ;
#22013=DIRECTION('center_axis',(0.111260321384975,0.982954607100363,-0.146360449799403)) ;
#22014=DIRECTION('ref_axis',(-0.594858782923059,0.183848416855222,0.782523346616014)) ;
#22015=DIRECTION('',(-0.0659605301634746,0.995991849453984,-0.060410630536239)) ;
#22016=DIRECTION('',(-0.0638930342712978,-0.995991845655893,-0.0625933188014015)) ;
#22017=DIRECTION('center_axis',(0.140122287222336,0.982954607100363,-0.119020943550922)) ;
#22018=DIRECTION('ref_axis',(-0.74917070344479,0.18384841685522,0.636351331199887)) ;
#22019=DIRECTION('center_axis',(0.140122287222336,0.982954607100363,-0.119020943550922)) ;
#22020=DIRECTION('ref_axis',(-0.74917070344479,0.18384841685522,0.636351331199887)) ;
#22021=DIRECTION('',(-0.0514320044769895,0.995991845655871,-0.073177812911361)) ;
#22022=DIRECTION('',(-0.0489441662532377,-0.995991897161693,-0.0748639391030673)) ;
#22023=DIRECTION('center_axis',(0.16243229064392,0.982954607100363,-0.0861161502642797)) ;
#22024=DIRECTION('ref_axis',(-0.868452234516877,0.18384841685522,0.460424234790559)) ;
#22025=DIRECTION('center_axis',(0.16243229064392,0.982954607100363,-0.0861161502642797)) ;
#22026=DIRECTION('ref_axis',(-0.868452234516877,0.18384841685522,0.460424234790559)) ;
#22027=DIRECTION('',(-0.0344972257278522,0.9959918971617,-0.0825232222184722)) ;
#22028=DIRECTION('',(-0.0316906021296349,-0.995990956174831,-0.0836523816433686)) ;
#22029=DIRECTION('center_axis',(0.17714714068552,0.982954607100363,-0.0491846615025046)) ;
#22030=DIRECTION('ref_axis',(-0.947125904318291,0.183848416855222,0.262968212887201)) ;
#22031=DIRECTION('center_axis',(0.17714714068552,0.982954607100363,-0.0491846615025046)) ;
#22032=DIRECTION('ref_axis',(-0.947125904318291,0.183848416855222,0.262968212887201)) ;
#22033=DIRECTION('',(-0.0159729881664467,0.995990956174826,-0.0880163556788801)) ;
#22034=DIRECTION('',(-0.0129825712619121,-0.99599173216567,-0.0884981485741822)) ;
#22035=DIRECTION('center_axis',(0.183578787313568,0.982954607100363,-0.00995335263369855)) ;
#22036=DIRECTION('ref_axis',(-0.981513019488616,0.183848416855221,0.0532160896174219)) ;
#22037=DIRECTION('center_axis',(0.183578787313568,0.982954607100363,-0.00995335263369855)) ;
#22038=DIRECTION('ref_axis',(-0.981513019488616,0.183848416855221,0.0532160896174219)) ;
#22039=DIRECTION('',(0.00333813391881109,0.995991732165649,-0.0893830314970895)) ;
#22040=DIRECTION('',(0.00634543999453281,-0.995991732165632,-0.0892199800996354)) ;
#22041=DIRECTION('center_axis',(0.181426493880003,0.982954607100363,0.0297433639419022)) ;
#22042=DIRECTION('ref_axis',(0.970005676741024,-0.183848416855221,0.159024358857432)) ;
#22043=DIRECTION('center_axis',(0.181426493880003,0.982954607100363,0.0297433639419022)) ;
#22044=DIRECTION('ref_axis',(0.970005676741024,-0.183848416855221,0.159024358857432)) ;
#22045=DIRECTION('',(0.0224747998304496,0.995991732165622,-0.0865757057742305)) ;
#22046=DIRECTION('',(0.0253750830216289,-0.995991800293954,-0.0857696852556559)) ;
#22047=DIRECTION('center_axis',(0.170790899233672,0.982954607100363,0.0680493138769549)) ;
#22048=DIRECTION('ref_axis',(0.913141946632898,-0.18384841685522,0.363829005054999)) ;
#22049=DIRECTION('center_axis',(0.170790899233672,0.982954607100363,0.0680493138769549)) ;
#22050=DIRECTION('ref_axis',(0.913141946632898,-0.18384841685522,0.363829005054999)) ;
#22051=DIRECTION('',(0.0405615702551252,0.995991800293957,-0.0797188357017419)) ;
#22052=DIRECTION('',(0.0432183562674327,-0.995991855108905,-0.0783096305588474)) ;
#22053=DIRECTION('center_axis',(0.152169311959628,0.982954607100363,0.1031733535265)) ;
#22054=DIRECTION('ref_axis',(0.813580713984602,-0.18384841685522,0.551621411343082)) ;
#22055=DIRECTION('center_axis',(0.152169311959628,0.982954607100363,0.1031733535265)) ;
#22056=DIRECTION('ref_axis',(0.813580713984602,-0.18384841685522,0.551621411343082)) ;
#22057=DIRECTION('',(0.0567510610609564,0.99599185510892,-0.0691342290413986)) ;
#22058=DIRECTION('',(0.0590424676390377,-0.995991843748321,-0.0671880510352316)) ;
#22059=DIRECTION('center_axis',(0.126432456782393,0.982954607100363,0.133473121834093)) ;
#22060=DIRECTION('ref_axis',(0.675977351380399,-0.183848416855219,0.713620613519936)) ;
#22061=DIRECTION('center_axis',(0.126432456782393,0.982954607100363,0.133473121834093)) ;
#22062=DIRECTION('ref_axis',(0.675977351380399,-0.183848416855219,0.713620613519936)) ;
#22063=DIRECTION('',(0.0702860087283124,0.995991843748332,-0.0553183890206689)) ;
#22064=DIRECTION('',(0.0721048469732812,-0.9959918746265,-0.0529251993000518)) ;
#22065=DIRECTION('center_axis',(0.0947837604455977,0.982954607100363,0.157531835309445)) ;
#22066=DIRECTION('ref_axis',(0.506766039120516,-0.18384841685522,0.842251708940939)) ;
#22067=DIRECTION('center_axis',(0.0947837604455977,0.982954607100363,0.157531835309445)) ;
#22068=DIRECTION('ref_axis',(0.506766039120516,-0.18384841685522,0.842251708940939)) ;
#22069=DIRECTION('',(0.0805345699739992,0.995991874626496,-0.0389148906859699)) ;
#22070=DIRECTION('',(0.0818041493280427,-0.995991472747948,-0.036181036000766)) ;
#22071=DIRECTION('center_axis',(0.0587030808149488,0.982954607100363,0.174224535249788)) ;
#22072=DIRECTION('ref_axis',(0.313858910101352,-0.183848416855221,0.931500050547406)) ;
#22073=DIRECTION('center_axis',(0.0587030808149488,0.982954607100363,0.174224535249788)) ;
#22074=DIRECTION('ref_axis',(0.313858910101352,-0.183848416855221,0.931500050547406)) ;
#22075=DIRECTION('',(0.087019546092724,0.99599147274794,-0.0207022899990529)) ;
#22076=DIRECTION('',(0.0876654961766692,-0.995991732165646,-0.0177547243790327)) ;
#22077=DIRECTION('center_axis',(0.0198775103691822,0.982954607100363,0.182770689558513)) ;
#22078=DIRECTION('ref_axis',(0.106276087274981,-0.183848416855221,0.977192485078221)) ;
#22079=DIRECTION('center_axis',(0.0198775103691822,0.982954607100363,0.182770689558513)) ;
#22080=DIRECTION('ref_axis',(0.106276087274981,-0.183848416855221,0.977192485078221)) ;
#22081=DIRECTION('',(0.089432666508431,0.995991732165632,-0.00150586151291223)) ;
#22082=DIRECTION('',(-1.83697019872103E-16,-1.,0.)) ;
#22083=DIRECTION('center_axis',(1.83697019872103E-16,1.,0.)) ;
#22084=DIRECTION('ref_axis',(6.12323399573677E-17,-1.12481983699639E-32,
1.)) ;
#22085=DIRECTION('center_axis',(-1.83697019872103E-16,-1.,0.)) ;
#22086=DIRECTION('ref_axis',(6.12323399573676E-17,-1.12481983699639E-32,
1.)) ;
#22087=DIRECTION('center_axis',(1.83697019872103E-16,1.,0.)) ;
#22088=DIRECTION('ref_axis',(6.12323399573676E-17,-1.12481983699639E-32,
1.)) ;
#22089=DIRECTION('',(-1.67503306565163E-16,-0.979306480331619,-0.202382849027518)) ;
#22090=DIRECTION('center_axis',(1.83697019872103E-16,1.,0.)) ;
#22091=DIRECTION('ref_axis',(6.12323399573676E-17,-1.12481983699639E-32,
1.)) ;
#22092=DIRECTION('center_axis',(-1.80565831993891E-16,-0.982954607100363,
0.18384841685522)) ;
#22093=DIRECTION('ref_axis',(3.97603040674231E-15,-0.18384841685522,-0.982954607100363)) ;
#22094=DIRECTION('center_axis',(0.0771959465766158,-0.982954607100363,0.166856304083218)) ;
#22095=DIRECTION('ref_axis',(-0.412731926849851,-0.183848416855221,-0.892105440056633)) ;
#22096=DIRECTION('center_axis',(0.140122287222336,-0.982954607100363,0.119020943550922)) ;
#22097=DIRECTION('ref_axis',(-0.749170703444893,-0.18384841685522,-0.636351331199766)) ;
#22098=DIRECTION('center_axis',(0.17714714068552,-0.982954607100363,0.0491846615025055)) ;
#22099=DIRECTION('ref_axis',(-0.947125904318309,-0.183848416855222,-0.262968212887135)) ;
#22100=DIRECTION('center_axis',(0.181426493880003,-0.982954607100363,-0.0297433639419022)) ;
#22101=DIRECTION('ref_axis',(-0.970005676741017,-0.183848416855221,0.159024358857473)) ;
#22102=DIRECTION('center_axis',(0.152169311959628,-0.982954607100363,-0.1031733535265)) ;
#22103=DIRECTION('ref_axis',(-0.813580713984591,-0.18384841685522,0.551621411343099)) ;
#22104=DIRECTION('center_axis',(0.0947837604455976,-0.982954607100363,-0.157531835309445)) ;
#22105=DIRECTION('ref_axis',(0.506766039120523,0.183848416855219,-0.842251708940935)) ;
#22106=DIRECTION('center_axis',(0.0198775103691822,-0.982954607100363,-0.182770689558513)) ;
#22107=DIRECTION('ref_axis',(0.106276087274989,0.183848416855221,-0.97719248507822)) ;
#22108=DIRECTION('center_axis',(0.0587030808149489,-0.982954607100363,-0.174224535249788)) ;
#22109=DIRECTION('ref_axis',(0.31385891010127,0.183848416855221,-0.931500050547434)) ;
#22110=DIRECTION('center_axis',(0.126432456782393,-0.982954607100363,-0.133473121834093)) ;
#22111=DIRECTION('ref_axis',(-0.675977351380272,-0.183848416855219,0.713620613520057)) ;
#22112=DIRECTION('center_axis',(0.170790899233672,-0.982954607100363,-0.0680493138769549)) ;
#22113=DIRECTION('ref_axis',(-0.913141946632923,-0.18384841685522,0.363829005054938)) ;
#22114=DIRECTION('center_axis',(0.183578787313568,-0.982954607100363,0.00995335263369878)) ;
#22115=DIRECTION('ref_axis',(-0.981513019488616,-0.183848416855221,-0.0532160896174178)) ;
#22116=DIRECTION('center_axis',(0.16243229064392,-0.982954607100363,0.0861161502642797)) ;
#22117=DIRECTION('ref_axis',(-0.868452234516837,-0.183848416855221,-0.460424234790635)) ;
#22118=DIRECTION('center_axis',(0.111260321384975,-0.982954607100363,0.146360449799402)) ;
#22119=DIRECTION('ref_axis',(-0.594858782922928,-0.183848416855221,-0.782523346616113)) ;
#22120=DIRECTION('center_axis',(0.0395219751034661,-0.982954607100363,0.179550143035566)) ;
#22121=DIRECTION('ref_axis',(-0.211306184595861,-0.183848416855221,-0.959973674624137)) ;
#22122=DIRECTION('center_axis',(-0.0771959465766158,-0.982954607100363,
0.166856304083218)) ;
#22123=DIRECTION('ref_axis',(0.412731926849952,-0.183848416855221,-0.892105440056586)) ;
#22124=DIRECTION('center_axis',(-0.140122287222336,-0.982954607100363,0.119020943550922)) ;
#22125=DIRECTION('ref_axis',(-0.749170703444845,0.18384841685522,0.636351331199822)) ;
#22126=DIRECTION('center_axis',(-0.17714714068552,-0.982954607100363,0.0491846615025046)) ;
#22127=DIRECTION('ref_axis',(-0.947125904318295,0.183848416855222,0.262968212887186)) ;
#22128=DIRECTION('center_axis',(-0.181426493880003,-0.982954607100363,-0.0297433639419022)) ;
#22129=DIRECTION('ref_axis',(-0.97000567674102,0.183848416855221,-0.159024358857453)) ;
#22130=DIRECTION('center_axis',(-0.152169311959628,-0.982954607100363,-0.1031733535265)) ;
#22131=DIRECTION('ref_axis',(-0.813580713984562,0.18384841685522,-0.551621411343141)) ;
#22132=DIRECTION('center_axis',(-0.0947837604455976,-0.982954607100363,
-0.157531835309445)) ;
#22133=DIRECTION('ref_axis',(-0.506766039120481,0.183848416855219,-0.842251708940961)) ;
#22134=DIRECTION('center_axis',(-0.0198775103691822,-0.982954607100363,
-0.182770689558513)) ;
#22135=DIRECTION('ref_axis',(-0.106276087274979,0.183848416855221,-0.977192485078221)) ;
#22136=DIRECTION('center_axis',(-0.0587030808149489,-0.982954607100363,
-0.174224535249788)) ;
#22137=DIRECTION('ref_axis',(-0.313858910101256,0.183848416855221,-0.931500050547439)) ;
#22138=DIRECTION('center_axis',(-0.126432456782393,-0.982954607100363,-0.133473121834093)) ;
#22139=DIRECTION('ref_axis',(-0.675977351380318,0.183848416855219,-0.713620613520013)) ;
#22140=DIRECTION('center_axis',(-0.170790899233673,-0.982954607100363,-0.0680493138769549)) ;
#22141=DIRECTION('ref_axis',(-0.913141946632883,0.183848416855221,-0.363829005055038)) ;
#22142=DIRECTION('center_axis',(-0.183578787313568,-0.982954607100363,0.00995335263369855)) ;
#22143=DIRECTION('ref_axis',(-0.981513019488616,0.183848416855221,0.0532160896174153)) ;
#22144=DIRECTION('center_axis',(-0.16243229064392,-0.982954607100363,0.0861161502642797)) ;
#22145=DIRECTION('ref_axis',(-0.868452234516967,0.18384841685522,0.460424234790391)) ;
#22146=DIRECTION('center_axis',(-0.111260321384975,-0.982954607100363,0.146360449799403)) ;
#22147=DIRECTION('ref_axis',(0.594858782923022,-0.183848416855222,-0.782523346616042)) ;
#22148=DIRECTION('center_axis',(-0.039521975103467,-0.982954607100363,0.179550143035566)) ;
#22149=DIRECTION('ref_axis',(0.211306184595843,-0.183848416855221,-0.959973674624141)) ;
#22150=DIRECTION('center_axis',(1.83697019872103E-16,1.,1.91045767932109E-48)) ;
#22151=DIRECTION('ref_axis',(6.12323399573677E-17,-1.12481983699639E-32,
1.)) ;
#22152=DIRECTION('center_axis',(1.83697019872103E-16,1.,1.91045767932109E-48)) ;
#22153=DIRECTION('ref_axis',(6.12323399573677E-17,-1.12481983699639E-32,
1.)) ;
#22154=DIRECTION('',(-1.83697019872103E-16,-1.,-1.91045767932109E-48)) ;
#22155=DIRECTION('center_axis',(1.83697019872103E-16,1.,1.91045767932109E-48)) ;
#22156=DIRECTION('ref_axis',(6.12323399573677E-17,-1.12481983699639E-32,
1.)) ;
#22157=DIRECTION('center_axis',(1.83697019872103E-16,1.,0.)) ;
#22158=DIRECTION('ref_axis',(0.,0.,1.)) ;
#22159=DIRECTION('center_axis',(1.83697019872103E-16,1.,0.)) ;
#22160=DIRECTION('ref_axis',(6.12323399573677E-17,-1.12481983699639E-32,
1.)) ;
#22161=DIRECTION('center_axis',(-1.,1.83697019872103E-16,1.22464679914735E-16)) ;
#22162=DIRECTION('ref_axis',(-1.22464679914735E-16,0.,-1.)) ;
#22163=DIRECTION('center_axis',(1.83697019872103E-16,1.,0.)) ;
#22164=DIRECTION('ref_axis',(6.12323399573677E-17,-1.12481983699639E-32,
1.)) ;
#22165=DIRECTION('center_axis',(1.83697019872103E-16,1.,0.)) ;
#22166=DIRECTION('ref_axis',(0.,0.,1.)) ;
#22167=DIRECTION('center_axis',(1.83697019872103E-16,1.,2.10365691773288E-48)) ;
#22168=DIRECTION('ref_axis',(6.12323399573676E-17,-1.12481983699639E-32,
1.)) ;
#22169=DIRECTION('center_axis',(-1.,1.83697019872103E-16,1.22464679914735E-16)) ;
#22170=DIRECTION('ref_axis',(-1.22464679914735E-16,0.,-1.)) ;
#22171=DIRECTION('center_axis',(1.83697019872103E-16,1.,-1.99295781592863E-48)) ;
#22172=DIRECTION('ref_axis',(6.12323399573676E-17,-1.12481983699639E-32,
1.)) ;
#22173=DIRECTION('center_axis',(1.83697019872103E-16,1.,0.)) ;
#22174=DIRECTION('ref_axis',(0.,0.,1.)) ;
#22175=DIRECTION('center_axis',(1.83697019872103E-16,1.,-1.99295781592863E-48)) ;
#22176=DIRECTION('ref_axis',(6.12323399573676E-17,-1.12481983699639E-32,
1.)) ;
#22177=DIRECTION('center_axis',(-1.,1.83697019872103E-16,1.22464679914735E-16)) ;
#22178=DIRECTION('ref_axis',(-1.22464679914735E-16,0.,-1.)) ;
#22179=DIRECTION('center_axis',(1.83697019872103E-16,1.,-2.01979869638278E-48)) ;
#22180=DIRECTION('ref_axis',(6.12323399573676E-17,-1.12481983699639E-32,
1.)) ;
#22181=DIRECTION('center_axis',(1.83697019872103E-16,1.,0.)) ;
#22182=DIRECTION('ref_axis',(6.12323399573677E-17,-1.12481983699639E-32,
1.)) ;
#22183=DIRECTION('',(1.83697019872103E-16,1.,0.)) ;
#22184=DIRECTION('center_axis',(1.83697019872103E-16,1.,0.)) ;
#22185=DIRECTION('ref_axis',(6.12323399573677E-17,-1.12481983699639E-32,
1.)) ;
#22186=DIRECTION('center_axis',(1.83697019872103E-16,1.,0.)) ;
#22187=DIRECTION('ref_axis',(0.,0.,1.)) ;
#22188=DIRECTION('center_axis',(-1.,1.83697019872103E-16,1.22464679914735E-16)) ;
#22189=DIRECTION('ref_axis',(-1.22464679914735E-16,0.,-1.)) ;
#22190=DIRECTION('center_axis',(1.83697019872103E-16,1.,0.)) ;
#22191=DIRECTION('ref_axis',(6.12323399573677E-17,-1.12481983699639E-32,
1.)) ;
#22192=DIRECTION('center_axis',(1.83697019872103E-16,1.,-1.99295781592863E-48)) ;
#22193=DIRECTION('ref_axis',(6.12323399573676E-17,-1.12481983699639E-32,
1.)) ;
#22194=DIRECTION('',(-1.83697019872103E-16,-1.,1.99295781592863E-48)) ;
#22195=DIRECTION('center_axis',(1.83697019872103E-16,1.,1.83697019872103E-16)) ;
#22196=DIRECTION('ref_axis',(6.12323399573676E-17,-1.83697019872103E-16,
1.)) ;
#22197=DIRECTION('center_axis',(-1.83697019872103E-16,-1.,-5.58347057653491E-16)) ;
#22198=DIRECTION('ref_axis',(-6.12323399573676E-17,5.58347057653491E-16,
-1.)) ;
#22199=DIRECTION('center_axis',(1.83697019872103E-16,1.,6.12323399573677E-17)) ;
#22200=DIRECTION('ref_axis',(6.12323399573676E-17,-6.12323399573677E-17,
1.)) ;
#22201=DIRECTION('center_axis',(1.80565831993891E-16,0.982954607100363,
-0.18384841685522)) ;
#22202=DIRECTION('ref_axis',(6.12323399573677E-17,0.18384841685522,0.982954607100363)) ;
#22203=DIRECTION('center_axis',(1.80565831993891E-16,0.982954607100363,
-0.18384841685522)) ;
#22204=DIRECTION('ref_axis',(6.12323399573677E-17,0.18384841685522,0.982954607100363)) ;
#22205=DIRECTION('center_axis',(1.80565831993891E-16,0.982954607100363,
-0.18384841685522)) ;
#22206=DIRECTION('ref_axis',(6.12323399573677E-17,0.18384841685522,0.982954607100363)) ;
#22207=DIRECTION('center_axis',(0.039521975103467,0.982954607100363,-0.179550143035566)) ;
#22208=DIRECTION('ref_axis',(-0.211306184595818,0.183848416855221,0.959973674624147)) ;
#22209=DIRECTION('center_axis',(0.039521975103467,0.982954607100363,-0.179550143035567)) ;
#22210=DIRECTION('ref_axis',(-0.211306184595818,0.183848416855222,0.959973674624146)) ;
#22211=DIRECTION('center_axis',(0.039521975103467,0.982954607100363,-0.179550143035567)) ;
#22212=DIRECTION('ref_axis',(-0.211306184595818,0.183848416855222,0.959973674624146)) ;
#22213=DIRECTION('center_axis',(0.0771959465766159,0.982954607100363,-0.166856304083218)) ;
#22214=DIRECTION('ref_axis',(-0.412731926849895,0.183848416855221,0.892105440056612)) ;
#22215=DIRECTION('center_axis',(0.0771959465766159,0.982954607100363,-0.166856304083218)) ;
#22216=DIRECTION('ref_axis',(-0.412731926849895,0.183848416855221,0.892105440056612)) ;
#22217=DIRECTION('center_axis',(0.0771959465766159,0.982954607100363,-0.166856304083218)) ;
#22218=DIRECTION('ref_axis',(-0.412731926849895,0.183848416855221,0.892105440056612)) ;
#22219=DIRECTION('center_axis',(0.111260321384975,0.982954607100363,-0.146360449799403)) ;
#22220=DIRECTION('ref_axis',(-0.594858782923058,0.183848416855222,0.782523346616014)) ;
#22221=DIRECTION('center_axis',(0.111260321384975,0.982954607100363,-0.146360449799403)) ;
#22222=DIRECTION('ref_axis',(-0.594858782923058,0.183848416855222,0.782523346616014)) ;
#22223=DIRECTION('center_axis',(0.111260321384975,0.982954607100363,-0.146360449799403)) ;
#22224=DIRECTION('ref_axis',(-0.594858782923058,0.183848416855222,0.782523346616014)) ;
#22225=DIRECTION('center_axis',(0.140122287222337,0.982954607100363,-0.119020943550922)) ;
#22226=DIRECTION('ref_axis',(-0.749170703444791,0.18384841685522,0.636351331199885)) ;
#22227=DIRECTION('center_axis',(0.140122287222337,0.982954607100363,-0.119020943550922)) ;
#22228=DIRECTION('ref_axis',(-0.749170703444791,0.18384841685522,0.636351331199885)) ;
#22229=DIRECTION('center_axis',(0.140122287222337,0.982954607100363,-0.119020943550922)) ;
#22230=DIRECTION('ref_axis',(-0.749170703444791,0.18384841685522,0.636351331199885)) ;
#22231=DIRECTION('center_axis',(0.162432290643921,0.982954607100363,-0.0861161502642798)) ;
#22232=DIRECTION('ref_axis',(-0.868452234516879,0.183848416855221,0.460424234790555)) ;
#22233=DIRECTION('center_axis',(0.162432290643921,0.982954607100363,-0.0861161502642798)) ;
#22234=DIRECTION('ref_axis',(-0.868452234516879,0.183848416855221,0.460424234790555)) ;
#22235=DIRECTION('center_axis',(0.162432290643921,0.982954607100363,-0.0861161502642798)) ;
#22236=DIRECTION('ref_axis',(-0.868452234516879,0.183848416855221,0.460424234790555)) ;
#22237=DIRECTION('center_axis',(0.17714714068552,0.982954607100363,-0.0491846615025047)) ;
#22238=DIRECTION('ref_axis',(-0.94712590431829,0.183848416855222,0.262968212887203)) ;
#22239=DIRECTION('center_axis',(0.17714714068552,0.982954607100363,-0.0491846615025047)) ;
#22240=DIRECTION('ref_axis',(-0.94712590431829,0.183848416855222,0.262968212887203)) ;
#22241=DIRECTION('center_axis',(0.17714714068552,0.982954607100363,-0.0491846615025047)) ;
#22242=DIRECTION('ref_axis',(-0.94712590431829,0.183848416855222,0.262968212887203)) ;
#22243=DIRECTION('center_axis',(0.183578787313568,0.982954607100363,-0.00995335263369857)) ;
#22244=DIRECTION('ref_axis',(-0.981513019488616,0.183848416855221,0.0532160896174226)) ;
#22245=DIRECTION('center_axis',(0.183578787313568,0.982954607100363,-0.00995335263369857)) ;
#22246=DIRECTION('ref_axis',(-0.981513019488616,0.183848416855221,0.0532160896174225)) ;
#22247=DIRECTION('center_axis',(0.183578787313568,0.982954607100363,-0.00995335263369857)) ;
#22248=DIRECTION('ref_axis',(-0.981513019488616,0.183848416855221,0.0532160896174225)) ;
#22249=DIRECTION('center_axis',(0.181426493880004,0.982954607100363,0.0297433639419023)) ;
#22250=DIRECTION('ref_axis',(-0.970005676741023,0.183848416855222,-0.159024358857435)) ;
#22251=DIRECTION('center_axis',(0.181426493880004,0.982954607100363,0.0297433639419023)) ;
#22252=DIRECTION('ref_axis',(-0.970005676741023,0.183848416855222,-0.159024358857435)) ;
#22253=DIRECTION('center_axis',(0.181426493880004,0.982954607100363,0.0297433639419023)) ;
#22254=DIRECTION('ref_axis',(-0.970005676741023,0.183848416855222,-0.159024358857435)) ;
#22255=DIRECTION('center_axis',(0.170790899233673,0.982954607100363,0.068049313876955)) ;
#22256=DIRECTION('ref_axis',(-0.913141946632898,0.183848416855221,-0.363829005055)) ;
#22257=DIRECTION('center_axis',(0.170790899233673,0.982954607100363,0.0680493138769549)) ;
#22258=DIRECTION('ref_axis',(-0.913141946632898,0.183848416855221,-0.363829005055)) ;
#22259=DIRECTION('center_axis',(0.170790899233673,0.982954607100363,0.0680493138769549)) ;
#22260=DIRECTION('ref_axis',(-0.913141946632898,0.183848416855221,-0.363829005055)) ;
#22261=DIRECTION('center_axis',(0.152169311959629,0.982954607100363,0.103173353526501)) ;
#22262=DIRECTION('ref_axis',(-0.813580713984599,0.183848416855221,-0.551621411343086)) ;
#22263=DIRECTION('center_axis',(0.152169311959629,0.982954607100363,0.103173353526501)) ;
#22264=DIRECTION('ref_axis',(-0.813580713984599,0.183848416855221,-0.551621411343086)) ;
#22265=DIRECTION('center_axis',(0.152169311959629,0.982954607100363,0.103173353526501)) ;
#22266=DIRECTION('ref_axis',(-0.813580713984599,0.183848416855221,-0.551621411343086)) ;
#22267=DIRECTION('center_axis',(0.126432456782393,0.982954607100363,0.133473121834094)) ;
#22268=DIRECTION('ref_axis',(-0.675977351380398,0.18384841685522,-0.713620613519937)) ;
#22269=DIRECTION('center_axis',(0.126432456782393,0.982954607100363,0.133473121834094)) ;
#22270=DIRECTION('ref_axis',(-0.675977351380398,0.18384841685522,-0.713620613519937)) ;
#22271=DIRECTION('center_axis',(0.126432456782393,0.982954607100363,0.133473121834094)) ;
#22272=DIRECTION('ref_axis',(-0.675977351380398,0.18384841685522,-0.713620613519937)) ;
#22273=DIRECTION('center_axis',(0.0947837604455978,0.982954607100363,0.157531835309445)) ;
#22274=DIRECTION('ref_axis',(-0.506766039120516,0.18384841685522,-0.84225170894094)) ;
#22275=DIRECTION('center_axis',(0.0947837604455977,0.982954607100363,0.157531835309445)) ;
#22276=DIRECTION('ref_axis',(-0.506766039120516,0.18384841685522,-0.84225170894094)) ;
#22277=DIRECTION('center_axis',(0.0947837604455977,0.982954607100363,0.157531835309445)) ;
#22278=DIRECTION('ref_axis',(-0.506766039120516,0.18384841685522,-0.84225170894094)) ;
#22279=DIRECTION('center_axis',(0.0587030808149489,0.982954607100363,0.174224535249788)) ;
#22280=DIRECTION('ref_axis',(-0.313858910101358,0.183848416855221,-0.931500050547404)) ;
#22281=DIRECTION('center_axis',(0.0587030808149489,0.982954607100363,0.174224535249788)) ;
#22282=DIRECTION('ref_axis',(-0.313858910101358,0.183848416855221,-0.931500050547404)) ;
#22283=DIRECTION('center_axis',(0.0587030808149489,0.982954607100363,0.174224535249788)) ;
#22284=DIRECTION('ref_axis',(-0.313858910101358,0.183848416855221,-0.931500050547404)) ;
#22285=DIRECTION('center_axis',(0.0198775103691822,0.982954607100363,0.182770689558513)) ;
#22286=DIRECTION('ref_axis',(-0.106276087274983,0.183848416855221,-0.977192485078221)) ;
#22287=DIRECTION('center_axis',(0.0198775103691822,0.982954607100363,0.182770689558513)) ;
#22288=DIRECTION('ref_axis',(-0.106276087274983,0.183848416855221,-0.977192485078221)) ;
#22289=DIRECTION('center_axis',(0.0198775103691822,0.982954607100363,0.182770689558513)) ;
#22290=DIRECTION('ref_axis',(-0.106276087274983,0.183848416855221,-0.977192485078221)) ;
#22291=DIRECTION('center_axis',(-0.0198775103691822,0.982954607100363,0.182770689558513)) ;
#22292=DIRECTION('ref_axis',(0.106276087274983,0.183848416855221,-0.977192485078221)) ;
#22293=DIRECTION('center_axis',(-0.0198775103691822,0.982954607100363,0.182770689558513)) ;
#22294=DIRECTION('ref_axis',(0.106276087274983,0.183848416855221,-0.977192485078221)) ;
#22295=DIRECTION('center_axis',(-0.0198775103691822,0.982954607100363,0.182770689558513)) ;
#22296=DIRECTION('ref_axis',(0.106276087274983,0.183848416855221,-0.977192485078221)) ;
#22297=DIRECTION('center_axis',(-0.0587030808149489,0.982954607100363,0.174224535249788)) ;
#22298=DIRECTION('ref_axis',(0.313858910101358,0.183848416855221,-0.931500050547404)) ;
#22299=DIRECTION('center_axis',(-0.0587030808149489,0.982954607100363,0.174224535249788)) ;
#22300=DIRECTION('ref_axis',(0.313858910101358,0.183848416855221,-0.931500050547404)) ;
#22301=DIRECTION('center_axis',(-0.0587030808149489,0.982954607100363,0.174224535249788)) ;
#22302=DIRECTION('ref_axis',(0.313858910101358,0.183848416855221,-0.931500050547404)) ;
#22303=DIRECTION('center_axis',(-0.0947837604455977,0.982954607100363,0.157531835309445)) ;
#22304=DIRECTION('ref_axis',(0.506766039120516,0.18384841685522,-0.842251708940939)) ;
#22305=DIRECTION('center_axis',(-0.0947837604455978,0.982954607100363,0.157531835309445)) ;
#22306=DIRECTION('ref_axis',(0.506766039120516,0.18384841685522,-0.842251708940939)) ;
#22307=DIRECTION('center_axis',(-0.0947837604455978,0.982954607100363,0.157531835309445)) ;
#22308=DIRECTION('ref_axis',(0.506766039120516,0.18384841685522,-0.842251708940939)) ;
#22309=DIRECTION('center_axis',(-0.126432456782393,0.982954607100363,0.133473121834094)) ;
#22310=DIRECTION('ref_axis',(0.6759773513804,0.18384841685522,-0.713620613519935)) ;
#22311=DIRECTION('center_axis',(-0.126432456782393,0.982954607100363,0.133473121834094)) ;
#22312=DIRECTION('ref_axis',(0.6759773513804,0.18384841685522,-0.713620613519935)) ;
#22313=DIRECTION('center_axis',(-0.126432456782393,0.982954607100363,0.133473121834094)) ;
#22314=DIRECTION('ref_axis',(0.6759773513804,0.18384841685522,-0.713620613519935)) ;
#22315=DIRECTION('center_axis',(-0.152169311959629,0.982954607100363,0.103173353526501)) ;
#22316=DIRECTION('ref_axis',(0.813580713984599,0.183848416855221,-0.551621411343086)) ;
#22317=DIRECTION('center_axis',(-0.152169311959629,0.982954607100363,0.103173353526501)) ;
#22318=DIRECTION('ref_axis',(0.813580713984599,0.183848416855221,-0.551621411343086)) ;
#22319=DIRECTION('center_axis',(-0.152169311959629,0.982954607100363,0.103173353526501)) ;
#22320=DIRECTION('ref_axis',(0.813580713984599,0.183848416855221,-0.551621411343086)) ;
#22321=DIRECTION('center_axis',(-0.170790899233673,0.982954607100363,0.068049313876955)) ;
#22322=DIRECTION('ref_axis',(0.913141946632899,0.183848416855221,-0.363829005054997)) ;
#22323=DIRECTION('center_axis',(-0.170790899233673,0.982954607100363,0.0680493138769549)) ;
#22324=DIRECTION('ref_axis',(0.913141946632899,0.183848416855221,-0.363829005054997)) ;
#22325=DIRECTION('center_axis',(-0.170790899233673,0.982954607100363,0.0680493138769549)) ;
#22326=DIRECTION('ref_axis',(0.913141946632899,0.183848416855221,-0.363829005054997)) ;
#22327=DIRECTION('center_axis',(-0.181426493880004,0.982954607100363,0.0297433639419023)) ;
#22328=DIRECTION('ref_axis',(0.970005676741023,0.183848416855222,-0.159024358857436)) ;
#22329=DIRECTION('center_axis',(-0.181426493880004,0.982954607100363,0.0297433639419023)) ;
#22330=DIRECTION('ref_axis',(0.970005676741023,0.183848416855222,-0.159024358857436)) ;
#22331=DIRECTION('center_axis',(-0.181426493880004,0.982954607100363,0.0297433639419023)) ;
#22332=DIRECTION('ref_axis',(0.970005676741023,0.183848416855222,-0.159024358857436)) ;
#22333=DIRECTION('center_axis',(-0.183578787313568,0.982954607100363,-0.00995335263369879)) ;
#22334=DIRECTION('ref_axis',(0.981513019488616,0.183848416855221,0.0532160896174224)) ;
#22335=DIRECTION('center_axis',(-0.183578787313568,0.982954607100363,-0.0099533526336988)) ;
#22336=DIRECTION('ref_axis',(0.981513019488616,0.183848416855221,0.0532160896174224)) ;
#22337=DIRECTION('center_axis',(-0.183578787313568,0.982954607100363,-0.0099533526336988)) ;
#22338=DIRECTION('ref_axis',(0.981513019488616,0.183848416855221,0.0532160896174224)) ;
#22339=DIRECTION('center_axis',(-0.17714714068552,0.982954607100363,-0.0491846615025056)) ;
#22340=DIRECTION('ref_axis',(0.94712590431829,0.183848416855222,0.262968212887203)) ;
#22341=DIRECTION('center_axis',(-0.17714714068552,0.982954607100363,-0.0491846615025056)) ;
#22342=DIRECTION('ref_axis',(0.94712590431829,0.183848416855222,0.262968212887203)) ;
#22343=DIRECTION('center_axis',(-0.17714714068552,0.982954607100363,-0.0491846615025056)) ;
#22344=DIRECTION('ref_axis',(0.94712590431829,0.183848416855222,0.262968212887203)) ;
#22345=DIRECTION('center_axis',(-0.162432290643921,0.982954607100363,-0.0861161502642798)) ;
#22346=DIRECTION('ref_axis',(0.868452234516879,0.183848416855221,0.460424234790556)) ;
#22347=DIRECTION('center_axis',(-0.16243229064392,0.982954607100363,-0.0861161502642798)) ;
#22348=DIRECTION('ref_axis',(0.868452234516879,0.183848416855221,0.460424234790556)) ;
#22349=DIRECTION('center_axis',(-0.16243229064392,0.982954607100363,-0.0861161502642798)) ;
#22350=DIRECTION('ref_axis',(0.868452234516879,0.183848416855221,0.460424234790556)) ;
#22351=DIRECTION('center_axis',(-0.140122287222337,0.982954607100363,-0.119020943550922)) ;
#22352=DIRECTION('ref_axis',(0.749170703444791,0.18384841685522,0.636351331199885)) ;
#22353=DIRECTION('center_axis',(-0.140122287222337,0.982954607100363,-0.119020943550922)) ;
#22354=DIRECTION('ref_axis',(0.749170703444791,0.18384841685522,0.636351331199885)) ;
#22355=DIRECTION('center_axis',(-0.140122287222337,0.982954607100363,-0.119020943550922)) ;
#22356=DIRECTION('ref_axis',(0.749170703444791,0.18384841685522,0.636351331199885)) ;
#22357=DIRECTION('center_axis',(-0.111260321384975,0.982954607100363,-0.146360449799403)) ;
#22358=DIRECTION('ref_axis',(0.594858782923056,0.183848416855222,0.782523346616016)) ;
#22359=DIRECTION('center_axis',(-0.111260321384975,0.982954607100363,-0.146360449799403)) ;
#22360=DIRECTION('ref_axis',(0.594858782923056,0.183848416855222,0.782523346616015)) ;
#22361=DIRECTION('center_axis',(-0.111260321384975,0.982954607100363,-0.146360449799403)) ;
#22362=DIRECTION('ref_axis',(0.594858782923056,0.183848416855222,0.782523346616015)) ;
#22363=DIRECTION('center_axis',(-0.077195946576616,0.982954607100363,-0.166856304083218)) ;
#22364=DIRECTION('ref_axis',(0.412731926849892,0.183848416855221,0.892105440056614)) ;
#22365=DIRECTION('center_axis',(-0.0771959465766159,0.982954607100363,-0.166856304083218)) ;
#22366=DIRECTION('ref_axis',(0.412731926849892,0.183848416855221,0.892105440056614)) ;
#22367=DIRECTION('center_axis',(-0.0771959465766159,0.982954607100363,-0.166856304083218)) ;
#22368=DIRECTION('ref_axis',(0.412731926849892,0.183848416855221,0.892105440056614)) ;
#22369=DIRECTION('center_axis',(-1.83697019872103E-16,-1.,0.)) ;
#22370=DIRECTION('ref_axis',(-6.12323399573677E-17,1.12481983699639E-32,
-1.)) ;
#22371=DIRECTION('center_axis',(-0.0395219751034661,0.982954607100363,-0.179550143035566)) ;
#22372=DIRECTION('ref_axis',(0.211306184595818,0.183848416855221,0.959973674624147)) ;
#22373=DIRECTION('center_axis',(-0.0395219751034661,0.982954607100363,-0.179550143035566)) ;
#22374=DIRECTION('ref_axis',(0.211306184595818,0.183848416855221,0.959973674624147)) ;
#22375=DIRECTION('center_axis',(-0.0395219751034661,0.982954607100363,-0.179550143035566)) ;
#22376=DIRECTION('ref_axis',(0.211306184595818,0.183848416855221,0.959973674624147)) ;
#22377=DIRECTION('center_axis',(1.83697019872103E-16,1.,2.02545731253837E-48)) ;
#22378=DIRECTION('ref_axis',(6.12323399573677E-17,-1.12481983699639E-32,
1.)) ;
#22379=DIRECTION('',(1.46793425709383E-16,-0.183848416855218,0.982954607100364)) ;
#22380=DIRECTION('center_axis',(-1.80565831993891E-16,-0.982954607100363,
0.18384841685522)) ;
#22381=DIRECTION('ref_axis',(1.,-1.84419353919637E-10,-9.8600616806345E-10)) ;
#22382=DIRECTION('center_axis',(1.80565831993891E-16,0.982954607100363,
-0.18384841685522)) ;
#22383=DIRECTION('ref_axis',(6.12323399573677E-17,0.18384841685522,0.982954607100363)) ;
#22384=DIRECTION('center_axis',(1.80565831993891E-16,0.982954607100363,
-0.18384841685522)) ;
#22385=DIRECTION('ref_axis',(6.12323399573677E-17,0.18384841685522,0.982954607100363)) ;
#22386=DIRECTION('center_axis',(-1.80565831993891E-16,-0.982954607100363,
0.18384841685522)) ;
#22387=DIRECTION('ref_axis',(-6.12323399573676E-17,-0.18384841685522,-0.982954607100363)) ;
#22388=DIRECTION('center_axis',(1.80565831993891E-16,0.982954607100363,
-0.18384841685522)) ;
#22389=DIRECTION('ref_axis',(6.12323399573677E-17,0.18384841685522,0.982954607100363)) ;
#22390=DIRECTION('center_axis',(1.80565831993891E-16,0.982954607100363,
-0.18384841685522)) ;
#22391=DIRECTION('ref_axis',(6.12323399573677E-17,0.18384841685522,0.982954607100363)) ;
#22392=DIRECTION('center_axis',(-1.80565831993891E-16,-0.982954607100363,
0.18384841685522)) ;
#22393=DIRECTION('ref_axis',(6.12323399573676E-17,0.18384841685522,0.982954607100363)) ;
#22394=DIRECTION('center_axis',(-0.039521975103467,-0.982954607100363,0.179550143035567)) ;
#22395=DIRECTION('ref_axis',(0.97662278989035,-1.9439115888104E-6,0.21496028996773)) ;
#22396=DIRECTION('center_axis',(0.039521975103467,0.982954607100363,-0.179550143035566)) ;
#22397=DIRECTION('ref_axis',(-0.211306184595818,0.183848416855221,0.959973674624147)) ;
#22398=DIRECTION('center_axis',(0.039521975103467,0.982954607100363,-0.179550143035566)) ;
#22399=DIRECTION('ref_axis',(-0.211306184595818,0.183848416855221,0.959973674624147)) ;
#22400=DIRECTION('center_axis',(-0.039521975103467,-0.982954607100363,0.179550143035566)) ;
#22401=DIRECTION('ref_axis',(0.211306184595818,-0.183848416855221,-0.959973674624147)) ;
#22402=DIRECTION('center_axis',(0.039521975103467,0.982954607100363,-0.179550143035566)) ;
#22403=DIRECTION('ref_axis',(-0.211306184595818,0.183848416855221,0.959973674624147)) ;
#22404=DIRECTION('center_axis',(0.039521975103467,0.982954607100363,-0.179550143035566)) ;
#22405=DIRECTION('ref_axis',(-0.211306184595818,0.183848416855221,0.959973674624147)) ;
#22406=DIRECTION('center_axis',(-0.039521975103467,-0.982954607100363,0.179550143035567)) ;
#22407=DIRECTION('ref_axis',(-0.211306184595818,0.183848416855222,0.959973674624146)) ;
#22408=DIRECTION('center_axis',(-0.0771959465766159,-0.982954607100363,
0.166856304083218)) ;
#22409=DIRECTION('ref_axis',(0.907575420122405,-2.010944117565E-10,0.419889100584476)) ;
#22410=DIRECTION('center_axis',(0.077195946576616,0.982954607100363,-0.166856304083218)) ;
#22411=DIRECTION('ref_axis',(-0.412731926849895,0.183848416855221,0.892105440056612)) ;
#22412=DIRECTION('center_axis',(0.077195946576616,0.982954607100363,-0.166856304083218)) ;
#22413=DIRECTION('ref_axis',(-0.412731926849895,0.183848416855221,0.892105440056612)) ;
#22414=DIRECTION('center_axis',(-0.0771959465766158,-0.982954607100363,
0.166856304083218)) ;
#22415=DIRECTION('ref_axis',(0.412731926849895,-0.183848416855221,-0.892105440056612)) ;
#22416=DIRECTION('center_axis',(0.077195946576616,0.982954607100363,-0.166856304083218)) ;
#22417=DIRECTION('ref_axis',(-0.412731926849895,0.183848416855221,0.892105440056612)) ;
#22418=DIRECTION('center_axis',(0.077195946576616,0.982954607100363,-0.166856304083218)) ;
#22419=DIRECTION('ref_axis',(-0.412731926849895,0.183848416855221,0.892105440056612)) ;
#22420=DIRECTION('center_axis',(-0.0771959465766159,-0.982954607100363,
0.166856304083218)) ;
#22421=DIRECTION('ref_axis',(-0.412731926849895,0.183848416855221,0.892105440056612)) ;
#22422=DIRECTION('center_axis',(-0.111260321384975,-0.982954607100363,0.146360449799403)) ;
#22423=DIRECTION('ref_axis',(0.796093066345906,-1.9788077417699E-10,0.605174214351514)) ;
#22424=DIRECTION('center_axis',(0.111260321384975,0.982954607100363,-0.146360449799403)) ;
#22425=DIRECTION('ref_axis',(-0.594858782923058,0.183848416855222,0.782523346616014)) ;
#22426=DIRECTION('center_axis',(0.111260321384975,0.982954607100363,-0.146360449799403)) ;
#22427=DIRECTION('ref_axis',(-0.594858782923058,0.183848416855222,0.782523346616014)) ;
#22428=DIRECTION('center_axis',(-0.111260321384975,-0.982954607100363,0.146360449799403)) ;
#22429=DIRECTION('ref_axis',(0.594858782923058,-0.183848416855222,-0.782523346616014)) ;
#22430=DIRECTION('center_axis',(0.111260321384975,0.982954607100363,-0.146360449799403)) ;
#22431=DIRECTION('ref_axis',(-0.594858782923058,0.183848416855222,0.782523346616014)) ;
#22432=DIRECTION('center_axis',(0.111260321384975,0.982954607100363,-0.146360449799403)) ;
#22433=DIRECTION('ref_axis',(-0.594858782923058,0.183848416855222,0.782523346616014)) ;
#22434=DIRECTION('center_axis',(-0.111260321384975,-0.982954607100363,0.146360449799403)) ;
#22435=DIRECTION('ref_axis',(-0.594858782923058,0.183848416855222,0.782523346616014)) ;
#22436=DIRECTION('center_axis',(-0.140122287222336,-0.982954607100363,0.119020943550922)) ;
#22437=DIRECTION('ref_axis',(0.647386285486055,-1.72818379975615E-10,0.76216205452946)) ;
#22438=DIRECTION('center_axis',(0.140122287222336,0.982954607100363,-0.119020943550922)) ;
#22439=DIRECTION('ref_axis',(-0.749170703444791,0.18384841685522,0.636351331199885)) ;
#22440=DIRECTION('center_axis',(0.140122287222336,0.982954607100363,-0.119020943550922)) ;
#22441=DIRECTION('ref_axis',(-0.749170703444791,0.18384841685522,0.636351331199885)) ;
#22442=DIRECTION('center_axis',(-0.140122287222336,-0.982954607100363,0.119020943550922)) ;
#22443=DIRECTION('ref_axis',(0.749170703444791,-0.18384841685522,-0.636351331199886)) ;
#22444=DIRECTION('center_axis',(0.140122287222336,0.982954607100363,-0.119020943550922)) ;
#22445=DIRECTION('ref_axis',(-0.749170703444791,0.18384841685522,0.636351331199885)) ;
#22446=DIRECTION('center_axis',(0.140122287222336,0.982954607100363,-0.119020943550922)) ;
#22447=DIRECTION('ref_axis',(-0.749170703444791,0.18384841685522,0.636351331199885)) ;
#22448=DIRECTION('center_axis',(-0.140122287222336,-0.982954607100363,0.119020943550922)) ;
#22449=DIRECTION('ref_axis',(-0.647386285943796,2.8514919837155E-10,-0.762162054140651)) ;
#22450=DIRECTION('center_axis',(-0.162432290643921,-0.982954607100363,0.0861161502642798)) ;
#22451=DIRECTION('ref_axis',(0.468408900302222,-9.72963020982897E-8,0.883511800780077)) ;
#22452=DIRECTION('center_axis',(0.162432290643921,0.982954607100363,-0.0861161502642798)) ;
#22453=DIRECTION('ref_axis',(-0.868452234516879,0.183848416855221,0.460424234790555)) ;
#22454=DIRECTION('center_axis',(0.162432290643921,0.982954607100363,-0.0861161502642798)) ;
#22455=DIRECTION('ref_axis',(-0.868452234516879,0.183848416855221,0.460424234790555)) ;
#22456=DIRECTION('center_axis',(-0.16243229064392,-0.982954607100363,0.0861161502642797)) ;
#22457=DIRECTION('ref_axis',(0.868452234516879,-0.18384841685522,-0.460424234790555)) ;
#22458=DIRECTION('center_axis',(0.162432290643921,0.982954607100363,-0.0861161502642798)) ;
#22459=DIRECTION('ref_axis',(-0.868452234516879,0.183848416855221,0.460424234790555)) ;
#22460=DIRECTION('center_axis',(0.162432290643921,0.982954607100363,-0.0861161502642798)) ;
#22461=DIRECTION('ref_axis',(-0.868452234516879,0.183848416855221,0.460424234790555)) ;
#22462=DIRECTION('center_axis',(-0.162432290643921,-0.982954607100363,0.0861161502642798)) ;
#22463=DIRECTION('ref_axis',(-0.868452234516879,0.183848416855221,0.460424234790555)) ;
#22464=DIRECTION('center_axis',(-0.17714714068552,-0.982954607100363,0.0491846615025047)) ;
#22465=DIRECTION('ref_axis',(0.267536309373971,-1.54723772605301E-6,0.963547779388319)) ;
#22466=DIRECTION('center_axis',(0.17714714068552,0.982954607100363,-0.0491846615025047)) ;
#22467=DIRECTION('ref_axis',(-0.94712590431829,0.183848416855222,0.262968212887203)) ;
#22468=DIRECTION('center_axis',(0.17714714068552,0.982954607100363,-0.0491846615025047)) ;
#22469=DIRECTION('ref_axis',(-0.94712590431829,0.183848416855222,0.262968212887203)) ;
#22470=DIRECTION('center_axis',(-0.17714714068552,-0.982954607100363,0.0491846615025046)) ;
#22471=DIRECTION('ref_axis',(0.94712590431829,-0.183848416855222,-0.262968212887203)) ;
#22472=DIRECTION('center_axis',(0.17714714068552,0.982954607100363,-0.0491846615025047)) ;
#22473=DIRECTION('ref_axis',(-0.94712590431829,0.183848416855222,0.262968212887203)) ;
#22474=DIRECTION('center_axis',(0.17714714068552,0.982954607100363,-0.0491846615025047)) ;
#22475=DIRECTION('ref_axis',(-0.94712590431829,0.183848416855222,0.262968212887203)) ;
#22476=DIRECTION('center_axis',(-0.17714714068552,-0.982954607100363,0.0491846615025047)) ;
#22477=DIRECTION('ref_axis',(-0.94712590431829,0.183848416855222,0.262968212887203)) ;
#22478=DIRECTION('center_axis',(-0.183578787313568,-0.982954607100363,0.00995335263369857)) ;
#22479=DIRECTION('ref_axis',(0.0541389096098241,-1.91882817342339E-10,0.998533413795582)) ;
#22480=DIRECTION('center_axis',(0.183578787313568,0.982954607100363,-0.00995335263369857)) ;
#22481=DIRECTION('ref_axis',(-0.981513019488616,0.183848416855221,0.0532160896174226)) ;
#22482=DIRECTION('center_axis',(0.183578787313568,0.982954607100363,-0.00995335263369857)) ;
#22483=DIRECTION('ref_axis',(-0.981513019488616,0.183848416855221,0.0532160896174226)) ;
#22484=DIRECTION('center_axis',(-0.183578787313568,-0.982954607100363,0.00995335263369856)) ;
#22485=DIRECTION('ref_axis',(0.981513019488616,-0.183848416855221,-0.0532160896174226)) ;
#22486=DIRECTION('center_axis',(0.183578787313568,0.982954607100363,-0.00995335263369857)) ;
#22487=DIRECTION('ref_axis',(-0.981513019488616,0.183848416855221,0.0532160896174226)) ;
#22488=DIRECTION('center_axis',(0.183578787313568,0.982954607100363,-0.00995335263369857)) ;
#22489=DIRECTION('ref_axis',(-0.981513019488616,0.183848416855221,0.0532160896174226)) ;
#22490=DIRECTION('center_axis',(-0.183578787313568,-0.982954607100363,0.00995335263369857)) ;
#22491=DIRECTION('ref_axis',(-0.981513019488616,0.183848416855221,0.0532160896174226)) ;
#22492=DIRECTION('center_axis',(-0.181426493880004,-0.982954607100363,-0.0297433639419023)) ;
#22493=DIRECTION('ref_axis',(-0.161781995558069,-1.88527458823811E-10,0.986826522704598)) ;
#22494=DIRECTION('center_axis',(0.181426493880004,0.982954607100363,0.0297433639419023)) ;
#22495=DIRECTION('ref_axis',(-0.970005676741023,0.183848416855222,-0.159024358857435)) ;
#22496=DIRECTION('center_axis',(0.181426493880004,0.982954607100363,0.0297433639419023)) ;
#22497=DIRECTION('ref_axis',(-0.970005676741023,0.183848416855222,-0.159024358857435)) ;
#22498=DIRECTION('center_axis',(-0.181426493880003,-0.982954607100363,-0.0297433639419022)) ;
#22499=DIRECTION('ref_axis',(0.970005676741023,-0.183848416855221,0.159024358857435)) ;
#22500=DIRECTION('center_axis',(0.181426493880004,0.982954607100363,0.0297433639419023)) ;
#22501=DIRECTION('ref_axis',(-0.970005676741023,0.183848416855222,-0.159024358857435)) ;
#22502=DIRECTION('center_axis',(0.181426493880004,0.982954607100363,0.0297433639419023)) ;
#22503=DIRECTION('ref_axis',(-0.970005676741023,0.183848416855222,-0.159024358857435)) ;
#22504=DIRECTION('center_axis',(-0.181426493880004,-0.982954607100363,-0.0297433639419023)) ;
#22505=DIRECTION('ref_axis',(0.161781994932387,3.07115069039933E-10,-0.986826522807174)) ;
#22506=DIRECTION('center_axis',(-0.170790899233673,-0.982954607100363,-0.0680493138769549)) ;
#22507=DIRECTION('ref_axis',(-0.370138154397863,-1.89668830078089E-10,0.928976720192139)) ;
#22508=DIRECTION('center_axis',(0.170790899233673,0.982954607100363,0.0680493138769549)) ;
#22509=DIRECTION('ref_axis',(-0.913141946632898,0.183848416855221,-0.363829005055)) ;
#22510=DIRECTION('center_axis',(0.170790899233673,0.982954607100363,0.0680493138769549)) ;
#22511=DIRECTION('ref_axis',(-0.913141946632898,0.183848416855221,-0.363829005055)) ;
#22512=DIRECTION('center_axis',(-0.170790899233673,-0.982954607100363,-0.0680493138769549)) ;
#22513=DIRECTION('ref_axis',(0.913141946632898,-0.183848416855221,0.363829005055)) ;
#22514=DIRECTION('center_axis',(0.170790899233673,0.982954607100363,0.0680493138769549)) ;
#22515=DIRECTION('ref_axis',(-0.913141946632898,0.183848416855221,-0.363829005055)) ;
#22516=DIRECTION('center_axis',(0.170790899233673,0.982954607100363,0.0680493138769549)) ;
#22517=DIRECTION('ref_axis',(-0.913141946632898,0.183848416855221,-0.363829005055)) ;
#22518=DIRECTION('center_axis',(-0.170790899233673,-0.982954607100363,-0.0680493138769549)) ;
#22519=DIRECTION('ref_axis',(-0.913141946632898,0.183848416855221,-0.363829005055)) ;
#22520=DIRECTION('center_axis',(-0.152169311959629,-0.982954607100363,-0.103173353526501)) ;
#22521=DIRECTION('ref_axis',(-0.561187064344022,-2.30122606296928E-10,0.827688998847356)) ;
#22522=DIRECTION('center_axis',(0.152169311959629,0.982954607100363,0.103173353526501)) ;
#22523=DIRECTION('ref_axis',(-0.8135807139846,0.183848416855221,-0.551621411343086)) ;
#22524=DIRECTION('center_axis',(0.152169311959629,0.982954607100363,0.103173353526501)) ;
#22525=DIRECTION('ref_axis',(-0.8135807139846,0.183848416855221,-0.551621411343086)) ;
#22526=DIRECTION('center_axis',(-0.152169311959628,-0.982954607100363,-0.1031733535265)) ;
#22527=DIRECTION('ref_axis',(0.8135807139846,-0.18384841685522,0.551621411343086)) ;
#22528=DIRECTION('center_axis',(0.152169311959629,0.982954607100363,0.103173353526501)) ;
#22529=DIRECTION('ref_axis',(-0.8135807139846,0.183848416855221,-0.551621411343086)) ;
#22530=DIRECTION('center_axis',(0.152169311959629,0.982954607100363,0.103173353526501)) ;
#22531=DIRECTION('ref_axis',(-0.8135807139846,0.183848416855221,-0.551621411343086)) ;
#22532=DIRECTION('center_axis',(-0.152169311959629,-0.982954607100363,-0.103173353526501)) ;
#22533=DIRECTION('ref_axis',(-0.813580713984599,0.183848416855221,-0.551621411343086)) ;
#22534=DIRECTION('center_axis',(-0.126432456782393,-0.982954607100363,-0.133473121834094)) ;
#22535=DIRECTION('ref_axis',(-0.725995491248325,-1.83529846792861E-10,0.687699459565807)) ;
#22536=DIRECTION('center_axis',(0.126432456782393,0.982954607100363,0.133473121834094)) ;
#22537=DIRECTION('ref_axis',(-0.675977351380398,0.18384841685522,-0.713620613519937)) ;
#22538=DIRECTION('center_axis',(0.126432456782393,0.982954607100363,0.133473121834094)) ;
#22539=DIRECTION('ref_axis',(-0.675977351380398,0.18384841685522,-0.713620613519937)) ;
#22540=DIRECTION('center_axis',(-0.126432456782393,-0.982954607100363,-0.133473121834093)) ;
#22541=DIRECTION('ref_axis',(0.675977351380398,-0.183848416855219,0.713620613519937)) ;
#22542=DIRECTION('center_axis',(0.126432456782393,0.982954607100363,0.133473121834094)) ;
#22543=DIRECTION('ref_axis',(-0.675977351380398,0.18384841685522,-0.713620613519937)) ;
#22544=DIRECTION('center_axis',(0.126432456782393,0.982954607100363,0.133473121834094)) ;
#22545=DIRECTION('ref_axis',(-0.675977351380398,0.18384841685522,-0.713620613519937)) ;
#22546=DIRECTION('center_axis',(-0.126432456782393,-0.982954607100363,-0.133473121834094)) ;
#22547=DIRECTION('ref_axis',(-0.675977351380398,0.18384841685522,-0.713620613519937)) ;
#22548=DIRECTION('center_axis',(-0.0947837604455977,-0.982954607100363,
-0.157531835309445)) ;
#22549=DIRECTION('ref_axis',(-0.856857175641539,-1.90844127298985E-10,0.515553858051324)) ;
#22550=DIRECTION('center_axis',(0.0947837604455977,0.982954607100363,0.157531835309445)) ;
#22551=DIRECTION('ref_axis',(-0.506766039120516,0.18384841685522,-0.84225170894094)) ;
#22552=DIRECTION('center_axis',(0.0947837604455977,0.982954607100363,0.157531835309445)) ;
#22553=DIRECTION('ref_axis',(-0.506766039120516,0.18384841685522,-0.84225170894094)) ;
#22554=DIRECTION('center_axis',(-0.0947837604455976,-0.982954607100363,
-0.157531835309445)) ;
#22555=DIRECTION('ref_axis',(0.506766039120516,-0.18384841685522,0.84225170894094)) ;
#22556=DIRECTION('center_axis',(0.0947837604455977,0.982954607100363,0.157531835309445)) ;
#22557=DIRECTION('ref_axis',(-0.506766039120516,0.18384841685522,-0.84225170894094)) ;
#22558=DIRECTION('center_axis',(0.0947837604455977,0.982954607100363,0.157531835309445)) ;
#22559=DIRECTION('ref_axis',(-0.506766039120516,0.18384841685522,-0.84225170894094)) ;
#22560=DIRECTION('center_axis',(-0.0947837604455977,-0.982954607100363,
-0.157531835309445)) ;
#22561=DIRECTION('ref_axis',(-0.506766039120516,0.18384841685522,-0.84225170894094)) ;
#22562=DIRECTION('center_axis',(-0.0587030808149489,-0.982954607100363,
-0.174224535249788)) ;
#22563=DIRECTION('ref_axis',(-0.94765317085513,-1.91940387467248E-10,0.319301531108476)) ;
#22564=DIRECTION('center_axis',(0.058703080814949,0.982954607100363,0.174224535249788)) ;
#22565=DIRECTION('ref_axis',(-0.313858910101358,0.183848416855221,-0.931500050547404)) ;
#22566=DIRECTION('center_axis',(0.058703080814949,0.982954607100363,0.174224535249788)) ;
#22567=DIRECTION('ref_axis',(-0.313858910101358,0.183848416855221,-0.931500050547404)) ;
#22568=DIRECTION('center_axis',(-0.0587030808149489,-0.982954607100363,
-0.174224535249788)) ;
#22569=DIRECTION('ref_axis',(0.313858910101358,-0.183848416855221,0.931500050547404)) ;
#22570=DIRECTION('center_axis',(0.058703080814949,0.982954607100363,0.174224535249788)) ;
#22571=DIRECTION('ref_axis',(-0.313858910101358,0.183848416855221,-0.931500050547404)) ;
#22572=DIRECTION('center_axis',(0.058703080814949,0.982954607100363,0.174224535249788)) ;
#22573=DIRECTION('ref_axis',(-0.313858910101358,0.183848416855221,-0.931500050547404)) ;
#22574=DIRECTION('center_axis',(-0.0587030808149489,-0.982954607100363,
-0.174224535249788)) ;
#22575=DIRECTION('ref_axis',(-0.313858910101358,0.183848416855221,-0.931500050547404)) ;
#22576=DIRECTION('center_axis',(-0.0198775103691822,-0.982954607100363,
-0.182770689558513)) ;
#22577=DIRECTION('ref_axis',(-0.994137957045046,-1.89103119640252E-10,0.108119019429064)) ;
#22578=DIRECTION('center_axis',(0.0198775103691822,0.982954607100363,0.182770689558513)) ;
#22579=DIRECTION('ref_axis',(-0.106276087274983,0.183848416855221,-0.977192485078221)) ;
#22580=DIRECTION('center_axis',(0.0198775103691822,0.982954607100363,0.182770689558513)) ;
#22581=DIRECTION('ref_axis',(-0.106276087274983,0.183848416855221,-0.977192485078221)) ;
#22582=DIRECTION('center_axis',(-0.0198775103691822,-0.982954607100363,
-0.182770689558513)) ;
#22583=DIRECTION('ref_axis',(0.106276087274983,-0.183848416855221,0.977192485078221)) ;
#22584=DIRECTION('center_axis',(0.0198775103691822,0.982954607100363,0.182770689558513)) ;
#22585=DIRECTION('ref_axis',(-0.106276087274983,0.183848416855221,-0.977192485078221)) ;
#22586=DIRECTION('center_axis',(0.0198775103691822,0.982954607100363,0.182770689558513)) ;
#22587=DIRECTION('ref_axis',(-0.106276087274983,0.183848416855221,-0.977192485078221)) ;
#22588=DIRECTION('center_axis',(-0.0198775103691822,-0.982954607100363,
-0.182770689558513)) ;
#22589=DIRECTION('ref_axis',(-0.106276087274983,0.183848416855221,-0.977192485078221)) ;
#22590=DIRECTION('center_axis',(0.0198775103691822,-0.982954607100363,-0.182770689558513)) ;
#22591=DIRECTION('ref_axis',(-0.994137957268381,-1.97246615825675E-10,-0.108119017375535)) ;
#22592=DIRECTION('center_axis',(-0.0198775103691822,0.982954607100363,0.182770689558513)) ;
#22593=DIRECTION('ref_axis',(0.106276087274983,0.183848416855221,-0.977192485078221)) ;
#22594=DIRECTION('center_axis',(-0.0198775103691822,0.982954607100363,0.182770689558513)) ;
#22595=DIRECTION('ref_axis',(0.106276087274983,0.183848416855221,-0.977192485078221)) ;
#22596=DIRECTION('center_axis',(0.0198775103691822,-0.982954607100363,-0.182770689558513)) ;
#22597=DIRECTION('ref_axis',(-0.106276087274983,-0.183848416855221,0.977192485078221)) ;
#22598=DIRECTION('center_axis',(-0.0198775103691822,0.982954607100363,0.182770689558513)) ;
#22599=DIRECTION('ref_axis',(0.106276087274983,0.183848416855221,-0.977192485078221)) ;
#22600=DIRECTION('center_axis',(-0.0198775103691822,0.982954607100363,0.182770689558513)) ;
#22601=DIRECTION('ref_axis',(0.106276087274983,0.183848416855221,-0.977192485078221)) ;
#22602=DIRECTION('center_axis',(0.0198775103691822,-0.982954607100363,-0.182770689558513)) ;
#22603=DIRECTION('ref_axis',(0.106276087274983,0.183848416855221,-0.977192485078221)) ;
#22604=DIRECTION('center_axis',(0.0587030808149489,-0.982954607100363,-0.174224535249788)) ;
#22605=DIRECTION('ref_axis',(-0.947653171526354,-2.01240630102731E-10,-0.319301529116356)) ;
#22606=DIRECTION('center_axis',(-0.058703080814949,0.982954607100363,0.174224535249788)) ;
#22607=DIRECTION('ref_axis',(0.313858910101358,0.183848416855221,-0.931500050547404)) ;
#22608=DIRECTION('center_axis',(-0.058703080814949,0.982954607100363,0.174224535249788)) ;
#22609=DIRECTION('ref_axis',(0.313858910101358,0.183848416855221,-0.931500050547404)) ;
#22610=DIRECTION('center_axis',(0.0587030808149489,-0.982954607100363,-0.174224535249788)) ;
#22611=DIRECTION('ref_axis',(-0.313858910101358,-0.183848416855221,0.931500050547404)) ;
#22612=DIRECTION('center_axis',(-0.058703080814949,0.982954607100363,0.174224535249788)) ;
#22613=DIRECTION('ref_axis',(0.313858910101358,0.183848416855221,-0.931500050547404)) ;
#22614=DIRECTION('center_axis',(-0.058703080814949,0.982954607100363,0.174224535249788)) ;
#22615=DIRECTION('ref_axis',(0.313858910101358,0.183848416855221,-0.931500050547404)) ;
#22616=DIRECTION('center_axis',(0.0587030808149489,-0.982954607100363,-0.174224535249788)) ;
#22617=DIRECTION('ref_axis',(0.313858910101358,0.183848416855221,-0.931500050547404)) ;
#22618=DIRECTION('center_axis',(0.0947837604455977,-0.982954607100363,-0.157531835309445)) ;
#22619=DIRECTION('ref_axis',(-0.856857176687482,-1.88611019607742E-10,-0.515553856312953)) ;
#22620=DIRECTION('center_axis',(-0.0947837604455977,0.982954607100363,0.157531835309445)) ;
#22621=DIRECTION('ref_axis',(0.506766039120516,0.18384841685522,-0.842251708940939)) ;
#22622=DIRECTION('center_axis',(-0.0947837604455977,0.982954607100363,0.157531835309445)) ;
#22623=DIRECTION('ref_axis',(0.506766039120516,0.18384841685522,-0.842251708940939)) ;
#22624=DIRECTION('center_axis',(0.0947837604455976,-0.982954607100363,-0.157531835309445)) ;
#22625=DIRECTION('ref_axis',(-0.506766039120516,-0.18384841685522,0.84225170894094)) ;
#22626=DIRECTION('center_axis',(-0.0947837604455977,0.982954607100363,0.157531835309445)) ;
#22627=DIRECTION('ref_axis',(0.506766039120516,0.18384841685522,-0.842251708940939)) ;
#22628=DIRECTION('center_axis',(-0.0947837604455977,0.982954607100363,0.157531835309445)) ;
#22629=DIRECTION('ref_axis',(0.506766039120516,0.18384841685522,-0.842251708940939)) ;
#22630=DIRECTION('center_axis',(0.0947837604455977,-0.982954607100363,-0.157531835309445)) ;
#22631=DIRECTION('ref_axis',(0.506766039120516,0.18384841685522,-0.842251708940939)) ;
#22632=DIRECTION('center_axis',(0.126432456782393,-0.982954607100363,-0.133473121834094)) ;
#22633=DIRECTION('ref_axis',(-0.725995492549092,-1.70245240902753E-10,-0.687699458192604)) ;
#22634=DIRECTION('center_axis',(-0.126432456782393,0.982954607100363,0.133473121834094)) ;
#22635=DIRECTION('ref_axis',(0.6759773513804,0.18384841685522,-0.713620613519935)) ;
#22636=DIRECTION('center_axis',(-0.126432456782393,0.982954607100363,0.133473121834094)) ;
#22637=DIRECTION('ref_axis',(0.6759773513804,0.18384841685522,-0.713620613519935)) ;
#22638=DIRECTION('center_axis',(0.126432456782393,-0.982954607100363,-0.133473121834093)) ;
#22639=DIRECTION('ref_axis',(-0.6759773513804,-0.183848416855219,0.713620613519935)) ;
#22640=DIRECTION('center_axis',(-0.126432456782393,0.982954607100363,0.133473121834094)) ;
#22641=DIRECTION('ref_axis',(0.6759773513804,0.18384841685522,-0.713620613519935)) ;
#22642=DIRECTION('center_axis',(-0.126432456782393,0.982954607100363,0.133473121834094)) ;
#22643=DIRECTION('ref_axis',(0.6759773513804,0.18384841685522,-0.713620613519935)) ;
#22644=DIRECTION('center_axis',(0.126432456782393,-0.982954607100363,-0.133473121834094)) ;
#22645=DIRECTION('ref_axis',(0.725995492955948,2.80899485909582E-10,0.687699457763092)) ;
#22646=DIRECTION('center_axis',(0.152169311959629,-0.982954607100363,-0.103173353526501)) ;
#22647=DIRECTION('ref_axis',(-0.561187066188927,-1.86778640161647E-10,-0.82768899759648)) ;
#22648=DIRECTION('center_axis',(-0.152169311959629,0.982954607100363,0.103173353526501)) ;
#22649=DIRECTION('ref_axis',(0.813580713984599,0.183848416855221,-0.551621411343086)) ;
#22650=DIRECTION('center_axis',(-0.152169311959629,0.982954607100363,0.103173353526501)) ;
#22651=DIRECTION('ref_axis',(0.813580713984599,0.183848416855221,-0.551621411343086)) ;
#22652=DIRECTION('center_axis',(0.152169311959628,-0.982954607100363,-0.1031733535265)) ;
#22653=DIRECTION('ref_axis',(-0.813580713984599,-0.18384841685522,0.551621411343087)) ;
#22654=DIRECTION('center_axis',(-0.152169311959629,0.982954607100363,0.103173353526501)) ;
#22655=DIRECTION('ref_axis',(0.813580713984599,0.183848416855221,-0.551621411343086)) ;
#22656=DIRECTION('center_axis',(-0.152169311959629,0.982954607100363,0.103173353526501)) ;
#22657=DIRECTION('ref_axis',(0.813580713984599,0.183848416855221,-0.551621411343086)) ;
#22658=DIRECTION('center_axis',(0.152169311959629,-0.982954607100363,-0.103173353526501)) ;
#22659=DIRECTION('ref_axis',(0.561187066725594,3.0805171850785E-10,0.82768899723261)) ;
#22660=DIRECTION('center_axis',(0.170790899233673,-0.982954607100363,-0.068049313876955)) ;
#22661=DIRECTION('ref_axis',(-0.370138156273929,-1.88050831664856E-10,-0.928976719444646)) ;
#22662=DIRECTION('center_axis',(-0.170790899233673,0.982954607100363,0.0680493138769549)) ;
#22663=DIRECTION('ref_axis',(0.913141946632899,0.183848416855221,-0.363829005054997)) ;
#22664=DIRECTION('center_axis',(-0.170790899233673,0.982954607100363,0.0680493138769549)) ;
#22665=DIRECTION('ref_axis',(0.913141946632899,0.183848416855221,-0.363829005054997)) ;
#22666=DIRECTION('center_axis',(0.170790899233673,-0.982954607100363,-0.0680493138769549)) ;
#22667=DIRECTION('ref_axis',(-0.913141946632899,-0.183848416855221,0.363829005054997)) ;
#22668=DIRECTION('center_axis',(-0.170790899233673,0.982954607100363,0.0680493138769549)) ;
#22669=DIRECTION('ref_axis',(0.913141946632899,0.183848416855221,-0.363829005054997)) ;
#22670=DIRECTION('center_axis',(-0.170790899233673,0.982954607100363,0.0680493138769549)) ;
#22671=DIRECTION('ref_axis',(0.913141946632899,0.183848416855221,-0.363829005054997)) ;
#22672=DIRECTION('center_axis',(0.170790899233673,-0.982954607100363,-0.068049313876955)) ;
#22673=DIRECTION('ref_axis',(0.913141946632899,0.183848416855221,-0.363829005054997)) ;
#22674=DIRECTION('center_axis',(0.181426493880004,-0.982954607100363,-0.0297433639419023)) ;
#22675=DIRECTION('ref_axis',(-0.161781997642536,-2.06548540774157E-10,-0.986826522362867)) ;
#22676=DIRECTION('center_axis',(-0.181426493880004,0.982954607100363,0.0297433639419023)) ;
#22677=DIRECTION('ref_axis',(0.970005676741023,0.183848416855222,-0.159024358857436)) ;
#22678=DIRECTION('center_axis',(-0.181426493880004,0.982954607100363,0.0297433639419023)) ;
#22679=DIRECTION('ref_axis',(0.970005676741023,0.183848416855222,-0.159024358857436)) ;
#22680=DIRECTION('center_axis',(0.181426493880003,-0.982954607100363,-0.0297433639419022)) ;
#22681=DIRECTION('ref_axis',(-0.970005676741023,-0.183848416855221,0.159024358857436)) ;
#22682=DIRECTION('center_axis',(-0.181426493880004,0.982954607100363,0.0297433639419023)) ;
#22683=DIRECTION('ref_axis',(0.970005676741023,0.183848416855222,-0.159024358857436)) ;
#22684=DIRECTION('center_axis',(-0.181426493880004,0.982954607100363,0.0297433639419023)) ;
#22685=DIRECTION('ref_axis',(0.970005676741023,0.183848416855222,-0.159024358857436)) ;
#22686=DIRECTION('center_axis',(0.181426493880004,-0.982954607100363,-0.0297433639419023)) ;
#22687=DIRECTION('ref_axis',(0.970005676741023,0.183848416855222,-0.159024358857436)) ;
#22688=DIRECTION('center_axis',(0.183578787313568,-0.982954607100363,0.0099533526336988)) ;
#22689=DIRECTION('ref_axis',(0.0541389075565303,-1.92722421117335E-10,-0.998533413906909)) ;
#22690=DIRECTION('center_axis',(-0.183578787313568,0.982954607100363,-0.00995335263369879)) ;
#22691=DIRECTION('ref_axis',(0.981513019488616,0.183848416855221,0.0532160896174224)) ;
#22692=DIRECTION('center_axis',(-0.183578787313568,0.982954607100363,-0.00995335263369879)) ;
#22693=DIRECTION('ref_axis',(0.981513019488616,0.183848416855221,0.0532160896174224)) ;
#22694=DIRECTION('center_axis',(0.183578787313568,-0.982954607100363,0.00995335263369878)) ;
#22695=DIRECTION('ref_axis',(-0.981513019488616,-0.183848416855221,-0.0532160896174224)) ;
#22696=DIRECTION('center_axis',(-0.183578787313568,0.982954607100363,-0.00995335263369879)) ;
#22697=DIRECTION('ref_axis',(0.981513019488616,0.183848416855221,0.0532160896174224)) ;
#22698=DIRECTION('center_axis',(-0.183578787313568,0.982954607100363,-0.00995335263369879)) ;
#22699=DIRECTION('ref_axis',(0.981513019488616,0.183848416855221,0.0532160896174224)) ;
#22700=DIRECTION('center_axis',(0.183578787313568,-0.982954607100363,0.0099533526336988)) ;
#22701=DIRECTION('ref_axis',(0.981513019488616,0.183848416855221,0.0532160896174224)) ;
#22702=DIRECTION('center_axis',(0.17714714068552,-0.982954607100363,0.0491846615025056)) ;
#22703=DIRECTION('ref_axis',(0.267536928724841,1.66746140147225E-6,-0.963547607420463)) ;
#22704=DIRECTION('center_axis',(-0.17714714068552,0.982954607100363,-0.0491846615025056)) ;
#22705=DIRECTION('ref_axis',(0.94712590431829,0.183848416855222,0.262968212887203)) ;
#22706=DIRECTION('center_axis',(-0.17714714068552,0.982954607100363,-0.0491846615025056)) ;
#22707=DIRECTION('ref_axis',(0.94712590431829,0.183848416855222,0.262968212887203)) ;
#22708=DIRECTION('center_axis',(0.17714714068552,-0.982954607100363,0.0491846615025055)) ;
#22709=DIRECTION('ref_axis',(-0.94712590431829,-0.183848416855222,-0.262968212887203)) ;
#22710=DIRECTION('center_axis',(-0.17714714068552,0.982954607100363,-0.0491846615025056)) ;
#22711=DIRECTION('ref_axis',(0.94712590431829,0.183848416855222,0.262968212887203)) ;
#22712=DIRECTION('center_axis',(-0.17714714068552,0.982954607100363,-0.0491846615025056)) ;
#22713=DIRECTION('ref_axis',(0.94712590431829,0.183848416855222,0.262968212887203)) ;
#22714=DIRECTION('center_axis',(0.17714714068552,-0.982954607100363,0.0491846615025056)) ;
#22715=DIRECTION('ref_axis',(-0.267536930966008,-1.66789643976773E-6,0.963547606798184)) ;
#22716=DIRECTION('center_axis',(0.16243229064392,-0.982954607100363,0.0861161502642798)) ;
#22717=DIRECTION('ref_axis',(0.468408439795022,-1.91537394307718E-10,-0.8835120449257)) ;
#22718=DIRECTION('center_axis',(-0.16243229064392,0.982954607100363,-0.0861161502642798)) ;
#22719=DIRECTION('ref_axis',(0.868452234516879,0.18384841685522,0.460424234790556)) ;
#22720=DIRECTION('center_axis',(-0.16243229064392,0.982954607100363,-0.0861161502642798)) ;
#22721=DIRECTION('ref_axis',(0.868452234516879,0.18384841685522,0.460424234790556)) ;
#22722=DIRECTION('center_axis',(0.16243229064392,-0.982954607100363,0.0861161502642797)) ;
#22723=DIRECTION('ref_axis',(-0.868452234516879,-0.183848416855221,-0.460424234790556)) ;
#22724=DIRECTION('center_axis',(-0.16243229064392,0.982954607100363,-0.0861161502642798)) ;
#22725=DIRECTION('ref_axis',(0.868452234516879,0.18384841685522,0.460424234790556)) ;
#22726=DIRECTION('center_axis',(-0.16243229064392,0.982954607100363,-0.0861161502642798)) ;
#22727=DIRECTION('ref_axis',(0.868452234516879,0.18384841685522,0.460424234790556)) ;
#22728=DIRECTION('center_axis',(0.16243229064392,-0.982954607100363,0.0861161502642798)) ;
#22729=DIRECTION('ref_axis',(0.868452234516879,0.183848416855221,0.460424234790556)) ;
#22730=DIRECTION('center_axis',(0.140122287222337,-0.982954607100363,0.119020943550922)) ;
#22731=DIRECTION('ref_axis',(0.647386284015078,-1.88162500161902E-10,-0.762162055778919)) ;
#22732=DIRECTION('center_axis',(-0.140122287222336,0.982954607100363,-0.119020943550922)) ;
#22733=DIRECTION('ref_axis',(0.749170703444791,0.18384841685522,0.636351331199885)) ;
#22734=DIRECTION('center_axis',(-0.140122287222336,0.982954607100363,-0.119020943550922)) ;
#22735=DIRECTION('ref_axis',(0.749170703444791,0.18384841685522,0.636351331199885)) ;
#22736=DIRECTION('center_axis',(0.140122287222336,-0.982954607100363,0.119020943550922)) ;
#22737=DIRECTION('ref_axis',(-0.749170703444791,-0.18384841685522,-0.636351331199885)) ;
#22738=DIRECTION('center_axis',(-0.140122287222336,0.982954607100363,-0.119020943550922)) ;
#22739=DIRECTION('ref_axis',(0.749170703444791,0.18384841685522,0.636351331199885)) ;
#22740=DIRECTION('center_axis',(-0.140122287222336,0.982954607100363,-0.119020943550922)) ;
#22741=DIRECTION('ref_axis',(0.749170703444791,0.18384841685522,0.636351331199885)) ;
#22742=DIRECTION('center_axis',(0.140122287222337,-0.982954607100363,0.119020943550922)) ;
#22743=DIRECTION('ref_axis',(0.749170703444791,0.18384841685522,0.636351331199885)) ;
#22744=DIRECTION('center_axis',(0.111260321384975,-0.982954607100363,0.146360449799403)) ;
#22745=DIRECTION('ref_axis',(0.796093065116338,-1.82132464471827E-10,-0.605174215968984)) ;
#22746=DIRECTION('center_axis',(-0.111260321384975,0.982954607100363,-0.146360449799403)) ;
#22747=DIRECTION('ref_axis',(0.594858782923056,0.183848416855222,0.782523346616016)) ;
#22748=DIRECTION('center_axis',(-0.111260321384975,0.982954607100363,-0.146360449799403)) ;
#22749=DIRECTION('ref_axis',(0.594858782923056,0.183848416855222,0.782523346616016)) ;
#22750=DIRECTION('center_axis',(0.111260321384975,-0.982954607100363,0.146360449799402)) ;
#22751=DIRECTION('ref_axis',(-0.594858782923056,-0.183848416855221,-0.782523346616016)) ;
#22752=DIRECTION('center_axis',(-0.111260321384975,0.982954607100363,-0.146360449799403)) ;
#22753=DIRECTION('ref_axis',(0.594858782923056,0.183848416855222,0.782523346616016)) ;
#22754=DIRECTION('center_axis',(-0.111260321384975,0.982954607100363,-0.146360449799403)) ;
#22755=DIRECTION('ref_axis',(0.594858782923056,0.183848416855222,0.782523346616016)) ;
#22756=DIRECTION('center_axis',(0.111260321384975,-0.982954607100363,0.146360449799403)) ;
#22757=DIRECTION('ref_axis',(-0.796093064783972,2.84854260519924E-10,0.605174216406204)) ;
#22758=DIRECTION('center_axis',(0.0771959465766159,-0.982954607100363,0.166856304083218)) ;
#22759=DIRECTION('ref_axis',(0.907575419211193,-2.04798413077975E-10,-0.419889102554029)) ;
#22760=DIRECTION('center_axis',(-0.0771959465766159,0.982954607100363,-0.166856304083218)) ;
#22761=DIRECTION('ref_axis',(0.412731926849892,0.183848416855221,0.892105440056614)) ;
#22762=DIRECTION('center_axis',(-0.0771959465766159,0.982954607100363,-0.166856304083218)) ;
#22763=DIRECTION('ref_axis',(0.412731926849892,0.183848416855221,0.892105440056614)) ;
#22764=DIRECTION('center_axis',(0.0771959465766158,-0.982954607100363,0.166856304083218)) ;
#22765=DIRECTION('ref_axis',(-0.412731926849892,-0.183848416855221,-0.892105440056614)) ;
#22766=DIRECTION('center_axis',(-0.0771959465766159,0.982954607100363,-0.166856304083218)) ;
#22767=DIRECTION('ref_axis',(0.412731926849892,0.183848416855221,0.892105440056614)) ;
#22768=DIRECTION('center_axis',(-0.0771959465766159,0.982954607100363,-0.166856304083218)) ;
#22769=DIRECTION('ref_axis',(0.412731926849892,0.183848416855221,0.892105440056614)) ;
#22770=DIRECTION('center_axis',(0.0771959465766159,-0.982954607100363,0.166856304083218)) ;
#22771=DIRECTION('ref_axis',(0.412731926849892,0.183848416855221,0.892105440056614)) ;
#22772=DIRECTION('center_axis',(0.0395219751034661,-0.982954607100363,0.179550143035567)) ;
#22773=DIRECTION('ref_axis',(0.976622826934841,1.97614399321564E-6,-0.214960121664217)) ;
#22774=DIRECTION('center_axis',(-0.0395219751034661,0.982954607100363,-0.179550143035566)) ;
#22775=DIRECTION('ref_axis',(0.211306184595818,0.183848416855221,0.959973674624147)) ;
#22776=DIRECTION('center_axis',(-0.0395219751034661,0.982954607100363,-0.179550143035566)) ;
#22777=DIRECTION('ref_axis',(0.211306184595818,0.183848416855221,0.959973674624147)) ;
#22778=DIRECTION('center_axis',(0.0395219751034661,-0.982954607100363,0.179550143035566)) ;
#22779=DIRECTION('ref_axis',(-0.211306184595818,-0.183848416855221,-0.959973674624147)) ;
#22780=DIRECTION('center_axis',(-0.0395219751034661,0.982954607100363,-0.179550143035566)) ;
#22781=DIRECTION('ref_axis',(0.211306184595818,0.183848416855221,0.959973674624147)) ;
#22782=DIRECTION('center_axis',(-0.0395219751034661,0.982954607100363,-0.179550143035566)) ;
#22783=DIRECTION('ref_axis',(0.211306184595818,0.183848416855221,0.959973674624147)) ;
#22784=DIRECTION('center_axis',(0.0395219751034661,-0.982954607100363,0.179550143035567)) ;
#22785=DIRECTION('ref_axis',(-0.976622827558554,-1.97668668594579E-6,0.214960118830513)) ;
#53877=CARTESIAN_POINT('',(0.,0.,0.)) ;
#53878=CARTESIAN_POINT('Origin',(-2.94971926719218E-15,-16.0575237924159,
0.)) ;
#53879=CARTESIAN_POINT('',(-1.27821691295437E-15,-16.2041857066289,-27.7395230264339)) ;
#53880=CARTESIAN_POINT('Origin',(-2.97666062376185E-15,-16.2041857066289,
0.)) ;
#53881=CARTESIAN_POINT('',(-8.3065322003863E-15,-15.9108618782029,-29.3077933083083)) ;
#53882=CARTESIAN_POINT('',(-8.1894302683888E-15,-16.0575237924159,-28.523658167371)) ;
#53883=CARTESIAN_POINT('',(-0.49246023091464,-15.9108618818334,-29.3036555873477)) ;
#53884=CARTESIAN_POINT('Origin',(-2.92277791062251E-15,-15.9108618782028,
0.)) ;
#53885=CARTESIAN_POINT('',(-2.30180707398644,-16.187744273641,-27.7320650306517)) ;
#53886=CARTESIAN_POINT('Ctrl Pts',(-0.49246024089823,-15.9108618853164,
-29.3036555618719)) ;
#53887=CARTESIAN_POINT('Ctrl Pts',(-0.524186138723702,-15.922600883412,
-29.2403504016751)) ;
#53888=CARTESIAN_POINT('Ctrl Pts',(-0.558017475224188,-15.9340937421157,
-29.178271027574)) ;
#53889=CARTESIAN_POINT('Ctrl Pts',(-0.593757701662899,-15.9452906232649,
-29.1176651035937)) ;
#53890=CARTESIAN_POINT('Ctrl Pts',(-0.606024695686751,-15.9491336899667,
-29.0968635424019)) ;
#53891=CARTESIAN_POINT('Ctrl Pts',(-0.618516201253947,-15.9529419398964,
-29.0762352962752)) ;
#53892=CARTESIAN_POINT('Ctrl Pts',(-0.631223168391001,-15.9567135267634,
-29.0557895107889)) ;
#53893=CARTESIAN_POINT('Ctrl Pts',(-0.667165886993807,-15.9673817754482,
-28.9979568976706)) ;
#53894=CARTESIAN_POINT('Ctrl Pts',(-0.704840463204382,-15.977757691291,
-28.9415784282644)) ;
#53895=CARTESIAN_POINT('Ctrl Pts',(-0.744004740092162,-15.9877997661731,
-28.8868614676232)) ;
#53896=CARTESIAN_POINT('Ctrl Pts',(-0.783488107070585,-15.997923658641,
-28.8316987017401)) ;
#53897=CARTESIAN_POINT('Ctrl Pts',(-0.824485149876229,-16.0077081692745,
-28.778224943148)) ;
#53898=CARTESIAN_POINT('Ctrl Pts',(-0.866713327822006,-16.0171189356806,
-28.7266128516104)) ;
#53899=CARTESIAN_POINT('Ctrl Pts',(-0.901270087053801,-16.0248200870137,
-28.6843769156199)) ;
#53900=CARTESIAN_POINT('Ctrl Pts',(-0.936650542924225,-16.0322710948775,
-28.6433869753027)) ;
#53901=CARTESIAN_POINT('Ctrl Pts',(-0.972685940156585,-16.0394576303854,
-28.6037161955719)) ;
#53902=CARTESIAN_POINT('Ctrl Pts',(-1.01677654000943,-16.0482506141109,
-28.5551775749572)) ;
#53903=CARTESIAN_POINT('Ctrl Pts',(-1.06297919541555,-16.0568730319549,
-28.5073700699597)) ;
#53904=CARTESIAN_POINT('Ctrl Pts',(-1.11118837792726,-16.0652608298865,
-28.4606078955835)) ;
#53905=CARTESIAN_POINT('Ctrl Pts',(-1.15900238541565,-16.073579872281,-28.4142290349743)) ;
#53906=CARTESIAN_POINT('Ctrl Pts',(-1.20878996696043,-16.081668020051,-28.3688788822698)) ;
#53907=CARTESIAN_POINT('Ctrl Pts',(-1.26040263359772,-16.0894673869311,
-28.3248412518989)) ;
#53908=CARTESIAN_POINT('Ctrl Pts',(-1.30281303157267,-16.0958761674669,
-28.2886553008216)) ;
#53909=CARTESIAN_POINT('Ctrl Pts',(-1.34645482892762,-16.1020900207685,
-28.2533552584702)) ;
#53910=CARTESIAN_POINT('Ctrl Pts',(-1.39122398593242,-16.108079933754,-28.2190838414456)) ;
#53911=CARTESIAN_POINT('Ctrl Pts',(-1.44727760151981,-16.1155796568301,
-28.17617401325)) ;
#53912=CARTESIAN_POINT('Ctrl Pts',(-1.50510762653917,-16.1227292229207,
-28.1348712493097)) ;
#53913=CARTESIAN_POINT('Ctrl Pts',(-1.56449742296339,-16.1294814162036,
-28.0954072564998)) ;
#53914=CARTESIAN_POINT('Ctrl Pts',(-1.62376979496718,-16.1362202591733,
-28.0560212911755)) ;
#53915=CARTESIAN_POINT('Ctrl Pts',(-1.68459540193731,-16.1425632136358,
-28.0184671715736)) ;
#53916=CARTESIAN_POINT('Ctrl Pts',(-1.74672461632394,-16.148471764915,-27.9829371559304)) ;
#53917=CARTESIAN_POINT('Ctrl Pts',(-1.79357965334542,-16.1529277264407,
-27.9561420287946)) ;
#53918=CARTESIAN_POINT('Ctrl Pts',(-1.84117536584348,-16.1571367885211,
-27.9304973511167)) ;
#53919=CARTESIAN_POINT('Ctrl Pts',(-1.88939385278889,-16.1610860188908,
-27.9060696007688)) ;
#53920=CARTESIAN_POINT('Ctrl Pts',(-1.95609837828205,-16.1665493080681,
-27.8722767217499)) ;
#53921=CARTESIAN_POINT('Ctrl Pts',(-2.02404088075897,-16.171518536629,-27.8407920493046)) ;
#53922=CARTESIAN_POINT('Ctrl Pts',(-2.09289039826686,-16.175968006779,-27.8117544103004)) ;
#53923=CARTESIAN_POINT('Ctrl Pts',(-2.16173991573683,-16.1804174769265,
-27.7827167713122)) ;
#53924=CARTESIAN_POINT('Ctrl Pts',(-2.23149584064641,-16.184347145014,-27.7561263494921)) ;
#53925=CARTESIAN_POINT('Ctrl Pts',(-2.30180707408357,-16.1877442734702,
-27.7320650305882)) ;
#53926=CARTESIAN_POINT('',(-2.44332709960924,-15.9108618782028,-29.2057682879055)) ;
#53927=CARTESIAN_POINT('Ctrl Pts',(-2.44332709960925,-15.9108618782028,
-29.2057682879055)) ;
#53928=CARTESIAN_POINT('Ctrl Pts',(-2.37152999340033,-16.0510971574587,
-28.4593807438797)) ;
#53929=CARTESIAN_POINT('Ctrl Pts',(-2.30180707378936,-16.1877442737199,
-27.7320650307343)) ;
#53930=CARTESIAN_POINT('',(-3.89217339575026,-15.9108618782028,-29.0481967574568)) ;
#53931=CARTESIAN_POINT('Origin',(-2.92277791062251E-15,-15.9108618782028,
0.)) ;
#53932=CARTESIAN_POINT('',(-3.71358212386582,-16.187744273641,-27.578525241199)) ;
#53933=CARTESIAN_POINT('Ctrl Pts',(-3.71358212407606,-16.1877442737199,
-27.5785252412373)) ;
#53934=CARTESIAN_POINT('Ctrl Pts',(-3.80184066656078,-16.0510971575306,
-28.3038250835262)) ;
#53935=CARTESIAN_POINT('Ctrl Pts',(-3.89217339575026,-15.9108618782028,
-29.0481967574569)) ;
#53936=CARTESIAN_POINT('',(-5.81847295702336,-15.9108618818334,-28.7244167966786)) ;
#53937=CARTESIAN_POINT('Ctrl Pts',(-3.71358212375731,-16.1877442734702,
-27.5785252411579)) ;
#53938=CARTESIAN_POINT('Ctrl Pts',(-3.78742199194626,-16.1843471450141,
-27.5869091829932)) ;
#53939=CARTESIAN_POINT('Ctrl Pts',(-3.86126321677957,-16.1804174769265,
-27.5978824736425)) ;
#53940=CARTESIAN_POINT('Ctrl Pts',(-3.93474530482747,-16.175968006779,-27.6114406176889)) ;
#53941=CARTESIAN_POINT('Ctrl Pts',(-4.00822739291584,-16.1715185366291,
-27.6249987617427)) ;
#53942=CARTESIAN_POINT('Ctrl Pts',(-4.08134971133666,-16.166549308068,-27.6411417103761)) ;
#53943=CARTESIAN_POINT('Ctrl Pts',(-4.15375919217085,-16.1610860188908,
-27.6598050294532)) ;
#53944=CARTESIAN_POINT('Ctrl Pts',(-4.22313933618834,-16.155851292919,-27.6776875463626)) ;
#53945=CARTESIAN_POINT('Ctrl Pts',(-4.29190989303592,-16.1501596984485,
-27.6978951324919)) ;
#53946=CARTESIAN_POINT('Ctrl Pts',(-4.35977148811458,-16.1440425621065,
-27.7203296643783)) ;
#53947=CARTESIAN_POINT('Ctrl Pts',(-4.42777328397754,-16.1379127878753,
-27.7428105455873)) ;
#53948=CARTESIAN_POINT('Ctrl Pts',(-4.49486188205611,-16.1313557844548,
-27.7675273949414)) ;
#53949=CARTESIAN_POINT('Ctrl Pts',(-4.5607563501789,-16.1244124680043,-27.7943340449523)) ;
#53950=CARTESIAN_POINT('Ctrl Pts',(-4.61040891985226,-16.1191805644221,
-27.8145332983235)) ;
#53951=CARTESIAN_POINT('Ctrl Pts',(-4.6593838589112,-16.1137295207043,-27.8359181045309)) ;
#53952=CARTESIAN_POINT('Ctrl Pts',(-4.7075709334888,-16.1080799337539,-27.8584093755501)) ;
#53953=CARTESIAN_POINT('Ctrl Pts',(-4.76966295670377,-16.1008000918637,
-27.8873907680604)) ;
#53954=CARTESIAN_POINT('Ctrl Pts',(-4.83045442176362,-16.0931892946344,
-27.9182150248434)) ;
#53955=CARTESIAN_POINT('Ctrl Pts',(-4.88971084783703,-16.085300212968,-27.9506685948721)) ;
#53956=CARTESIAN_POINT('Ctrl Pts',(-4.94945047354874,-16.0773468007022,
-27.9833868037652)) ;
#53957=CARTESIAN_POINT('Ctrl Pts',(-5.00762956373555,-16.0691106491232,
-28.0177606545818)) ;
#53958=CARTESIAN_POINT('Ctrl Pts',(-5.06404484329238,-16.060651803057,-28.0535335007289)) ;
#53959=CARTESIAN_POINT('Ctrl Pts',(-5.110245354077,-16.0537245483846,-28.082829176957)) ;
#53960=CARTESIAN_POINT('Ctrl Pts',(-5.15526359580896,-16.0466480826282,
-28.1130622837498)) ;
#53961=CARTESIAN_POINT('Ctrl Pts',(-5.19900837882609,-16.0394576303854,
-28.1440759310355)) ;
#53962=CARTESIAN_POINT('Ctrl Pts',(-5.25251261681066,-16.0306629892538,
-28.1820087186892)) ;
#53963=CARTESIAN_POINT('Ctrl Pts',(-5.30548320190949,-16.0214720150689,
-28.2220830974099)) ;
#53964=CARTESIAN_POINT('Ctrl Pts',(-5.35759068651864,-16.0119118209665,
-28.2642301528485)) ;
#53965=CARTESIAN_POINT('Ctrl Pts',(-5.40927139607099,-16.0024299275614,
-28.3060320119662)) ;
#53966=CARTESIAN_POINT('Ctrl Pts',(-5.46010261316689,-15.9925848997548,
-28.3498725976557)) ;
#53967=CARTESIAN_POINT('Ctrl Pts',(-5.50978147538154,-15.9824119250018,
-28.3956378490517)) ;
#53968=CARTESIAN_POINT('Ctrl Pts',(-5.55057275114205,-15.9740589032143,
-28.4332156619629)) ;
#53969=CARTESIAN_POINT('Ctrl Pts',(-5.59058732671593,-15.965484957055,-28.4720901843792)) ;
#53970=CARTESIAN_POINT('Ctrl Pts',(-5.62967034032201,-15.9567135267634,
-28.5121756210024)) ;
#53971=CARTESIAN_POINT('Ctrl Pts',(-5.67863253635718,-15.9457249040903,
-28.5623936268574)) ;
#53972=CARTESIAN_POINT('Ctrl Pts',(-5.72613910993178,-15.9344245943246,
-28.6145204117879)) ;
#53973=CARTESIAN_POINT('Ctrl Pts',(-5.7719333306353,-15.9228603613917,-28.6683698779022)) ;
#53974=CARTESIAN_POINT('Ctrl Pts',(-5.78765112225729,-15.9188912098106,
-28.6868524434823)) ;
#53975=CARTESIAN_POINT('Ctrl Pts',(-5.8031674745876,-15.9148910209384,-28.7055376017322)) ;
#53976=CARTESIAN_POINT('Ctrl Pts',(-5.81847294179664,-15.9108618853164,
-28.7244167739446)) ;
#53977=CARTESIAN_POINT('',(-6.78036653080772,-15.9108618828344,-28.5126880007908)) ;
#53978=CARTESIAN_POINT('Origin',(-2.92277791062251E-15,-15.9108618782028,
0.)) ;
#53979=CARTESIAN_POINT('',(-8.20956633133313,-16.1877442736409,-26.5888842812482)) ;
#53980=CARTESIAN_POINT('Ctrl Pts',(-6.78036653281022,-15.9108618871751,
-28.5126879735306)) ;
#53981=CARTESIAN_POINT('Ctrl Pts',(-6.79774195886506,-15.9226008852454,
-28.4440427226535)) ;
#53982=CARTESIAN_POINT('Ctrl Pts',(-6.81743710737947,-15.9340937439209,
-28.3761419926111)) ;
#53983=CARTESIAN_POINT('Ctrl Pts',(-6.83931326525882,-15.9452906250393,
-28.3092699093489)) ;
#53984=CARTESIAN_POINT('Ctrl Pts',(-6.84682174193608,-15.9491336911389,
-28.2863176395625)) ;
#53985=CARTESIAN_POINT('Ctrl Pts',(-6.85458673873747,-15.9529419404769,
-28.2634863694506)) ;
#53986=CARTESIAN_POINT('Ctrl Pts',(-6.86260138330426,-15.9567135267634,
-28.2407869762416)) ;
#53987=CARTESIAN_POINT('Ctrl Pts',(-6.8852714788191,-15.9673817754481,-28.1765798354398)) ;
#53988=CARTESIAN_POINT('Ctrl Pts',(-6.90994553998719,-15.9777576912908,
-28.1134205430859)) ;
#53989=CARTESIAN_POINT('Ctrl Pts',(-6.93643164872909,-15.9877997661729,
-28.0515636727349)) ;
#53990=CARTESIAN_POINT('Ctrl Pts',(-6.96313355246351,-15.9979236586408,
-27.9892028248837)) ;
#53991=CARTESIAN_POINT('Ctrl Pts',(-6.99167682976634,-16.0077081692742,
-27.9281661007126)) ;
#53992=CARTESIAN_POINT('Ctrl Pts',(-7.02182266234008,-16.0171189356803,
-27.8686828611919)) ;
#53993=CARTESIAN_POINT('Ctrl Pts',(-7.04649202599232,-16.0248200870135,
-27.8200056961688)) ;
#53994=CARTESIAN_POINT('Ctrl Pts',(-7.07223368095194,-16.0322710948773,
-27.7723683257036)) ;
#53995=CARTESIAN_POINT('Ctrl Pts',(-7.09889854564042,-16.0394576303853,
-27.7258784815505)) ;
#53996=CARTESIAN_POINT('Ctrl Pts',(-7.13152396312936,-16.0482506141108,
-27.6689964912531)) ;
#53997=CARTESIAN_POINT('Ctrl Pts',(-7.16636922573244,-16.0568730319548,
-27.6123744939841)) ;
#53998=CARTESIAN_POINT('Ctrl Pts',(-7.20339881913625,-16.0652608298864,
-27.5563420440722)) ;
#53999=CARTESIAN_POINT('Ctrl Pts',(-7.24012487761836,-16.0735798722808,
-27.5007688972131)) ;
#54000=CARTESIAN_POINT('Ctrl Pts',(-7.27899951088328,-16.0816680200507,
-27.4457761475559)) ;
#54001=CARTESIAN_POINT('Ctrl Pts',(-7.31993871326926,-16.0894673869308,
-27.3916728948438)) ;
#54002=CARTESIAN_POINT('Ctrl Pts',(-7.35357866987537,-16.0958761674666,
-27.347215969271)) ;
#54003=CARTESIAN_POINT('Ctrl Pts',(-7.38861168061711,-16.1020900207684,
-27.3033595259035)) ;
#54004=CARTESIAN_POINT('Ctrl Pts',(-7.42496681800589,-16.1080799337539,
-27.2602653101741)) ;
#54005=CARTESIAN_POINT('Ctrl Pts',(-7.47048558655389,-16.1155796568301,
-27.206308819498)) ;
#54006=CARTESIAN_POINT('Ctrl Pts',(-7.51808470437888,-16.1227292229208,
-27.1535399452904)) ;
#54007=CARTESIAN_POINT('Ctrl Pts',(-7.56760240845947,-16.1294814162036,
-27.1022315480204)) ;
#54008=CARTESIAN_POINT('Ctrl Pts',(-7.61702220704024,-16.1362202591733,
-27.0510245967762)) ;
#54009=CARTESIAN_POINT('Ctrl Pts',(-7.66835271949838,-16.1425632136358,
-27.0012727641148)) ;
#54010=CARTESIAN_POINT('Ctrl Pts',(-7.72139148427502,-16.148471764915,-26.9532174759262)) ;
#54011=CARTESIAN_POINT('Ctrl Pts',(-7.76139091629272,-16.1529277264407,
-26.916976356038)) ;
#54012=CARTESIAN_POINT('Ctrl Pts',(-7.80236101983229,-16.1571367885211,
-26.8816995654055)) ;
#54013=CARTESIAN_POINT('Ctrl Pts',(-7.84420094110262,-16.1610860188908,
-26.8474773729212)) ;
#54014=CARTESIAN_POINT('Ctrl Pts',(-7.90208148177932,-16.166549308068,-26.8001350514255)) ;
#54015=CARTESIAN_POINT('Ctrl Pts',(-7.96166725240902,-16.171518536629,-26.7547808434592)) ;
#54016=CARTESIAN_POINT('Ctrl Pts',(-8.02266487241837,-16.1759680067789,
-26.7116214772316)) ;
#54017=CARTESIAN_POINT('Ctrl Pts',(-8.08366249239416,-16.1804174769265,
-26.6684621110276)) ;
#54018=CARTESIAN_POINT('Ctrl Pts',(-8.14607140785925,-16.184347145014,-26.6274978966081)) ;
#54019=CARTESIAN_POINT('Ctrl Pts',(-8.20956633141436,-16.1877442734702,
-26.5888842811653)) ;
#54020=CARTESIAN_POINT('',(-8.6645803353537,-15.9108618782028,-27.9977105530919)) ;
#54021=CARTESIAN_POINT('Ctrl Pts',(-8.66458033535307,-15.9108618782028,
-27.9977105530921)) ;
#54022=CARTESIAN_POINT('Ctrl Pts',(-8.43401054721174,-16.0510971571362,
-27.2842073922392)) ;
#54023=CARTESIAN_POINT('Ctrl Pts',(-8.20956633115848,-16.1877442737199,
-26.5888842813712)) ;
#54024=CARTESIAN_POINT('',(-10.0456801889648,-15.9108618782028,-27.5323638313813)) ;
#54025=CARTESIAN_POINT('Origin',(-2.92277791062251E-15,-15.9108618782028,
0.)) ;
#54026=CARTESIAN_POINT('',(-9.55532834895708,-16.187744273641,-26.1354442627972)) ;
#54027=CARTESIAN_POINT('Ctrl Pts',(-9.55532834917054,-16.1877442737199,
-26.1354442627894)) ;
#54028=CARTESIAN_POINT('Ctrl Pts',(-9.79744148403593,-16.0510971565844,
-26.8248140248655)) ;
#54029=CARTESIAN_POINT('Ctrl Pts',(-10.0456801889654,-15.9108618782028,
-27.5323638313811)) ;
#54030=CARTESIAN_POINT('',(-11.8573408058246,-15.9108618828344,-26.8020561960657)) ;
#54031=CARTESIAN_POINT('Ctrl Pts',(-9.55532834884232,-16.1877442734702,
-26.1354442627804)) ;
#54032=CARTESIAN_POINT('Ctrl Pts',(-9.62924418161346,-16.184347145014,-26.1277588037449)) ;
#54033=CARTESIAN_POINT('Ctrl Pts',(-9.70371797276582,-16.1804174769265,
-26.1226018643487)) ;
#54034=CARTESIAN_POINT('Ctrl Pts',(-9.77839669062387,-16.1759680067789,
-26.1200465497064)) ;
#54035=CARTESIAN_POINT('Ctrl Pts',(-9.85307540852301,-16.1715185366289,
-26.1174912350626)) ;
#54036=CARTESIAN_POINT('Ctrl Pts',(-9.92795842454781,-16.166549308068,-26.1175376335476)) ;
#54037=CARTESIAN_POINT('Ctrl Pts',(-10.0026870738764,-16.1610860188908,
-26.1201987166258)) ;
#54038=CARTESIAN_POINT('Ctrl Pts',(-10.0742893612143,-16.155851292919,-26.1227484701259)) ;
#54039=CARTESIAN_POINT('Ctrl Pts',(-10.1457961343455,-16.1501596984485,
-26.1276999772421)) ;
#54040=CARTESIAN_POINT('Ctrl Pts',(-10.2168939242383,-16.1440425621064,
-26.1350217652726)) ;
#54041=CARTESIAN_POINT('Ctrl Pts',(-10.2881386008333,-16.1379127878752,
-26.1423586799801)) ;
#54042=CARTESIAN_POINT('Ctrl Pts',(-10.3589720967571,-16.1313557844547,
-26.1520755976696)) ;
#54043=CARTESIAN_POINT('Ctrl Pts',(-10.4290886261871,-16.1244124680042,
-26.1640901602802)) ;
#54044=CARTESIAN_POINT('Ctrl Pts',(-10.4819225887626,-16.119180564422,-26.1731433315722)) ;
#54045=CARTESIAN_POINT('Ctrl Pts',(-10.534349622166,-16.1137295207043,-26.1835000086853)) ;
#54046=CARTESIAN_POINT('Ctrl Pts',(-10.5862450681494,-16.108079933754,-26.1951066496522)) ;
#54047=CARTESIAN_POINT('Ctrl Pts',(-10.6531155570727,-16.1008000918637,
-26.2100625237468)) ;
#54048=CARTESIAN_POINT('Ctrl Pts',(-10.7191120555118,-16.0931892946344,
-26.2270977585306)) ;
#54049=CARTESIAN_POINT('Ctrl Pts',(-10.7839596575085,-16.085300212968,-26.2460542021285)) ;
#54050=CARTESIAN_POINT('Ctrl Pts',(-10.8493360517377,-16.0773468007022,
-26.2651652238421)) ;
#54051=CARTESIAN_POINT('Ctrl Pts',(-10.9135443089684,-16.0691106491231,
-26.2862286485001)) ;
#54052=CARTESIAN_POINT('Ctrl Pts',(-10.9763307351236,-16.0606518030569,
-26.3090375279026)) ;
#54053=CARTESIAN_POINT('Ctrl Pts',(-11.0277488080551,-16.0537245483846,
-26.327716543359)) ;
#54054=CARTESIAN_POINT('Ctrl Pts',(-11.0782137725886,-16.0466480826281,
-26.3475652256732)) ;
#54055=CARTESIAN_POINT('Ctrl Pts',(-11.1276028442977,-16.0394576303853,
-26.3684499558578)) ;
#54056=CARTESIAN_POINT('Ctrl Pts',(-11.1880106109912,-16.0306629892538,
-26.393994066423)) ;
#54057=CARTESIAN_POINT('Ctrl Pts',(-11.2483575800814,-16.0214720150689,
-26.421744418442)) ;
#54058=CARTESIAN_POINT('Ctrl Pts',(-11.3083071917182,-16.0119118209665,
-26.4517045302412)) ;
#54059=CARTESIAN_POINT('Ctrl Pts',(-11.3677657990569,-16.0024299275615,
-26.4814192602395)) ;
#54060=CARTESIAN_POINT('Ctrl Pts',(-11.4268330405492,-15.9925848997549,
-26.5133076682826)) ;
#54061=CARTESIAN_POINT('Ctrl Pts',(-11.4851886148112,-15.9824119250019,
-26.5473234666537)) ;
#54062=CARTESIAN_POINT('Ctrl Pts',(-11.5331043321964,-15.9740589032144,
-26.5752538126744)) ;
#54063=CARTESIAN_POINT('Ctrl Pts',(-11.5805402624269,-15.965484957055,-26.6046175194338)) ;
#54064=CARTESIAN_POINT('Ctrl Pts',(-11.6273267208508,-15.9567135267634,
-26.635364088185)) ;
#54065=CARTESIAN_POINT('Ctrl Pts',(-11.685939594779,-15.9457249040899,-26.673882600136)) ;
#54066=CARTESIAN_POINT('Ctrl Pts',(-11.743541208969,-15.9344245943236,-26.7145781807697)) ;
#54067=CARTESIAN_POINT('Ctrl Pts',(-11.7998408296788,-15.9228603613902,
-26.7573242725093)) ;
#54068=CARTESIAN_POINT('Ctrl Pts',(-11.8191643503523,-15.91889121042,-26.7719958631351)) ;
#54069=CARTESIAN_POINT('Ctrl Pts',(-11.8383346927553,-15.9148910221682,
-26.7869086133455)) ;
#54070=CARTESIAN_POINT('Ctrl Pts',(-11.8573407877332,-15.9108618871751,
-26.802056175576)) ;
#54071=CARTESIAN_POINT('',(-12.751230463362,-15.9108618962294,-26.3884985273164)) ;
#54072=CARTESIAN_POINT('Origin',(-2.92277791062251E-15,-15.9108618782028,
0.)) ;
#54073=CARTESIAN_POINT('',(-13.733455391304,-16.1877442736409,-24.2024368542766)) ;
#54074=CARTESIAN_POINT('Ctrl Pts',(-12.7512304249355,-15.9108619321403,
-26.3884985240484)) ;
#54075=CARTESIAN_POINT('Ctrl Pts',(-12.7534429295709,-15.9226009295965,
-26.317722958503)) ;
#54076=CARTESIAN_POINT('Ctrl Pts',(-12.7580809727586,-15.9340937875902,
-26.2471758359495)) ;
#54077=CARTESIAN_POINT('Ctrl Pts',(-12.7650701630532,-15.9452906679662,
-26.1771644588304)) ;
#54078=CARTESIAN_POINT('Ctrl Pts',(-12.7674690293055,-15.9491337194976,
-26.1531347897597)) ;
#54079=CARTESIAN_POINT('Ctrl Pts',(-12.7701444276626,-15.9529419545197,
-26.1291681467903)) ;
#54080=CARTESIAN_POINT('Ctrl Pts',(-12.7730919847679,-15.9567135267634,
-26.1052766300655)) ;
#54081=CARTESIAN_POINT('Ctrl Pts',(-12.7814294287248,-15.9673817754482,
-26.0376972161225)) ;
#54082=CARTESIAN_POINT('Ctrl Pts',(-12.7919492431736,-15.9777576912909,
-25.9707103591345)) ;
#54083=CARTESIAN_POINT('Ctrl Pts',(-12.8045187227623,-15.987799766173,-25.904605937582)) ;
#54084=CARTESIAN_POINT('Ctrl Pts',(-12.8171906119115,-15.9979236586409,
-25.8379629316985)) ;
#54085=CARTESIAN_POINT('Ctrl Pts',(-12.8319454717887,-16.0077081692743,
-25.7722172513329)) ;
#54086=CARTESIAN_POINT('Ctrl Pts',(-12.8485993733643,-16.0171189356803,
-25.7076442339976)) ;
#54087=CARTESIAN_POINT('Ctrl Pts',(-12.8622278294101,-16.0248200870135,
-25.6548019300786)) ;
#54088=CARTESIAN_POINT('Ctrl Pts',(-12.8771270322822,-16.0322710948774,
-25.6027445999641)) ;
#54089=CARTESIAN_POINT('Ctrl Pts',(-12.8931745449892,-16.0394576303854,
-25.5516095048324)) ;
#54090=CARTESIAN_POINT('Ctrl Pts',(-12.9128092518532,-16.0482506141109,
-25.4890438834985)) ;
#54091=CARTESIAN_POINT('Ctrl Pts',(-12.934667795902,-16.0568730319549,-25.4262549756191)) ;
#54092=CARTESIAN_POINT('Ctrl Pts',(-12.9587863375661,-16.0652608298865,
-25.3635722652533)) ;
#54093=CARTESIAN_POINT('Ctrl Pts',(-12.9827071773659,-16.0735798722809,
-25.3014033707258)) ;
#54094=CARTESIAN_POINT('Ctrl Pts',(-13.008851127706,-16.0816680200508,-25.2393394239693)) ;
#54095=CARTESIAN_POINT('Ctrl Pts',(-13.0372025942384,-16.089467386931,-25.1777003568806)) ;
#54096=CARTESIAN_POINT('Ctrl Pts',(-13.0604991424922,-16.0958761674668,
-25.1270512132426)) ;
#54097=CARTESIAN_POINT('Ctrl Pts',(-13.0852852619739,-16.1020900207685,
-25.0766890474091)) ;
#54098=CARTESIAN_POINT('Ctrl Pts',(-13.1115264539273,-16.108079933754,-25.0267870706076)) ;
#54099=CARTESIAN_POINT('Ctrl Pts',(-13.1443819684093,-16.1155796568302,
-24.9643068629862)) ;
#54100=CARTESIAN_POINT('Ctrl Pts',(-13.1795244971934,-16.1227292229209,
-24.9025392924203)) ;
#54101=CARTESIAN_POINT('Ctrl Pts',(-13.2168547161228,-16.1294814162038,
-24.8417856143209)) ;
#54102=CARTESIAN_POINT('Ctrl Pts',(-13.2541111264253,-16.1362202591735,
-24.7811520572841)) ;
#54103=CARTESIAN_POINT('Ctrl Pts',(-13.2935463866587,-16.142563213636,-24.7215288519631)) ;
#54104=CARTESIAN_POINT('Ctrl Pts',(-13.335014668133,-16.1484717649152,-24.663195303095)) ;
#54105=CARTESIAN_POINT('Ctrl Pts',(-13.3662881661615,-16.1529277264408,
-24.6192027849421)) ;
#54106=CARTESIAN_POINT('Ctrl Pts',(-13.3987169442358,-16.1571367885212,
-24.5759433848783)) ;
#54107=CARTESIAN_POINT('Ctrl Pts',(-13.4322219116137,-16.1610860188908,
-24.5335269419437)) ;
#54108=CARTESIAN_POINT('Ctrl Pts',(-13.4785720377214,-16.166549308068,-24.4748488523074)) ;
#54109=CARTESIAN_POINT('Ctrl Pts',(-13.5270149120941,-16.171518536629,-24.4177458211771)) ;
#54110=CARTESIAN_POINT('Ctrl Pts',(-13.5773084536872,-16.1759680067789,
-24.3624828117227)) ;
#54111=CARTESIAN_POINT('Ctrl Pts',(-13.6276019952526,-16.1804174769264,
-24.3072198022987)) ;
#54112=CARTESIAN_POINT('Ctrl Pts',(-13.6797457297486,-16.1843471450139,
-24.2537972364176)) ;
#54113=CARTESIAN_POINT('Ctrl Pts',(-13.7334553913656,-16.1877442734701,
-24.2024368541783)) ;
#54114=CARTESIAN_POINT('',(-14.4806874246056,-15.9108618782028,-25.4805109900367)) ;
#54115=CARTESIAN_POINT('Ctrl Pts',(-14.4806874246052,-15.9108618782028,
-25.480510990037)) ;
#54116=CARTESIAN_POINT('Ctrl Pts',(-14.1021261398189,-16.0510971577221,
-24.8332548227359)) ;
#54117=CARTESIAN_POINT('Ctrl Pts',(-13.7334553911596,-16.1877442737198,
-24.2024368544343)) ;
#54118=CARTESIAN_POINT('',(-15.7294621415161,-15.9108618782028,-24.7291481725741)) ;
#54119=CARTESIAN_POINT('Origin',(-2.92277791062251E-15,-15.9108618782028,
0.)) ;
#54120=CARTESIAN_POINT('',(-14.9502780404369,-16.1877442736409,-23.4702989581261)) ;
#54121=CARTESIAN_POINT('Ctrl Pts',(-14.9502780406439,-16.1877442737198,
-23.4702989580725)) ;
#54122=CARTESIAN_POINT('Ctrl Pts',(-15.334924823484,-16.051097157543,-24.0915044666593)) ;
#54123=CARTESIAN_POINT('Ctrl Pts',(-15.7294621415166,-15.9108618782028,
-24.7291481725738)) ;
#54124=CARTESIAN_POINT('',(-17.3417723053831,-15.9108618962294,-23.6264611434764)) ;
#54125=CARTESIAN_POINT('Ctrl Pts',(-14.9502780403211,-16.1877442734701,
-23.4702989581345)) ;
#54126=CARTESIAN_POINT('Ctrl Pts',(-15.0208136154855,-16.1843471450139,
-23.4469034617511)) ;
#54127=CARTESIAN_POINT('Ctrl Pts',(-15.0924376612541,-16.1804174769263,
-23.4258574250642)) ;
#54128=CARTESIAN_POINT('Ctrl Pts',(-15.1648211150744,-16.1759680067789,
-23.4073081354059)) ;
#54129=CARTESIAN_POINT('Ctrl Pts',(-15.2372045689347,-16.171518536629,-23.3887588457375)) ;
#54130=CARTESIAN_POINT('Ctrl Pts',(-15.3103468359606,-16.166549308068,-23.3727065245325)) ;
#54131=CARTESIAN_POINT('Ctrl Pts',(-15.3839004251958,-16.1610860188908,
-23.3592409423246)) ;
#54132=CARTESIAN_POINT('Ctrl Pts',(-15.4543768124774,-16.155851292919,-23.3463387087759)) ;
#54133=CARTESIAN_POINT('Ctrl Pts',(-15.5252762246533,-16.1501596984486,
-23.3358026099092)) ;
#54134=CARTESIAN_POINT('Ctrl Pts',(-15.5962857557236,-16.1440425621066,
-23.3276692954131)) ;
#54135=CARTESIAN_POINT('Ctrl Pts',(-15.6674419911549,-16.1379127878755,
-23.3195191776417)) ;
#54136=CARTESIAN_POINT('Ctrl Pts',(-15.7387082893792,-16.1313557844551,
-23.3137818113949)) ;
#54137=CARTESIAN_POINT('Ctrl Pts',(-15.8097683091281,-16.1244124680047,
-23.3104424990107)) ;
#54138=CARTESIAN_POINT('Ctrl Pts',(-15.8633132072386,-16.1191805644224,
-23.3079262719957)) ;
#54139=CARTESIAN_POINT('Ctrl Pts',(-15.9167409051749,-16.1137295207044,
-23.3067705533035)) ;
#54140=CARTESIAN_POINT('Ctrl Pts',(-15.9699181491897,-16.1080799337539,
-23.3069498505864)) ;
#54141=CARTESIAN_POINT('Ctrl Pts',(-16.0384403140804,-16.1008000918637,
-23.3071808862148)) ;
#54142=CARTESIAN_POINT('Ctrl Pts',(-16.1065559229815,-16.0931892946344,
-23.3096305503542)) ;
#54143=CARTESIAN_POINT('Ctrl Pts',(-16.173962499105,-16.085300212968,-23.3142034852872)) ;
#54144=CARTESIAN_POINT('Ctrl Pts',(-16.2419187343181,-16.0773468007022,
-23.3188137096865)) ;
#54145=CARTESIAN_POINT('Ctrl Pts',(-16.3091538518471,-16.0691106491231,
-23.3255818058591)) ;
#54146=CARTESIAN_POINT('Ctrl Pts',(-16.3753756010958,-16.0606518030569,
-23.3343602006664)) ;
#54147=CARTESIAN_POINT('Ctrl Pts',(-16.429606984231,-16.0537245483846,-23.3415491453487)) ;
#54148=CARTESIAN_POINT('Ctrl Pts',(-16.4831589859123,-16.0466480826281,
-23.3500853008595)) ;
#54149=CARTESIAN_POINT('Ctrl Pts',(-16.5358829682123,-16.0394576303854,
-23.3598645671713)) ;
#54150=CARTESIAN_POINT('Ctrl Pts',(-16.6003696635835,-16.0306629892537,
-23.3718255864285)) ;
#54151=CARTESIAN_POINT('Ctrl Pts',(-16.6652712594621,-16.0214720150687,
-23.3859543361279)) ;
#54152=CARTESIAN_POINT('Ctrl Pts',(-16.7302598209164,-16.0119118209662,
-23.4023266027586)) ;
#54153=CARTESIAN_POINT('Ctrl Pts',(-16.7947161076464,-16.002429927561,-23.4185647758886)) ;
#54154=CARTESIAN_POINT('Ctrl Pts',(-16.8592574549723,-15.9925848997543,
-23.437009939767)) ;
#54155=CARTESIAN_POINT('Ctrl Pts',(-16.9235610994876,-15.9824119250012,
-23.4576857441875)) ;
#54156=CARTESIAN_POINT('Ctrl Pts',(-16.9763607728054,-15.9740589032139,
-23.4746626313798)) ;
#54157=CARTESIAN_POINT('Ctrl Pts',(-17.0290000063144,-15.9654849570548,
-23.4931425081888)) ;
#54158=CARTESIAN_POINT('Ctrl Pts',(-17.081302226758,-15.9567135267635,-23.513112533685)) ;
#54159=CARTESIAN_POINT('Ctrl Pts',(-17.1468251058111,-15.9457249040773,
-23.53813046895)) ;
#54160=CARTESIAN_POINT('Ctrl Pts',(-17.2118283732285,-15.9344245942977,
-23.5654919651982)) ;
#54161=CARTESIAN_POINT('Ctrl Pts',(-17.2760008863226,-15.9228603613504,
-23.5951359228588)) ;
#54162=CARTESIAN_POINT('Ctrl Pts',(-17.2980265101066,-15.9188912251585,
-23.6053104762216)) ;
#54163=CARTESIAN_POINT('Ctrl Pts',(-17.3199543797531,-15.9148910519162,
-23.6157534777929)) ;
#54164=CARTESIAN_POINT('Ctrl Pts',(-17.341772320495,-15.9108619321403,-23.6264611079952)) ;
#54165=CARTESIAN_POINT('',(-18.1258609279822,-15.9108618949459,-23.0304124971064)) ;
#54166=CARTESIAN_POINT('Origin',(-2.92277791062251E-15,-15.9108618782028,
0.)) ;
#54167=CARTESIAN_POINT('',(-18.6151833408184,-16.1877442736409,-20.6843103790748)) ;
#54168=CARTESIAN_POINT('Ctrl Pts',(-18.125860892512,-15.9108619279123,-23.0304125002963)) ;
#54169=CARTESIAN_POINT('Ctrl Pts',(-18.1128070149588,-15.9226009254264,
-22.9608160051258)) ;
#54170=CARTESIAN_POINT('Ctrl Pts',(-18.1021710767023,-15.9340937834842,
-22.8909211929491)) ;
#54171=CARTESIAN_POINT('Ctrl Pts',(-18.0939464864751,-15.9452906639301,
-22.8210441736094)) ;
#54172=CARTESIAN_POINT('Ctrl Pts',(-18.0911235988425,-15.9491337168313,
-22.7970606111163)) ;
#54173=CARTESIAN_POINT('Ctrl Pts',(-18.0885843270955,-15.9529419531994,
-22.7730791549778)) ;
#54174=CARTESIAN_POINT('Ctrl Pts',(-18.0863270012958,-15.9567135267635,
-22.7491125625987)) ;
#54175=CARTESIAN_POINT('Ctrl Pts',(-18.0799419440817,-15.9673817754481,
-22.6813208138021)) ;
#54176=CARTESIAN_POINT('Ctrl Pts',(-18.0758156169796,-15.9777576912907,
-22.6136386231626)) ;
#54177=CARTESIAN_POINT('Ctrl Pts',(-18.0738807325195,-15.9877997661727,
-22.5463776196913)) ;
#54178=CARTESIAN_POINT('Ctrl Pts',(-18.0719300836305,-15.9979236586405,
-22.478568608663)) ;
#54179=CARTESIAN_POINT('Ctrl Pts',(-18.0722066052329,-16.0077081692739,
-22.4111881670463)) ;
#54180=CARTESIAN_POINT('Ctrl Pts',(-18.0745898578821,-16.0171189356799,
-22.3445447344199)) ;
#54181=CARTESIAN_POINT('Ctrl Pts',(-18.0765401548637,-16.0248200870132,
-22.2900081390048)) ;
#54182=CARTESIAN_POINT('Ctrl Pts',(-18.0799002354814,-16.0322710948773,
-22.2359649921384)) ;
#54183=CARTESIAN_POINT('Ctrl Pts',(-18.0845800323485,-16.0394576303854,
-22.1825756662427)) ;
#54184=CARTESIAN_POINT('Ctrl Pts',(-18.090305931517,-16.0482506141108,-22.1172519127896)) ;
#54185=CARTESIAN_POINT('Ctrl Pts',(-18.0981556757857,-16.0568730319548,
-22.0512320338478)) ;
#54186=CARTESIAN_POINT('Ctrl Pts',(-18.1082354095076,-16.0652608298863,
-21.9848300368986)) ;
#54187=CARTESIAN_POINT('Ctrl Pts',(-18.1182325187418,-16.0735798722807,
-21.9189723431157)) ;
#54188=CARTESIAN_POINT('Ctrl Pts',(-18.1304233240958,-16.0816680200506,
-21.8527392404316)) ;
#54189=CARTESIAN_POINT('Ctrl Pts',(-18.1448613717095,-16.0894673869308,
-21.7864465332374)) ;
#54190=CARTESIAN_POINT('Ctrl Pts',(-18.1567251909072,-16.0958761674667,
-21.7319734691972)) ;
#54191=CARTESIAN_POINT('Ctrl Pts',(-18.1701054477303,-16.1020900207684,
-21.6774604597971)) ;
#54192=CARTESIAN_POINT('Ctrl Pts',(-18.1850056852781,-16.108079933754,-21.6230840828955)) ;
#54193=CARTESIAN_POINT('Ctrl Pts',(-18.2036616583526,-16.1155796568301,
-21.5550016633967)) ;
#54194=CARTESIAN_POINT('Ctrl Pts',(-18.2247043725071,-16.1227292229207,
-21.4871235794238)) ;
#54195=CARTESIAN_POINT('Ctrl Pts',(-18.2481015867369,-16.1294814162035,
-21.4197653949614)) ;
#54196=CARTESIAN_POINT('Ctrl Pts',(-18.2714525404223,-16.1362202591732,
-21.3525403898704)) ;
#54197=CARTESIAN_POINT('Ctrl Pts',(-18.2971485994912,-16.1425632136357,
-21.2858337267049)) ;
#54198=CARTESIAN_POINT('Ctrl Pts',(-18.3251073869094,-16.1484717649149,
-21.2199495290698)) ;
#54199=CARTESIAN_POINT('Ctrl Pts',(-18.3461926369402,-16.1529277264406,
-21.1702626539049)) ;
#54200=CARTESIAN_POINT('Ctrl Pts',(-18.3685637559296,-16.1571367885211,
-21.1210434058756)) ;
#54201=CARTESIAN_POINT('Ctrl Pts',(-18.39216711438,-16.1610860188908,-21.0724160582178)) ;
#54202=CARTESIAN_POINT('Ctrl Pts',(-18.4248195455367,-16.166549308068,-21.0051459226958)) ;
#54203=CARTESIAN_POINT('Ctrl Pts',(-18.4598543886873,-16.171518536629,-20.9389641426716)) ;
#54204=CARTESIAN_POINT('Ctrl Pts',(-18.4970921817568,-16.1759680067789,
-20.8741815268919)) ;
#54205=CARTESIAN_POINT('Ctrl Pts',(-18.5343299748059,-16.1804174769264,
-20.809398911148)) ;
#54206=CARTESIAN_POINT('Ctrl Pts',(-18.5737703452613,-16.1843471450139,
-20.746015973611)) ;
#54207=CARTESIAN_POINT('Ctrl Pts',(-18.6151833408574,-16.1877442734701,
-20.6843103789655)) ;
#54208=CARTESIAN_POINT('',(-19.6196936640125,-15.9108618782028,-21.7718710526408)) ;
#54209=CARTESIAN_POINT('Ctrl Pts',(-19.6196936640131,-15.9108618782028,
-21.7718710526403)) ;
#54210=CARTESIAN_POINT('Ctrl Pts',(-19.1108419877152,-16.051097157933,-21.2211268600534)) ;
#54211=CARTESIAN_POINT('Ctrl Pts',(-18.6151833407114,-16.1877442737198,
-20.6843103792598)) ;
#54212=CARTESIAN_POINT('',(-20.67775192637,-15.9108618782028,-20.7696250296921)) ;
#54213=CARTESIAN_POINT('Origin',(-2.92277791062251E-15,-15.9108618782028,
0.)) ;
#54214=CARTESIAN_POINT('',(-19.6461693467843,-16.1877442736409,-19.7077085595372)) ;
#54215=CARTESIAN_POINT('Ctrl Pts',(-19.6461693469749,-16.1877442737198,
-19.7077085594403)) ;
#54216=CARTESIAN_POINT('Ctrl Pts',(-20.1553641225658,-16.0510971577741,
-20.2317029393282)) ;
#54217=CARTESIAN_POINT('Ctrl Pts',(-20.6777519263695,-15.9108618782028,
-20.7696250296926)) ;
#54218=CARTESIAN_POINT('',(-22.0153220853232,-15.9108618949459,-19.3461191882741)) ;
#54219=CARTESIAN_POINT('Ctrl Pts',(-19.646169346673,-16.1877442734701,-19.7077085595702)) ;
#54220=CARTESIAN_POINT('Ctrl Pts',(-19.710026499131,-16.1843471450139,-19.6696969732475)) ;
#54221=CARTESIAN_POINT('Ctrl Pts',(-19.7754517387404,-16.1804174769264,
-19.6337459285543)) ;
#54222=CARTESIAN_POINT('Ctrl Pts',(-19.8421553586713,-16.1759680067789,
-19.6000700080484)) ;
#54223=CARTESIAN_POINT('Ctrl Pts',(-19.9088589786389,-16.171518536629,-19.5663940875241)) ;
#54224=CARTESIAN_POINT('Ctrl Pts',(-19.9768404455518,-16.166549308068,-19.5349936353279)) ;
#54225=CARTESIAN_POINT('Ctrl Pts',(-20.0457796906103,-16.1610860188908,
-19.506031023492)) ;
#54226=CARTESIAN_POINT('Ctrl Pts',(-20.1118347802969,-16.155851292919,-19.4782800969949)) ;
#54227=CARTESIAN_POINT('Ctrl Pts',(-20.178811653805,-16.1501596984485,-19.4527490484184)) ;
#54228=CARTESIAN_POINT('Ctrl Pts',(-20.2464125993028,-16.1440425621064,
-19.4295409361418)) ;
#54229=CARTESIAN_POINT('Ctrl Pts',(-20.3141532070876,-16.1379127878752,
-19.4062848763401)) ;
#54230=CARTESIAN_POINT('Ctrl Pts',(-20.3825199747161,-16.1313557844546,
-19.3853614990262)) ;
#54231=CARTESIAN_POINT('Ctrl Pts',(-20.4512007972396,-16.1244124680041,
-19.3668244541829)) ;
#54232=CARTESIAN_POINT('Ctrl Pts',(-20.5029529309569,-16.119180564422,-19.3528564848399)) ;
#54233=CARTESIAN_POINT('Ctrl Pts',(-20.554883073648,-16.1137295207043,-19.3402424104641)) ;
#54234=CARTESIAN_POINT('Ctrl Pts',(-20.606855606863,-16.1080799337539,-19.3289859803215)) ;
#54235=CARTESIAN_POINT('Ctrl Pts',(-20.6738254274474,-16.1008000918637,
-19.3144813745146)) ;
#54236=CARTESIAN_POINT('Ctrl Pts',(-20.7408751366427,-16.0931892946345,
-19.3022309244371)) ;
#54237=CARTESIAN_POINT('Ctrl Pts',(-20.8076888303103,-16.0853002129681,
-19.2922065253502)) ;
#54238=CARTESIAN_POINT('Ctrl Pts',(-20.8750473484763,-16.0773468007024,
-19.2821003834662)) ;
#54239=CARTESIAN_POINT('Ctrl Pts',(-20.9421654869339,-16.0691106491234,
-19.2742566824985)) ;
#54240=CARTESIAN_POINT('Ctrl Pts',(-21.0087261038809,-16.0606518030573,
-19.268594124726)) ;
#54241=CARTESIAN_POINT('Ctrl Pts',(-21.0632349980193,-16.0537245483848,
-19.2639568515705)) ;
#54242=CARTESIAN_POINT('Ctrl Pts',(-21.1173700047693,-16.0466480826282,
-19.2607813391335)) ;
#54243=CARTESIAN_POINT('Ctrl Pts',(-21.1709635828472,-16.0394576303853,
-19.2589978739486)) ;
#54244=CARTESIAN_POINT('Ctrl Pts',(-21.236513880691,-16.0306629892538,-19.2568165179308)) ;
#54245=CARTESIAN_POINT('Ctrl Pts',(-21.3029353768662,-16.0214720150689,
-19.2566630206773)) ;
#54246=CARTESIAN_POINT('Ctrl Pts',(-21.3699240952328,-16.0119118209665,
-19.2586818931478)) ;
#54247=CARTESIAN_POINT('Ctrl Pts',(-21.4363641570234,-16.0024299275614,
-19.260684230481)) ;
#54248=CARTESIAN_POINT('Ctrl Pts',(-21.503361728513,-15.9925848997548,-19.2648236748315)) ;
#54249=CARTESIAN_POINT('Ctrl Pts',(-21.570606676331,-15.9824119250018,-19.2711927076656)) ;
#54250=CARTESIAN_POINT('Ctrl Pts',(-21.6258214515424,-15.9740589032143,
-19.2764223156535)) ;
#54251=CARTESIAN_POINT('Ctrl Pts',(-21.6812026362782,-15.965484957055,-19.2831542640125)) ;
#54252=CARTESIAN_POINT('Ctrl Pts',(-21.736575025046,-15.9567135267634,-19.2914139700576)) ;
#54253=CARTESIAN_POINT('Ctrl Pts',(-21.8059441321483,-15.9457249040784,
-19.3017615177437)) ;
#54254=CARTESIAN_POINT('Ctrl Pts',(-21.8753095721824,-15.9344245943001,
-19.3145095364013)) ;
#54255=CARTESIAN_POINT('Ctrl Pts',(-21.9443543422025,-15.9228603613541,
-19.3296652414138)) ;
#54256=CARTESIAN_POINT('Ctrl Pts',(-21.968052255654,-15.9188912237726,-19.3348670631533)) ;
#54257=CARTESIAN_POINT('Ctrl Pts',(-21.9917124088085,-15.914891049119,-19.3403520713795)) ;
#54258=CARTESIAN_POINT('Ctrl Pts',(-22.0153220904287,-15.9108619279123,
-19.3461191530285)) ;
#54259=CARTESIAN_POINT('',(-22.6529462781943,-15.9108618960635,-18.5954499255471)) ;
#54260=CARTESIAN_POINT('Origin',(-2.92277791062251E-15,-15.9108618782028,
0.)) ;
#54261=CARTESIAN_POINT('',(-22.6264860066071,-16.1877442736409,-16.1990085395056)) ;
#54262=CARTESIAN_POINT('Ctrl Pts',(-22.6529462422389,-15.9108619316234,
-18.5954499384047)) ;
#54263=CARTESIAN_POINT('Ctrl Pts',(-22.6252363683656,-15.9226009290868,
-18.5302867682431)) ;
#54264=CARTESIAN_POINT('Ctrl Pts',(-22.599823774383,-15.9340937870884,-18.4643124701177)) ;
#54265=CARTESIAN_POINT('Ctrl Pts',(-22.5767699773912,-15.945290667473,-18.3978371803287)) ;
#54266=CARTESIAN_POINT('Ctrl Pts',(-22.5688573329178,-15.9491337191718,
-18.3750211845709)) ;
#54267=CARTESIAN_POINT('Ctrl Pts',(-22.5612221261822,-15.9529419543584,
-18.3521462769307)) ;
#54268=CARTESIAN_POINT('Ctrl Pts',(-22.5538654687518,-15.9567135267635,
-18.3292252755274)) ;
#54269=CARTESIAN_POINT('Ctrl Pts',(-22.5330564685454,-15.9673817754482,
-18.2643910587044)) ;
#54270=CARTESIAN_POINT('Ctrl Pts',(-22.5144769423616,-15.9777576912909,
-18.1991782784233)) ;
#54271=CARTESIAN_POINT('Ctrl Pts',(-22.4981281668995,-15.987799766173,-18.133905742799)) ;
#54272=CARTESIAN_POINT('Ctrl Pts',(-22.4816461901464,-15.9979236586409,
-18.0681014006162)) ;
#54273=CARTESIAN_POINT('Ctrl Pts',(-22.4674314436314,-16.0077081692744,
-18.0022368323092)) ;
#54274=CARTESIAN_POINT('Ctrl Pts',(-22.4554326091091,-16.0171189356805,
-17.9366391572315)) ;
#54275=CARTESIAN_POINT('Ctrl Pts',(-22.4456135533074,-16.0248200870136,
-17.8829583409114)) ;
#54276=CARTESIAN_POINT('Ctrl Pts',(-22.4372773980355,-16.0322710948774,
-17.8294563747781)) ;
#54277=CARTESIAN_POINT('Ctrl Pts',(-22.4303706569622,-16.0394576303854,
-17.7763092436615)) ;
#54278=CARTESIAN_POINT('Ctrl Pts',(-22.4219200117541,-16.0482506141108,
-17.7112818241983)) ;
#54279=CARTESIAN_POINT('Ctrl Pts',(-22.4153939109251,-16.0568730319548,
-17.6451179903573)) ;
#54280=CARTESIAN_POINT('Ctrl Pts',(-22.410963519559,-16.0652608298863,-17.5781015904011)) ;
#54281=CARTESIAN_POINT('Ctrl Pts',(-22.406569444511,-16.0735798722807,-17.5116345299279)) ;
#54282=CARTESIAN_POINT('Ctrl Pts',(-22.4042370763699,-16.0816680200506,
-17.4443292575847)) ;
#54283=CARTESIAN_POINT('Ctrl Pts',(-22.4040865980054,-16.0894673869308,
-17.3764826835936)) ;
#54284=CARTESIAN_POINT('Ctrl Pts',(-22.4039629491467,-16.0958761674667,
-17.3207327990841)) ;
#54285=CARTESIAN_POINT('Ctrl Pts',(-22.4053116973728,-16.1020900207684,
-17.2646179138511)) ;
#54286=CARTESIAN_POINT('Ctrl Pts',(-22.4081742619674,-16.108079933754,-17.2083097157992)) ;
#54287=CARTESIAN_POINT('Ctrl Pts',(-22.4117583610684,-16.1155796568301,
-17.1378085426898)) ;
#54288=CARTESIAN_POINT('Ctrl Pts',(-22.4177173266673,-16.1227292229207,
-17.0669938490745)) ;
#54289=CARTESIAN_POINT('Ctrl Pts',(-22.4260875084648,-16.1294814162036,
-16.9961807520905)) ;
#54290=CARTESIAN_POINT('Ctrl Pts',(-22.4344411408918,-16.1362202591732,
-16.9255076654682)) ;
#54291=CARTESIAN_POINT('Ctrl Pts',(-22.4451964796334,-16.1425632136357,
-16.8548366738882)) ;
#54292=CARTESIAN_POINT('Ctrl Pts',(-22.4583384511702,-16.1484717649149,
-16.7844824993424)) ;
#54293=CARTESIAN_POINT('Ctrl Pts',(-22.4682495303456,-16.1529277264406,
-16.7314245702261)) ;
#54294=CARTESIAN_POINT('Ctrl Pts',(-22.4795169415893,-16.1571367885211,
-16.6785469115667)) ;
#54295=CARTESIAN_POINT('Ctrl Pts',(-22.4921150243034,-16.1610860188908,
-16.6259824199178)) ;
#54296=CARTESIAN_POINT('Ctrl Pts',(-22.5095429691188,-16.166549308068,-16.5532657152817)) ;
#54297=CARTESIAN_POINT('Ctrl Pts',(-22.5295315907202,-16.171518536629,-16.4810997728415)) ;
#54298=CARTESIAN_POINT('Ctrl Pts',(-22.5519724374491,-16.1759680067789,
-16.4098267138496)) ;
#54299=CARTESIAN_POINT('Ctrl Pts',(-22.5744132841656,-16.1804174769265,
-16.3385536548968)) ;
#54300=CARTESIAN_POINT('Ctrl Pts',(-22.5993061026932,-16.184347145014,-16.2681740614176)) ;
#54301=CARTESIAN_POINT('Ctrl Pts',(-22.6264860066216,-16.1877442734701,
-16.1990085393905)) ;
#54302=CARTESIAN_POINT('',(-23.841304833414,-15.9108618782028,-17.0452026225194)) ;
#54303=CARTESIAN_POINT('Ctrl Pts',(-23.841304833414,-15.9108618782028,-17.0452026225194)) ;
#54304=CARTESIAN_POINT('Ctrl Pts',(-23.2259561080038,-16.0510971572507,
-16.6167225940414)) ;
#54305=CARTESIAN_POINT('Ctrl Pts',(-22.6264860065426,-16.1877442737199,
-16.1990085397092)) ;
#54306=CARTESIAN_POINT('',(-24.6591730128172,-15.9108618782028,-15.8389373042025)) ;
#54307=CARTESIAN_POINT('Origin',(-2.92277791062251E-15,-15.9108618782028,
0.)) ;
#54308=CARTESIAN_POINT('',(-23.4234276096243,-16.1877442736409,-15.0236076122501)) ;
#54309=CARTESIAN_POINT('Ctrl Pts',(-23.4234276097895,-16.1877442737199,
-15.0236076121148)) ;
#54310=CARTESIAN_POINT('Ctrl Pts',(-24.0333609985744,-16.0510971574224,
-15.4258894705628)) ;
#54311=CARTESIAN_POINT('Ctrl Pts',(-24.6591730128173,-15.9108618782028,
-15.8389373042025)) ;
#54312=CARTESIAN_POINT('',(-25.6594598237771,-15.9108618960635,-14.1611741945453)) ;
#54313=CARTESIAN_POINT('Ctrl Pts',(-23.4234276095227,-16.1877442734701,
-15.0236076123062)) ;
#54314=CARTESIAN_POINT('Ctrl Pts',(-23.4776204497976,-16.184347145014,-14.9727573155735)) ;
#54315=CARTESIAN_POINT('Ctrl Pts',(-23.5337876717588,-16.1804174769265,
-14.9235822937669)) ;
#54316=CARTESIAN_POINT('Ctrl Pts',(-23.5916924706681,-16.1759680067789,
-14.8763543910281)) ;
#54317=CARTESIAN_POINT('Ctrl Pts',(-23.6495972696091,-16.171518536629,-14.8291264882633)) ;
#54318=CARTESIAN_POINT('Ctrl Pts',(-23.7092391985723,-16.166549308068,-14.7838461553214)) ;
#54319=CARTESIAN_POINT('Ctrl Pts',(-23.7703405769756,-16.1610860188908,
-14.7407407733973)) ;
#54320=CARTESIAN_POINT('Ctrl Pts',(-23.8288857064871,-16.155851292919,-14.6994387564324)) ;
#54321=CARTESIAN_POINT('Ctrl Pts',(-23.8888082771604,-16.1501596984486,
-14.6601065616019)) ;
#54322=CARTESIAN_POINT('Ctrl Pts',(-23.949839692006,-16.1440425621066,-14.6229088370813)) ;
#54323=CARTESIAN_POINT('Ctrl Pts',(-24.0109971966116,-16.1379127878754,
-14.5856342627586)) ;
#54324=CARTESIAN_POINT('Ctrl Pts',(-24.0732676795727,-16.1313557844549,
-14.5505032282463)) ;
#54325=CARTESIAN_POINT('Ctrl Pts',(-24.1363578659418,-16.1244124680045,
-14.5176352225583)) ;
#54326=CARTESIAN_POINT('Ctrl Pts',(-24.1838973630142,-16.1191805644222,
-14.4928686376089)) ;
#54327=CARTESIAN_POINT('Ctrl Pts',(-24.2319017547066,-16.1137295207044,
-14.4693860276473)) ;
#54328=CARTESIAN_POINT('Ctrl Pts',(-24.2802393992346,-16.108079933754,-14.4472202082417)) ;
#54329=CARTESIAN_POINT('Ctrl Pts',(-24.3425254411343,-16.1008000918637,
-14.4186581802463)) ;
#54330=CARTESIAN_POINT('Ctrl Pts',(-24.4053740807431,-16.0931892946345,
-14.392280433382)) ;
#54331=CARTESIAN_POINT('Ctrl Pts',(-24.4684707578974,-16.0853002129681,
-14.3681274300352)) ;
#54332=CARTESIAN_POINT('Ctrl Pts',(-24.5320819495711,-16.0773468007023,
-14.3437774738302)) ;
#54333=CARTESIAN_POINT('Ctrl Pts',(-24.5959447393999,-16.0691106491233,
-14.3216887384619)) ;
#54334=CARTESIAN_POINT('Ctrl Pts',(-24.6597319235742,-16.0606518030571,
-14.3018500030175)) ;
#54335=CARTESIAN_POINT('Ctrl Pts',(-24.7119695534068,-16.0537245483847,
-14.2856033457633)) ;
#54336=CARTESIAN_POINT('Ctrl Pts',(-24.7641562724755,-16.0466480826282,
-14.2708646488106)) ;
#54337=CARTESIAN_POINT('Ctrl Pts',(-24.8161134701841,-16.0394576303854,
-14.2576018449789)) ;
#54338=CARTESIAN_POINT('Ctrl Pts',(-24.8796623114282,-16.0306629892537,
-14.241380111469)) ;
#54339=CARTESIAN_POINT('Ctrl Pts',(-24.9444979125622,-16.0214720150687,
-14.2269515446236)) ;
#54340=CARTESIAN_POINT('Ctrl Pts',(-25.0103544698237,-16.0119118209663,
-14.2145226227012)) ;
#54341=CARTESIAN_POINT('Ctrl Pts',(-25.0756716432292,-16.0024299275612,
-14.2021954971695)) ;
#54342=CARTESIAN_POINT('Ctrl Pts',(-25.1419927069031,-15.9925848997546,
-14.1918356661752)) ;
#54343=CARTESIAN_POINT('Ctrl Pts',(-25.2090346590021,-15.9824119250015,
-14.1836001185266)) ;
#54344=CARTESIAN_POINT('Ctrl Pts',(-25.2640827545833,-15.9740589032141,
-14.1768379166526)) ;
#54345=CARTESIAN_POINT('Ctrl Pts',(-25.3196163278975,-15.9654849570549,
-14.1715071581381)) ;
#54346=CARTESIAN_POINT('Ctrl Pts',(-25.3754697336308,-15.9567135267634,
-14.1676703300569)) ;
#54347=CARTESIAN_POINT('Ctrl Pts',(-25.4454414464462,-15.9457249040773,
-14.1628636503371)) ;
#54348=CARTESIAN_POINT('Ctrl Pts',(-25.5159256082289,-15.9344245942979,
-14.160402108223)) ;
#54349=CARTESIAN_POINT('Ctrl Pts',(-25.5866141784799,-15.9228603613507,
-14.1603608966696)) ;
#54350=CARTESIAN_POINT('Ctrl Pts',(-25.6108762783375,-15.918891224989,-14.1603467518252)) ;
#54351=CARTESIAN_POINT('Ctrl Pts',(-25.635162377422,-15.9148910515742,-14.1606172898976)) ;
#54352=CARTESIAN_POINT('Ctrl Pts',(-25.6594598224132,-15.9108619316234,
-14.1611741563845)) ;
#54353=CARTESIAN_POINT('',(-26.1208051708581,-15.9108618823941,-13.2909850543147)) ;
#54354=CARTESIAN_POINT('Origin',(-2.92277791062251E-15,-15.9108618782028,
0.)) ;
#54355=CARTESIAN_POINT('',(-25.5797993342587,-16.1877442736409,-10.9562590645362)) ;
#54356=CARTESIAN_POINT('Ctrl Pts',(-26.1208051521851,-15.9108618900532,
-13.2909850310202)) ;
#54357=CARTESIAN_POINT('Ctrl Pts',(-26.0797349595563,-15.9226008880842,
-13.2333021464419)) ;
#54358=CARTESIAN_POINT('Ctrl Pts',(-26.0407339689744,-15.9340937467161,
-13.1743332500262)) ;
#54359=CARTESIAN_POINT('Ctrl Pts',(-26.0039289294952,-15.9452906277871,
-13.1143680028723)) ;
#54360=CARTESIAN_POINT('Ctrl Pts',(-25.9912964683392,-15.9491336929542,
-13.0937863470422)) ;
#54361=CARTESIAN_POINT('Ctrl Pts',(-25.9789222960317,-15.9529419413758,
-13.0730875148955)) ;
#54362=CARTESIAN_POINT('Ctrl Pts',(-25.96681025371,-15.9567135267635,-13.0522837860431)) ;
#54363=CARTESIAN_POINT('Ctrl Pts',(-25.9325503162336,-15.9673817754482,
-12.9934386771153)) ;
#54364=CARTESIAN_POINT('Ctrl Pts',(-25.9003863489627,-15.9777576912909,
-12.9337445843205)) ;
#54365=CARTESIAN_POINT('Ctrl Pts',(-25.8703881330689,-15.987799766173,-12.8735125877646)) ;
#54366=CARTESIAN_POINT('Ctrl Pts',(-25.8401455073662,-15.9979236586409,
-12.8127898523318)) ;
#54367=CARTESIAN_POINT('Ctrl Pts',(-25.8121041584821,-16.0077081692744,
-12.7515209113459)) ;
#54368=CARTESIAN_POINT('Ctrl Pts',(-25.7862842889548,-16.0171189356805,
-12.6900362681975)) ;
#54369=CARTESIAN_POINT('Ctrl Pts',(-25.765155008506,-16.0248200870136,-12.6397212862801)) ;
#54370=CARTESIAN_POINT('Ctrl Pts',(-25.7455124067001,-16.0322710948774,
-12.589262193352)) ;
#54371=CARTESIAN_POINT('Ctrl Pts',(-25.7273420792229,-16.0394576303854,
-12.5388423577955)) ;
#54372=CARTESIAN_POINT('Ctrl Pts',(-25.7051100324156,-16.0482506141109,
-12.477151882183)) ;
#54373=CARTESIAN_POINT('Ctrl Pts',(-25.6845132397104,-16.0568730319549,
-12.4139378407768)) ;
#54374=CARTESIAN_POINT('Ctrl Pts',(-25.6657798834323,-16.0652608298865,
-12.3494406501917)) ;
#54375=CARTESIAN_POINT('Ctrl Pts',(-25.6472000861677,-16.0735798722809,
-12.2854721489032)) ;
#54376=CARTESIAN_POINT('Ctrl Pts',(-25.6304536034734,-16.0816680200508,
-12.220241826631)) ;
#54377=CARTESIAN_POINT('Ctrl Pts',(-25.6157216353318,-16.089467386931,-12.154013816237)) ;
#54378=CARTESIAN_POINT('Ctrl Pts',(-25.6036163001002,-16.0958761674668,
-12.0995939138967)) ;
#54379=CARTESIAN_POINT('Ctrl Pts',(-25.5928704737616,-16.1020900207685,
-12.0445010224976)) ;
#54380=CARTESIAN_POINT('Ctrl Pts',(-25.583561515064,-16.1080799337539,-11.9888939120547)) ;
#54381=CARTESIAN_POINT('Ctrl Pts',(-25.5719061517011,-16.11557965683,-11.9192705418331)) ;
#54382=CARTESIAN_POINT('Ctrl Pts',(-25.5625027341359,-16.1227292229207,
-11.8488304549445)) ;
#54383=CARTESIAN_POINT('Ctrl Pts',(-25.555454503103,-16.1294814162035,-11.7778735871511)) ;
#54384=CARTESIAN_POINT('Ctrl Pts',(-25.5484202077037,-16.1362202591731,
-11.7070570139801)) ;
#54385=CARTESIAN_POINT('Ctrl Pts',(-25.5437319184324,-16.1425632136356,
-11.6357261910069)) ;
#54386=CARTESIAN_POINT('Ctrl Pts',(-25.5414425701049,-16.1484717649147,
-11.5641917225591)) ;
#54387=CARTESIAN_POINT('Ctrl Pts',(-25.5397160473781,-16.1529277264405,
-11.5102436692869)) ;
#54388=CARTESIAN_POINT('Ctrl Pts',(-25.5393528992489,-16.1571367885211,
-11.4561801005468)) ;
#54389=CARTESIAN_POINT('Ctrl Pts',(-25.5403566338809,-16.1610860188908,
-11.4021363221146)) ;
#54390=CARTESIAN_POINT('Ctrl Pts',(-25.541745181025,-16.166549308068,-11.3273732006547)) ;
#54391=CARTESIAN_POINT('Ctrl Pts',(-25.5457529353466,-16.171518536629,-11.2525974950609)) ;
#54392=CARTESIAN_POINT('Ctrl Pts',(-25.5523475266828,-16.1759680067789,
-11.1781666418811)) ;
#54393=CARTESIAN_POINT('Ctrl Pts',(-25.5589421180155,-16.1804174769264,
-11.1037357887422)) ;
#54394=CARTESIAN_POINT('Ctrl Pts',(-25.568123424087,-16.184347145014,-11.0296504108911)) ;
#54395=CARTESIAN_POINT('Ctrl Pts',(-25.579799334248,-16.1877442734701,-10.9562590644207)) ;
#54396=CARTESIAN_POINT('',(-26.9481230865112,-15.9108618782028,-11.5215194621523)) ;
#54397=CARTESIAN_POINT('Ctrl Pts',(-26.9481230865112,-15.9108618782028,
-11.5215194621523)) ;
#54398=CARTESIAN_POINT('Ctrl Pts',(-26.2550503307714,-16.0510971574997,
-11.2353388445058)) ;
#54399=CARTESIAN_POINT('Ctrl Pts',(-25.5797993342394,-16.1877442737198,
-10.9562590647489)) ;
#54400=CARTESIAN_POINT('',(-27.4875585758881,-15.9108618782028,-10.167638474082)) ;
#54401=CARTESIAN_POINT('Origin',(-2.92277791062251E-15,-15.9108618782028,
0.)) ;
#54402=CARTESIAN_POINT('',(-26.1054324307094,-16.1877442736409,-9.63701947055377)) ;
#54403=CARTESIAN_POINT('Ctrl Pts',(-26.1054324308417,-16.1877442737199,
-9.637019470386)) ;
#54404=CARTESIAN_POINT('Ctrl Pts',(-26.7875846245017,-16.0510971573504,
-9.89877855358705)) ;
#54405=CARTESIAN_POINT('Ctrl Pts',(-27.4875585758881,-15.9108618782028,
-10.1676384740821)) ;
#54406=CARTESIAN_POINT('',(-28.1037900289265,-15.9108618823941,-8.31406834816473)) ;
#54407=CARTESIAN_POINT('Ctrl Pts',(-26.1054324306223,-16.1877442734701,
-9.63701947063037)) ;
#54408=CARTESIAN_POINT('Ctrl Pts',(-26.1474269617335,-16.184347145014,-9.57570816684729)) ;
#54409=CARTESIAN_POINT('Ctrl Pts',(-26.1917098491728,-16.1804174769264,
-9.51560853729301)) ;
#54410=CARTESIAN_POINT('Ctrl Pts',(-26.2381082630198,-16.1759680067789,
-9.45703697656336)) ;
#54411=CARTESIAN_POINT('Ctrl Pts',(-26.2845066768924,-16.171518536629,-9.39846541580148)) ;
#54412=CARTESIAN_POINT('Ctrl Pts',(-26.3330202775945,-16.166549308068,-9.34142246015677)) ;
#54413=CARTESIAN_POINT('Ctrl Pts',(-26.3834267567978,-16.1610860188908,
-9.28618986789506)) ;
#54414=CARTESIAN_POINT('Ctrl Pts',(-26.4317244209472,-16.155851292919,-9.23326799687132)) ;
#54415=CARTESIAN_POINT('Ctrl Pts',(-26.4817907759808,-16.1501596984485,
-9.1819737855022)) ;
#54416=CARTESIAN_POINT('Ctrl Pts',(-26.5333988990483,-16.1440425621064,
-9.13252577299347)) ;
#54417=CARTESIAN_POINT('Ctrl Pts',(-26.5851136435314,-16.1379127878752,
-9.08297560181711)) ;
#54418=CARTESIAN_POINT('Ctrl Pts',(-26.6383761432513,-16.1313557844547,
-9.03527959823452)) ;
#54419=CARTESIAN_POINT('Ctrl Pts',(-26.6929256664716,-16.1244124680042,
-8.98961750311754)) ;
#54420=CARTESIAN_POINT('Ctrl Pts',(-26.734029632851,-16.119180564422,-8.95521036054868)) ;
#54421=CARTESIAN_POINT('Ctrl Pts',(-26.7758636415409,-16.1137295207043,
-8.9219572357447)) ;
#54422=CARTESIAN_POINT('Ctrl Pts',(-26.8183061828457,-16.108079933754,-8.8899184761565)) ;
#54423=CARTESIAN_POINT('Ctrl Pts',(-26.8729960199674,-16.1008000918637,
-8.84863455465709)) ;
#54424=CARTESIAN_POINT('Ctrl Pts',(-26.9287048574528,-16.0931892946344,
-8.80936290513267)) ;
#54425=CARTESIAN_POINT('Ctrl Pts',(-26.985134187597,-16.085300212968,-8.77221066511824)) ;
#54426=CARTESIAN_POINT('Ctrl Pts',(-27.0420236641543,-16.0773468007022,
-8.73475547148128)) ;
#54427=CARTESIAN_POINT('Ctrl Pts',(-27.0996449522805,-16.0691106491232,
-8.69945454642825)) ;
#54428=CARTESIAN_POINT('Ctrl Pts',(-27.1576760858445,-16.060651803057,-8.66636727053211)) ;
#54429=CARTESIAN_POINT('Ctrl Pts',(-27.2051998778583,-16.0537245483846,
-8.63927090481558)) ;
#54430=CARTESIAN_POINT('Ctrl Pts',(-27.2529981162635,-16.0466480826281,
-8.61365818843598)) ;
#54431=CARTESIAN_POINT('Ctrl Pts',(-27.3008894727844,-16.0394576303854,
-8.5895361999242)) ;
#54432=CARTESIAN_POINT('Ctrl Pts',(-27.3594653842418,-16.0306629892537,
-8.56003259915179)) ;
#54433=CARTESIAN_POINT('Ctrl Pts',(-27.4196834496852,-16.0214720150686,
-8.53200362646388)) ;
#54434=CARTESIAN_POINT('Ctrl Pts',(-27.4813284664185,-16.0119118209661,
-8.5057080727237)) ;
#54435=CARTESIAN_POINT('Ctrl Pts',(-27.5424685930055,-16.0024299275609,
-8.4796278870161)) ;
#54436=CARTESIAN_POINT('Ctrl Pts',(-27.6050120496373,-15.9925848997542,
-8.45525319485998)) ;
#54437=CARTESIAN_POINT('Ctrl Pts',(-27.6687161988492,-15.9824119250011,
-8.43279815178344)) ;
#54438=CARTESIAN_POINT('Ctrl Pts',(-27.7210236270318,-15.9740589032138,
-8.41436033309198)) ;
#54439=CARTESIAN_POINT('Ctrl Pts',(-27.774112900757,-15.9654849570548,-8.39721612804761)) ;
#54440=CARTESIAN_POINT('Ctrl Pts',(-27.82783568028,-15.9567135267635,-8.38146217165729)) ;
#54441=CARTESIAN_POINT('Ctrl Pts',(-27.8951381992077,-15.9457249040889,
-8.36172601955273)) ;
#54442=CARTESIAN_POINT('Ctrl Pts',(-27.963445321592,-15.9344245943217,-8.34417001565522)) ;
#54443=CARTESIAN_POINT('Ctrl Pts',(-28.0324723730129,-15.9228603613872,
-8.32893381455141)) ;
#54444=CARTESIAN_POINT('Ctrl Pts',(-28.0561642792868,-15.918891211363,-8.32370434811628)) ;
#54445=CARTESIAN_POINT('Ctrl Pts',(-28.0799408226937,-15.9148910240721,
-8.31874775162405)) ;
#54446=CARTESIAN_POINT('Ctrl Pts',(-28.1037899993503,-15.9108618900532,
-8.314068352235)) ;
#54447=CARTESIAN_POINT('',(-28.3672841893431,-15.9108618818334,-7.36504824030182)) ;
#54448=CARTESIAN_POINT('Origin',(-2.92277791062251E-15,-15.9108618782028,
0.)) ;
#54449=CARTESIAN_POINT('',(-27.3370296749455,-16.187744273641,-5.20120709271515)) ;
#54450=CARTESIAN_POINT('Ctrl Pts',(-28.3672841674668,-15.9108618853164,
-7.36504822386666)) ;
#54451=CARTESIAN_POINT('Ctrl Pts',(-28.3147740575662,-15.922600883412,-7.31754281092639)) ;
#54452=CARTESIAN_POINT('Ctrl Pts',(-28.2640083183597,-15.9340937421158,
-7.26833663508417)) ;
#54453=CARTESIAN_POINT('Ctrl Pts',(-28.2151730041596,-15.9452906232649,
-7.21768533801899)) ;
#54454=CARTESIAN_POINT('Ctrl Pts',(-28.1984114285588,-15.9491336899667,
-7.20030046891469)) ;
#54455=CARTESIAN_POINT('Ctrl Pts',(-28.1818769138879,-15.9529419398964,
-7.18274563840582)) ;
#54456=CARTESIAN_POINT('Ctrl Pts',(-28.1655758512416,-15.9567135267634,
-7.16503201329499)) ;
#54457=CARTESIAN_POINT('Ctrl Pts',(-28.1194669330942,-15.9673817754482,
-7.11492754415393)) ;
#54458=CARTESIAN_POINT('Ctrl Pts',(-28.0752224760982,-15.9777576912909,
-7.06354336827925)) ;
#54459=CARTESIAN_POINT('Ctrl Pts',(-28.0329775030073,-15.987799766173,-7.01116829200742)) ;
#54460=CARTESIAN_POINT('Ctrl Pts',(-27.9903883399206,-15.9979236586409,
-6.95836649094546)) ;
#54461=CARTESIAN_POINT('Ctrl Pts',(-27.9498315709757,-16.0077081692744,
-6.90455804486584)) ;
#54462=CARTESIAN_POINT('Ctrl Pts',(-27.9113979748458,-16.0171189356805,
-6.85006138722518)) ;
#54463=CARTESIAN_POINT('Ctrl Pts',(-27.8799464514201,-16.0248200870136,
-6.80546491234382)) ;
#54464=CARTESIAN_POINT('Ctrl Pts',(-27.8499158693093,-16.0322710948774,
-6.76040810372474)) ;
#54465=CARTESIAN_POINT('Ctrl Pts',(-27.8213315797461,-16.0394576303854,
-6.71507313920122)) ;
#54466=CARTESIAN_POINT('Ctrl Pts',(-27.7863576771393,-16.0482506141109,
-6.6596041855153)) ;
#54467=CARTESIAN_POINT('Ctrl Pts',(-27.752653275693,-16.0568730319549,-6.60229575486319)) ;
#54468=CARTESIAN_POINT('Ctrl Pts',(-27.7204929054219,-16.0652608298865,
-6.54333359059779)) ;
#54469=CARTESIAN_POINT('Ctrl Pts',(-27.6885961566106,-16.0735798722809,
-6.48485474451842)) ;
#54470=CARTESIAN_POINT('Ctrl Pts',(-27.6582186062815,-16.0816680200509,
-6.42474946968839)) ;
#54471=CARTESIAN_POINT('Ctrl Pts',(-27.6295939988196,-16.0894673869311,
-6.36323677105028)) ;
#54472=CARTESIAN_POINT('Ctrl Pts',(-27.6060730092364,-16.0958761674669,
-6.3126914650289)) ;
#54473=CARTESIAN_POINT('Ctrl Pts',(-27.5837350712296,-16.1020900207685,
-6.26119664983373)) ;
#54474=CARTESIAN_POINT('Ctrl Pts',(-27.5626898658027,-16.1080799337539,
-6.20889075368096)) ;
#54475=CARTESIAN_POINT('Ctrl Pts',(-27.5363400318123,-16.1155796568301,
-6.14340069775686)) ;
#54476=CARTESIAN_POINT('Ctrl Pts',(-27.512013924437,-16.1227292229208,-6.07662891776802)) ;
#54477=CARTESIAN_POINT('Ctrl Pts',(-27.4898768480231,-16.1294814162037,
-6.00884614343911)) ;
#54478=CARTESIAN_POINT('Ctrl Pts',(-27.4677835406323,-16.1362202591734,
-5.94119738797336)) ;
#54479=CARTESIAN_POINT('Ctrl Pts',(-27.4478708425436,-16.142563213636,-5.87254208360997)) ;
#54480=CARTESIAN_POINT('Ctrl Pts',(-27.4302572217353,-16.1484717649152,
-5.80317219349924)) ;
#54481=CARTESIAN_POINT('Ctrl Pts',(-27.4169738273903,-16.1529277264408,
-5.75085656708513)) ;
#54482=CARTESIAN_POINT('Ctrl Pts',(-27.4049971002915,-16.1571367885212,
-5.69813504065318)) ;
#54483=CARTESIAN_POINT('Ctrl Pts',(-27.3943595533256,-16.1610860188908,
-5.64513900245386)) ;
#54484=CARTESIAN_POINT('Ctrl Pts',(-27.3796437758774,-16.166549308068,-5.57182530463607)) ;
#54485=CARTESIAN_POINT('Ctrl Pts',(-27.3674832647814,-16.171518536629,-5.4979362647745)) ;
#54486=CARTESIAN_POINT('Ctrl Pts',(-27.3579232449636,-16.1759680067789,
-5.42382792137737)) ;
#54487=CARTESIAN_POINT('Ctrl Pts',(-27.348363225151,-16.1804174769265,-5.34971957802103)) ;
#54488=CARTESIAN_POINT('Ctrl Pts',(-27.3414037110988,-16.184347145014,-5.27539256572608)) ;
#54489=CARTESIAN_POINT('Ctrl Pts',(-27.3370296749104,-16.1877442734702,
-5.20120709260462)) ;
#54490=CARTESIAN_POINT('',(-28.7948770547711,-15.9108618782028,-5.4591028569837)) ;
#54491=CARTESIAN_POINT('Ctrl Pts',(-28.7948770547711,-15.9108618782028,
-5.45910285698361)) ;
#54492=CARTESIAN_POINT('Ctrl Pts',(-28.0564875827971,-16.0510971572643,
-5.32860313876284)) ;
#54493=CARTESIAN_POINT('Ctrl Pts',(-27.3370296749724,-16.1877442737199,
-5.20120709292708)) ;
#54494=CARTESIAN_POINT('',(-29.0306564501774,-15.9108618782028,-4.02091216943199)) ;
#54495=CARTESIAN_POINT('Origin',(-2.92277791062251E-15,-15.9108618782028,
0.)) ;
#54496=CARTESIAN_POINT('',(-27.5667762454386,-16.1877442736409,-3.79981500919265)) ;
#54497=CARTESIAN_POINT('Ctrl Pts',(-27.5667762455317,-16.1877442737199,
-3.79981500900038)) ;
#54498=CARTESIAN_POINT('Ctrl Pts',(-28.2892505640487,-16.0510971575924,
-3.90881175274295)) ;
#54499=CARTESIAN_POINT('Ctrl Pts',(-29.0306564501774,-15.9108618782028,
-4.02091216943207)) ;
#54500=CARTESIAN_POINT('',(-29.2340179925284,-15.9108618818334,-2.0782059266231)) ;
#54501=CARTESIAN_POINT('Ctrl Pts',(-27.56677624537,-16.1877442734702,-3.79981500928619)) ;
#54502=CARTESIAN_POINT('Ctrl Pts',(-27.5946088497164,-16.184347145014,-3.73090954687479)) ;
#54503=CARTESIAN_POINT('Ctrl Pts',(-27.624936784034,-16.1804174769265,-3.66269550145485)) ;
#54504=CARTESIAN_POINT('Ctrl Pts',(-27.6576592745555,-16.1759680067789,
-3.59551902381641)) ;
#54505=CARTESIAN_POINT('Ctrl Pts',(-27.690381765095,-16.171518536629,-3.528342546141)) ;
#54506=CARTESIAN_POINT('Ctrl Pts',(-27.7254985954864,-16.166549308068,-3.46220423300075)) ;
#54507=CARTESIAN_POINT('Ctrl Pts',(-27.7628532245447,-16.1610860188908,
-3.39742704502896)) ;
#54508=CARTESIAN_POINT('Ctrl Pts',(-27.798645078235,-16.155851292919,-3.33535988781728)) ;
#54509=CARTESIAN_POINT('Ctrl Pts',(-27.8365141705119,-16.1501596984485,
-3.27450212022401)) ;
#54510=CARTESIAN_POINT('Ctrl Pts',(-27.8762858633247,-16.1440425621065,
-3.21511595383477)) ;
#54511=CARTESIAN_POINT('Ctrl Pts',(-27.9161397237098,-16.1379127878753,
-3.15560709673814)) ;
#54512=CARTESIAN_POINT('Ctrl Pts',(-27.9579037448983,-16.1313557844547,
-3.09757633620262)) ;
#54513=CARTESIAN_POINT('Ctrl Pts',(-28.001361929891,-16.1244124680043,-3.04125526047473)) ;
#54514=CARTESIAN_POINT('Ctrl Pts',(-28.034108389794,-16.1191805644221,-2.99881640003158)) ;
#54515=CARTESIAN_POINT('Ctrl Pts',(-28.067815903731,-16.1137295207043,-2.95734763954236)) ;
#54516=CARTESIAN_POINT('Ctrl Pts',(-28.1023787757534,-16.1080799337539,
-2.91693403656097)) ;
#54517=CARTESIAN_POINT('Ctrl Pts',(-28.1469151720963,-16.1008000918637,
-2.86485861184352)) ;
#54518=CARTESIAN_POINT('Ctrl Pts',(-28.1928793241329,-16.0931892946345,
-2.81452935834372)) ;
#54519=CARTESIAN_POINT('Ctrl Pts',(-28.2400027345056,-16.0853002129681,
-2.76611507911336)) ;
#54520=CARTESIAN_POINT('Ctrl Pts',(-28.2875104072504,-16.0773468007024,
-2.71730601127082)) ;
#54521=CARTESIAN_POINT('Ctrl Pts',(-28.3361958862822,-16.0691106491234,
-2.67044352855458)) ;
#54522=CARTESIAN_POINT('Ctrl Pts',(-28.3857574979268,-16.0606518030573,
-2.62565483645402)) ;
#54523=CARTESIAN_POINT('Ctrl Pts',(-28.4263452924272,-16.0537245483848,
-2.58897575821992)) ;
#54524=CARTESIAN_POINT('Ctrl Pts',(-28.4675200576659,-16.0466480826283,
-2.55368664456423)) ;
#54525=CARTESIAN_POINT('Ctrl Pts',(-28.5091062263966,-16.0394576303854,
-2.51983338874492)) ;
#54526=CARTESIAN_POINT('Ctrl Pts',(-28.5599702635483,-16.0306629892539,
-2.47842747629227)) ;
#54527=CARTESIAN_POINT('Ctrl Pts',(-28.6127550634868,-16.021472015069,-2.43810870137365)) ;
#54528=CARTESIAN_POINT('Ctrl Pts',(-28.6673060872213,-16.0119118209667,
-2.399176066684)) ;
#54529=CARTESIAN_POINT('Ctrl Pts',(-28.7214103226214,-16.0024299275618,
-2.36056230129898)) ;
#54530=CARTESIAN_POINT('Ctrl Pts',(-28.7772517096891,-15.9925848997552,
-2.32331248149642)) ;
#54531=CARTESIAN_POINT('Ctrl Pts',(-28.834639320797,-15.9824119250023,-2.28768791584975)) ;
#54532=CARTESIAN_POINT('Ctrl Pts',(-28.8817602443783,-15.9740589032147,
-2.25843661224884)) ;
#54533=CARTESIAN_POINT('Ctrl Pts',(-28.929922823083,-15.9654849570552,-2.23028060464648)) ;
#54534=CARTESIAN_POINT('Ctrl Pts',(-28.9790029589372,-15.9567135267634,
-2.20334615743715)) ;
#54535=CARTESIAN_POINT('Ctrl Pts',(-29.0404892930589,-15.9457249040904,
-2.16960337348452)) ;
#54536=CARTESIAN_POINT('Ctrl Pts',(-29.1034254109862,-15.9344245943247,
-2.13777380703749)) ;
#54537=CARTESIAN_POINT('Ctrl Pts',(-29.1675633154367,-15.9228603613918,
-2.10805504422152)) ;
#54538=CARTESIAN_POINT('Ctrl Pts',(-29.1895771460413,-15.9188912098107,
-2.09785477628302)) ;
#54539=CARTESIAN_POINT('Ctrl Pts',(-29.2117322940924,-15.9148910209385,
-2.08790280445291)) ;
#54540=CARTESIAN_POINT('Ctrl Pts',(-29.2340179665494,-15.9108618853164,
-2.07820593521283)) ;
#54541=CARTESIAN_POINT('',(-29.2873405113753,-15.9108618818334,-1.09472993550088)) ;
#54542=CARTESIAN_POINT('Origin',(-2.92277791062251E-15,-15.9108618782028,
0.)) ;
#54543=CARTESIAN_POINT('',(-27.8160108909582,-16.1877442736409,0.797047542034005)) ;
#54544=CARTESIAN_POINT('Ctrl Pts',(-29.2873404864774,-15.9108618853164,
-1.09472992415271)) ;
#54545=CARTESIAN_POINT('Ctrl Pts',(-29.2258457742339,-15.922600883412,-1.0596232828087)) ;
#54546=CARTESIAN_POINT('Ctrl Pts',(-29.1656890365171,-15.9340937421157,
-1.02248065331821)) ;
#54547=CARTESIAN_POINT('Ctrl Pts',(-29.1071069331975,-15.9452906232649,
-0.983511704422473)) ;
#54548=CARTESIAN_POINT('Ctrl Pts',(-29.0870000009552,-15.9491336899667,
-0.970136527182337)) ;
#54549=CARTESIAN_POINT('Ctrl Pts',(-29.0670782844065,-15.9529419398964,
-0.95654655075281)) ;
#54550=CARTESIAN_POINT('Ctrl Pts',(-29.0473504257583,-15.9567135267634,
-0.942751306966341)) ;
#54551=CARTESIAN_POINT('Ctrl Pts',(-28.9915485287064,-15.9673817754481,
-0.903730306902203)) ;
#54552=CARTESIAN_POINT('Ctrl Pts',(-28.9372924036204,-15.9777576912908,
-0.863058714902215)) ;
#54553=CARTESIAN_POINT('Ctrl Pts',(-28.8847760013223,-15.9877997661729,
-0.820989559270527)) ;
#54554=CARTESIAN_POINT('Ctrl Pts',(-28.8318317227835,-15.9979236586407,
-0.778577646112123)) ;
#54555=CARTESIAN_POINT('Ctrl Pts',(-28.7806559232182,-16.0077081692741,
-0.734745718073906)) ;
#54556=CARTESIAN_POINT('Ctrl Pts',(-28.7314057127251,-16.0171189356801,
-0.68978524908376)) ;
#54557=CARTESIAN_POINT('Ctrl Pts',(-28.6911025846015,-16.0248200870134,
-0.652992562838112)) ;
#54558=CARTESIAN_POINT('Ctrl Pts',(-28.6520882188283,-16.0322710948773,
-0.615444844821693)) ;
#54559=CARTESIAN_POINT('Ctrl Pts',(-28.6144265367895,-16.0394576303853,
-0.577314563885692)) ;
#54560=CARTESIAN_POINT('Ctrl Pts',(-28.5683461191982,-16.0482506141109,
-0.530660798751411)) ;
#54561=CARTESIAN_POINT('Ctrl Pts',(-28.5231100893626,-16.056873031955,-0.481937657376859)) ;
#54562=CARTESIAN_POINT('Ctrl Pts',(-28.4790264882685,-16.0652608298866,
-0.431267524700463)) ;
#54563=CARTESIAN_POINT('Ctrl Pts',(-28.4353042444341,-16.0735798722811,
-0.381012739678)) ;
#54564=CARTESIAN_POINT('Ctrl Pts',(-28.3927160469611,-16.0816680200511,
-0.328842968138768)) ;
#54565=CARTESIAN_POINT('Ctrl Pts',(-28.3515372550096,-16.0894673869314,
-0.274921846678084)) ;
#54566=CARTESIAN_POINT('Ctrl Pts',(-28.3177004264064,-16.095876167467,-0.230614579308406)) ;
#54567=CARTESIAN_POINT('Ctrl Pts',(-28.2848148738862,-16.1020900207686,
-0.185125680643661)) ;
#54568=CARTESIAN_POINT('Ctrl Pts',(-28.2530174721459,-16.108079933754,-0.13856676435159)) ;
#54569=CARTESIAN_POINT('Ctrl Pts',(-28.2132052564801,-16.1155796568301,
-0.0802722649541275)) ;
#54570=CARTESIAN_POINT('Ctrl Pts',(-28.1750939210392,-16.1227292229208,
-0.0202909660870273)) ;
#54571=CARTESIAN_POINT('Ctrl Pts',(-28.138903104334,-16.1294814162037,0.0411482675837251)) ;
#54572=CARTESIAN_POINT('Ctrl Pts',(-28.1027838434504,-16.1362202591734,
0.102466024724218)) ;
#54573=CARTESIAN_POINT('Ctrl Pts',(-28.0685778321754,-16.1425632136359,
0.165235564750095)) ;
#54574=CARTESIAN_POINT('Ctrl Pts',(-28.036463532219,-16.1484717649151,0.229197217560653)) ;
#54575=CARTESIAN_POINT('Ctrl Pts',(-28.0122443830118,-16.1529277264407,
0.277434196571948)) ;
#54576=CARTESIAN_POINT('Ctrl Pts',(-27.9892140953912,-16.1571367885212,
0.326348480717388)) ;
#54577=CARTESIAN_POINT('Ctrl Pts',(-27.9674326667007,-16.1610860188908,
0.375818742840291)) ;
#54578=CARTESIAN_POINT('Ctrl Pts',(-27.9373006580581,-16.166549308068,0.444254949988105)) ;
#54579=CARTESIAN_POINT('Ctrl Pts',(-27.909540493528,-16.171518536629,0.513802354735114)) ;
#54580=CARTESIAN_POINT('Ctrl Pts',(-27.8842728784576,-16.1759680067789,
0.584122964577656)) ;
#54581=CARTESIAN_POINT('Ctrl Pts',(-27.859005263401,-16.1804174769265,0.654443574381521)) ;
#54582=CARTESIAN_POINT('Ctrl Pts',(-27.8362303483673,-16.184347145014,0.725536772633798)) ;
#54583=CARTESIAN_POINT('Ctrl Pts',(-27.8160108909,-16.1877442734702,0.797047542134341)) ;
#54584=CARTESIAN_POINT('',(-29.2952145751572,-15.9108618782028,0.858575330420999)) ;
#54585=CARTESIAN_POINT('Ctrl Pts',(-29.2952145751572,-15.9108618782028,
0.858575330421035)) ;
#54586=CARTESIAN_POINT('Ctrl Pts',(-28.5460346555085,-16.0510971575125,
0.827292127857017)) ;
#54587=CARTESIAN_POINT('Ctrl Pts',(-27.8160108910301,-16.1877442737199,
0.79704754183291)) ;
#54588=CARTESIAN_POINT('',(-29.2163130941136,-15.9108618782028,2.31382751933691)) ;
#54589=CARTESIAN_POINT('Origin',(-2.92277791062251E-15,-15.9108618782028,
0.)) ;
#54590=CARTESIAN_POINT('',(-27.7391282412025,-16.1877442736409,2.21506457880742)) ;
#54591=CARTESIAN_POINT('Ctrl Pts',(-27.7391282412522,-16.1877442737199,
2.21506457901514)) ;
#54592=CARTESIAN_POINT('Ctrl Pts',(-28.4681425923452,-16.0510971570914,
2.26392674104202)) ;
#54593=CARTESIAN_POINT('Ctrl Pts',(-29.2163130941136,-15.9108618782028,
2.31382751933687)) ;
#54594=CARTESIAN_POINT('',(-28.9972957403971,-15.9108618818334,4.25483109005219)) ;
#54595=CARTESIAN_POINT('Ctrl Pts',(-27.7391282411555,-16.1877442734701,
2.21506457870136)) ;
#54596=CARTESIAN_POINT('Ctrl Pts',(-27.7514974970917,-16.184347145014,2.28834225690161)) ;
#54597=CARTESIAN_POINT('Ctrl Pts',(-27.766452377786,-16.1804174769264,2.36148110523782)) ;
#54598=CARTESIAN_POINT('Ctrl Pts',(-27.7839688776935,-16.1759680067789,
2.43412140235194)) ;
#54599=CARTESIAN_POINT('Ctrl Pts',(-27.8014853776107,-16.171518536629,2.50676169950601)) ;
#54600=CARTESIAN_POINT('Ctrl Pts',(-27.8215634137317,-16.166549308068,2.57890281612686)) ;
#54601=CARTESIAN_POINT('Ctrl Pts',(-27.8441195317072,-16.1610860188908,
2.65019569049379)) ;
#54602=CARTESIAN_POINT('Ctrl Pts',(-27.8657319876396,-16.155851292919,2.71850594260504)) ;
#54603=CARTESIAN_POINT('Ctrl Pts',(-27.8896331004936,-16.1501596984485,
2.78608162484854)) ;
#54604=CARTESIAN_POINT('Ctrl Pts',(-27.9157086828988,-16.1440425621064,
2.85262911398106)) ;
#54605=CARTESIAN_POINT('Ctrl Pts',(-27.9418381369688,-16.1379127878752,
2.91931408897965)) ;
#54606=CARTESIAN_POINT('Ctrl Pts',(-27.9701508404126,-16.1313557844547,
2.98496615260209)) ;
#54607=CARTESIAN_POINT('Ctrl Pts',(-28.000485630748,-16.1244124680042,3.04931269803643)) ;
#54608=CARTESIAN_POINT('Ctrl Pts',(-28.0233433961044,-16.119180564422,3.09779888240661)) ;
#54609=CARTESIAN_POINT('Ctrl Pts',(-28.0473482893997,-16.1137295207043,
3.14554424542948)) ;
#54610=CARTESIAN_POINT('Ctrl Pts',(-28.0724153706577,-16.108079933754,3.19244299664483)) ;
#54611=CARTESIAN_POINT('Ctrl Pts',(-28.1047158538276,-16.1008000918638,
3.25287493559833)) ;
#54612=CARTESIAN_POINT('Ctrl Pts',(-28.138786087752,-16.0931892946346,3.31190845311691)) ;
#54613=CARTESIAN_POINT('Ctrl Pts',(-28.1744001400584,-16.0853002129682,
3.36932097367515)) ;
#54614=CARTESIAN_POINT('Ctrl Pts',(-28.2103046030145,-16.0773468007025,
3.42720165795851)) ;
#54615=CARTESIAN_POINT('Ctrl Pts',(-28.2477777940625,-16.0691106491235,
3.48343446072996)) ;
#54616=CARTESIAN_POINT('Ctrl Pts',(-28.2865524379113,-16.0606518030574,
3.53783029957149)) ;
#54617=CARTESIAN_POINT('Ctrl Pts',(-28.318306394737,-16.0537245483849,3.58237701739061)) ;
#54618=CARTESIAN_POINT('Ctrl Pts',(-28.3509324005486,-16.0466480826283,
3.62569244858873)) ;
#54619=CARTESIAN_POINT('Ctrl Pts',(-28.3842688584583,-16.0394576303854,
3.66769403109849)) ;
#54620=CARTESIAN_POINT('Ctrl Pts',(-28.4250426754601,-16.0306629892538,
3.71906616078553)) ;
#54621=CARTESIAN_POINT('Ctrl Pts',(-28.4679260513165,-16.0214720150689,
3.76978947683178)) ;
#54622=CARTESIAN_POINT('Ctrl Pts',(-28.5128323368133,-16.0119118209665,
3.81953874574425)) ;
#54623=CARTESIAN_POINT('Ctrl Pts',(-28.5573708271134,-16.0024299275614,
3.86888055405428)) ;
#54624=CARTESIAN_POINT('Ctrl Pts',(-28.6038990634226,-15.9925848997548,
3.91726374133018)) ;
#54625=CARTESIAN_POINT('Ctrl Pts',(-28.6522867555149,-15.9824119250018,
3.96439206445185)) ;
#54626=CARTESIAN_POINT('Ctrl Pts',(-28.6920178524757,-15.9740589032143,
4.00308909451437)) ;
#54627=CARTESIAN_POINT('Ctrl Pts',(-28.733001707505,-15.965484957055,4.04094036105058)) ;
#54628=CARTESIAN_POINT('Ctrl Pts',(-28.775144267083,-15.9567135267634,4.07779587426135)) ;
#54629=CARTESIAN_POINT('Ctrl Pts',(-28.8279393837613,-15.9457249040904,
4.12396751498949)) ;
#54630=CARTESIAN_POINT('Ctrl Pts',(-28.8825616743147,-15.9344245943247,
4.1685823288369)) ;
#54631=CARTESIAN_POINT('Ctrl Pts',(-28.9388114146762,-15.9228603613918,
4.21139403704719)) ;
#54632=CARTESIAN_POINT('Ctrl Pts',(-28.9581178180656,-15.9188912098107,
4.22608815124554)) ;
#54633=CARTESIAN_POINT('Ctrl Pts',(-28.9776156113019,-15.9148910209385,
4.24057015343419)) ;
#54634=CARTESIAN_POINT('Ctrl Pts',(-28.9972957168721,-15.9108618853164,
4.25483107607861)) ;
#54635=CARTESIAN_POINT('',(-28.8379530854688,-15.9108618948274,5.22677683844469)) ;
#54636=CARTESIAN_POINT('Origin',(-2.92277791062251E-15,-15.9108618782028,
0.)) ;
#54637=CARTESIAN_POINT('',(-26.9943463529852,-16.1877442736409,6.75803311957258)) ;
#54638=CARTESIAN_POINT('Ctrl Pts',(-28.8379530716378,-15.9108619275541,
5.22677680590787)) ;
#54639=CARTESIAN_POINT('Ctrl Pts',(-28.7703491834565,-15.9226009250731,
5.24784313359756)) ;
#54640=CARTESIAN_POINT('Ctrl Pts',(-28.7036143117797,-15.9340937831364,
5.27118547398356)) ;
#54641=CARTESIAN_POINT('Ctrl Pts',(-28.6380246560567,-15.9452906635882,
5.29664993508353)) ;
#54642=CARTESIAN_POINT('Ctrl Pts',(-28.6155126246555,-15.9491337166054,
5.30538998321425)) ;
#54643=CARTESIAN_POINT('Ctrl Pts',(-28.5931353023263,-15.9529419530875,
5.31437962277664)) ;
#54644=CARTESIAN_POINT('Ctrl Pts',(-28.5709031781777,-15.9567135267634,
5.32361140268328)) ;
#54645=CARTESIAN_POINT('Ctrl Pts',(-28.5080175369082,-15.9673817754481,
5.34972435507637)) ;
#54646=CARTESIAN_POINT('Ctrl Pts',(-28.4462866998398,-15.9777576912908,
5.37778160476311)) ;
#54647=CARTESIAN_POINT('Ctrl Pts',(-28.3859544769382,-15.9877997661729,
5.40757773279399)) ;
#54648=CARTESIAN_POINT('Ctrl Pts',(-28.3251306985681,-15.9979236586407,
5.4376166241273)) ;
#54649=CARTESIAN_POINT('Ctrl Pts',(-28.265728791892,-16.0077081692741,5.46942250188518)) ;
#54650=CARTESIAN_POINT('Ctrl Pts',(-28.2079648521405,-16.0171189356801,
5.50274448066511)) ;
#54651=CARTESIAN_POINT('Ctrl Pts',(-28.1606946487967,-16.0248200870134,
5.53001299315784)) ;
#54652=CARTESIAN_POINT('Ctrl Pts',(-28.1145207677436,-16.0322710948773,
5.55829593100791)) ;
#54653=CARTESIAN_POINT('Ctrl Pts',(-28.0695427116236,-16.0394576303853,
5.58743859879807)) ;
#54654=CARTESIAN_POINT('Ctrl Pts',(-28.0145104481598,-16.0482506141109,
5.62309569717482)) ;
#54655=CARTESIAN_POINT('Ctrl Pts',(-27.9598579764138,-16.056873031955,5.66095530933291)) ;
#54656=CARTESIAN_POINT('Ctrl Pts',(-27.9059124446885,-16.0652608298867,
5.70096413133199)) ;
#54657=CARTESIAN_POINT('Ctrl Pts',(-27.8524091093593,-16.0735798722811,
5.74064499740345)) ;
#54658=CARTESIAN_POINT('Ctrl Pts',(-27.7996016415232,-16.0816680200511,
5.7824398651166)) ;
#54659=CARTESIAN_POINT('Ctrl Pts',(-27.7477941396272,-16.0894673869313,
5.82624811768868)) ;
#54660=CARTESIAN_POINT('Ctrl Pts',(-27.7052236445022,-16.0958761674669,
5.86224558782921)) ;
#54661=CARTESIAN_POINT('Ctrl Pts',(-27.6633281693541,-16.1020900207685,
5.89960155962014)) ;
#54662=CARTESIAN_POINT('Ctrl Pts',(-27.6222653824652,-16.1080799337539,
5.93823645287304)) ;
#54663=CARTESIAN_POINT('Ctrl Pts',(-27.5708523600797,-16.1155796568302,
5.98660960974249)) ;
#54664=CARTESIAN_POINT('Ctrl Pts',(-27.5207378402602,-16.1227292229209,
6.03699576861805)) ;
#54665=CARTESIAN_POINT('Ctrl Pts',(-27.4721855256291,-16.1294814162039,
6.08921863134986)) ;
#54666=CARTESIAN_POINT('Ctrl Pts',(-27.4237292077474,-16.1362202591736,
6.14133823999151)) ;
#54667=CARTESIAN_POINT('Ctrl Pts',(-27.3768293183559,-16.1425632136362,
6.19528698175209)) ;
#54668=CARTESIAN_POINT('Ctrl Pts',(-27.3317159682247,-16.1484717649154,
6.25084962146588)) ;
#54669=CARTESIAN_POINT('Ctrl Pts',(-27.2976935246555,-16.1529277264409,
6.29275244554604)) ;
#54670=CARTESIAN_POINT('Ctrl Pts',(-27.2646865471668,-16.1571367885212,
6.3355723098413)) ;
#54671=CARTESIAN_POINT('Ctrl Pts',(-27.2327797121498,-16.1610860188907,
6.37920362141181)) ;
#54672=CARTESIAN_POINT('Ctrl Pts',(-27.1886404115476,-16.166549308068,6.43956233690491)) ;
#54673=CARTESIAN_POINT('Ctrl Pts',(-27.1465786280237,-16.171518536629,6.50151614718778)) ;
#54674=CARTESIAN_POINT('Ctrl Pts',(-27.1067849032983,-16.1759680067789,
6.56476090991532)) ;
#54675=CARTESIAN_POINT('Ctrl Pts',(-27.0669911785948,-16.1804174769265,
6.62800567260807)) ;
#54676=CARTESIAN_POINT('Ctrl Pts',(-27.0294657922941,-16.184347145014,6.69254081788182)) ;
#54677=CARTESIAN_POINT('Ctrl Pts',(-26.9943463529069,-16.1877442734701,
6.75803311965814)) ;
#54678=CARTESIAN_POINT('',(-28.4257404213015,-15.9108618782028,7.13610748961195)) ;
#54679=CARTESIAN_POINT('Ctrl Pts',(-28.4257404213014,-15.9108618782028,
7.1361074896125)) ;
#54680=CARTESIAN_POINT('Ctrl Pts',(-27.7008008765093,-16.0510971573508,
6.94450413403671)) ;
#54681=CARTESIAN_POINT('Ctrl Pts',(-26.9943463530986,-16.1877442737199,
6.75803311939151)) ;
#54682=CARTESIAN_POINT('',(-28.0358474093686,-15.9108618782028,8.54037520493741)) ;
#54683=CARTESIAN_POINT('Origin',(-2.92277791062251E-15,-15.9108618782028,
0.)) ;
#54684=CARTESIAN_POINT('',(-26.6144294302345,-16.1877442736409,8.12637020896991)) ;
#54685=CARTESIAN_POINT('Ctrl Pts',(-26.6144294302383,-16.1877442737199,
8.12637020918352)) ;
#54686=CARTESIAN_POINT('Ctrl Pts',(-27.315895907299,-16.0510971577038,8.3308065360743)) ;
#54687=CARTESIAN_POINT('Ctrl Pts',(-28.0358474093688,-15.9108618782028,
8.54037520493686)) ;
#54688=CARTESIAN_POINT('',(-27.4046920069319,-15.9108618948274,10.3889167040556)) ;
#54689=CARTESIAN_POINT('Ctrl Pts',(-26.6144294302115,-16.1877442734702,
8.12637020885619)) ;
#54690=CARTESIAN_POINT('Ctrl Pts',(-26.6107569650772,-16.184347145014,8.20059372005496)) ;
#54691=CARTESIAN_POINT('Ctrl Pts',(-26.6096395185481,-16.1804174769265,
8.27523748004725)) ;
#54692=CARTESIAN_POINT('Ctrl Pts',(-26.6111309757742,-16.1759680067789,
8.34994501707787)) ;
#54693=CARTESIAN_POINT('Ctrl Pts',(-26.6126224330011,-16.171518536629,8.4246525541496)) ;
#54694=CARTESIAN_POINT('Ctrl Pts',(-26.6167228481979,-16.166549308068,8.49942323581695)) ;
#54695=CARTESIAN_POINT('Ctrl Pts',(-26.6234257560832,-16.1610860188908,
8.57389822100999)) ;
#54696=CARTESIAN_POINT('Ctrl Pts',(-26.6298482398389,-16.155851292919,8.64525745655306)) ;
#54697=CARTESIAN_POINT('Ctrl Pts',(-26.6386637837969,-16.1501596984486,
8.7163912896496)) ;
#54698=CARTESIAN_POINT('Ctrl Pts',(-26.6498239905421,-16.1440425621066,
8.78698841489538)) ;
#54699=CARTESIAN_POINT('Ctrl Pts',(-26.6610072540654,-16.1379127878754,
8.85773139247953)) ;
#54700=CARTESIAN_POINT('Ctrl Pts',(-26.6745447692185,-16.1313557844549,
8.92793494166045)) ;
#54701=CARTESIAN_POINT('Ctrl Pts',(-26.690337743815,-16.1244124680045,8.99729818385233)) ;
#54702=CARTESIAN_POINT('Ctrl Pts',(-26.7022380109217,-16.1191805644222,
9.04956453205789)) ;
#54703=CARTESIAN_POINT('Ctrl Pts',(-26.7154178414446,-16.1137295207044,
9.10135397750546)) ;
#54704=CARTESIAN_POINT('Ctrl Pts',(-26.7298170230788,-16.108079933754,9.15254494347305)) ;
#54705=CARTESIAN_POINT('Ctrl Pts',(-26.7483712583824,-16.1008000918637,
9.21850766636298)) ;
#54706=CARTESIAN_POINT('Ctrl Pts',(-26.7689544879227,-16.0931892946345,
9.28348510623268)) ;
#54707=CARTESIAN_POINT('Ctrl Pts',(-26.7913939086595,-16.085300212968,9.34721132246741)) ;
#54708=CARTESIAN_POINT('Ctrl Pts',(-26.8140163090442,-16.0773468007022,
9.41145718672468)) ;
#54709=CARTESIAN_POINT('Ctrl Pts',(-26.8385250073438,-16.0691106491232,
9.47443092619252)) ;
#54710=CARTESIAN_POINT('Ctrl Pts',(-26.8646996241457,-16.0606518030571,
9.53589042280775)) ;
#54711=CARTESIAN_POINT('Ctrl Pts',(-26.8861349635669,-16.0537245483847,
9.58622182519577)) ;
#54712=CARTESIAN_POINT('Ctrl Pts',(-26.9086866541803,-16.0466480826282,
9.63553819251415)) ;
#54713=CARTESIAN_POINT('Ctrl Pts',(-26.9322146255474,-16.0394576303854,
9.68372415439674)) ;
#54714=CARTESIAN_POINT('Ctrl Pts',(-26.9609916840328,-16.0306629892538,
9.74266039762971)) ;
#54715=CARTESIAN_POINT('Ctrl Pts',(-26.991968456813,-16.0214720150688,9.8014164889199)) ;
#54716=CARTESIAN_POINT('Ctrl Pts',(-27.0251302360714,-16.0119118209664,
9.85965617153281)) ;
#54717=CARTESIAN_POINT('Ctrl Pts',(-27.0580204109656,-16.0024299275614,
9.91741885465047)) ;
#54718=CARTESIAN_POINT('Ctrl Pts',(-27.0930598878988,-15.9925848997548,
9.97467306533666)) ;
#54719=CARTESIAN_POINT('Ctrl Pts',(-27.1301851062715,-15.9824119250018,
10.0311014779233)) ;
#54720=CARTESIAN_POINT('Ctrl Pts',(-27.160668594677,-15.9740589032143,10.077434804331)) ;
#54721=CARTESIAN_POINT('Ctrl Pts',(-27.192557366521,-15.965484957055,10.1232114466471)) ;
#54722=CARTESIAN_POINT('Ctrl Pts',(-27.225791810576,-15.9567135267634,10.168264703024)) ;
#54723=CARTESIAN_POINT('Ctrl Pts',(-27.2674270688776,-15.9457249040784,
10.2247062659845)) ;
#54724=CARTESIAN_POINT('Ctrl Pts',(-27.3111814545091,-15.9344245943002,
10.2800201881814)) ;
#54725=CARTESIAN_POINT('Ctrl Pts',(-27.3569128554931,-15.9228603613542,
10.3339230139472)) ;
#54726=CARTESIAN_POINT('Ctrl Pts',(-27.372609030806,-15.9188912236551,10.3524238292486)) ;
#54727=CARTESIAN_POINT('Ctrl Pts',(-27.3885377175626,-15.914891048882,10.3707586359222)) ;
#54728=CARTESIAN_POINT('Ctrl Pts',(-27.4046919783062,-15.9108619275541,
10.3889167248043)) ;
#54729=CARTESIAN_POINT('',(-27.040135303883,-15.9108618883339,11.303885129792)) ;
#54730=CARTESIAN_POINT('Origin',(-2.92277791062251E-15,-15.9108618782028,
0.)) ;
#54731=CARTESIAN_POINT('',(-24.9104561816077,-16.1877442736409,12.4030205794544)) ;
#54732=CARTESIAN_POINT('Ctrl Pts',(-27.040135269086,-15.9108619232992,11.3038851331636)) ;
#54733=CARTESIAN_POINT('Ctrl Pts',(-26.9695832844262,-15.9226009208762,
11.3099261036344)) ;
#54734=CARTESIAN_POINT('Ctrl Pts',(-26.8993907236594,-15.934093779004,11.3183766877575)) ;
#54735=CARTESIAN_POINT('Ctrl Pts',(-26.8298604110735,-15.945290659526,11.3291459661828)) ;
#54736=CARTESIAN_POINT('Ctrl Pts',(-26.8059958379989,-15.9491337139218,
11.332842256655)) ;
#54737=CARTESIAN_POINT('Ctrl Pts',(-26.7822091698441,-15.9529419517586,
11.3368112619122)) ;
#54738=CARTESIAN_POINT('Ctrl Pts',(-26.7585122522638,-15.9567135267634,
11.3410479599125)) ;
#54739=CARTESIAN_POINT('Ctrl Pts',(-26.6914833294693,-15.9673817754482,
11.3530318520033)) ;
#54740=CARTESIAN_POINT('Ctrl Pts',(-26.6251642457505,-15.9777576912909,
11.367162833565)) ;
#54741=CARTESIAN_POINT('Ctrl Pts',(-26.5598372699333,-15.9877997661731,
11.3832927001646)) ;
#54742=CARTESIAN_POINT('Ctrl Pts',(-26.4939780440072,-15.997923658641,11.3995539845001)) ;
#54743=CARTESIAN_POINT('Ctrl Pts',(-26.4291275973556,-16.0077081692744,
11.4178466044834)) ;
#54744=CARTESIAN_POINT('Ctrl Pts',(-26.3655509059679,-16.0171189356805,
11.4379719943604)) ;
#54745=CARTESIAN_POINT('Ctrl Pts',(-26.3135239295762,-16.0248200870137,
11.4544412877625)) ;
#54746=CARTESIAN_POINT('Ctrl Pts',(-26.2623495726037,-16.0322710948774,
11.4721369667062)) ;
#54747=CARTESIAN_POINT('Ctrl Pts',(-26.2121582663181,-16.0394576303854,
11.490929342594)) ;
#54748=CARTESIAN_POINT('Ctrl Pts',(-26.1507474044579,-16.0482506141109,
11.513922487923)) ;
#54749=CARTESIAN_POINT('Ctrl Pts',(-26.089233979639,-16.0568730319549,11.5391482974777)) ;
#54750=CARTESIAN_POINT('Ctrl Pts',(-26.0279489503903,-16.0652608298865,
11.5666250407491)) ;
#54751=CARTESIAN_POINT('Ctrl Pts',(-25.9671662800619,-16.0735798722808,
11.5938765546741)) ;
#54752=CARTESIAN_POINT('Ctrl Pts',(-25.9066087603678,-16.0816680200508,
11.6233422369986)) ;
#54753=CARTESIAN_POINT('Ctrl Pts',(-25.8465950097364,-16.0894673869309,
11.6549891954811)) ;
#54754=CARTESIAN_POINT('Ctrl Pts',(-25.797281397127,-16.0958761674667,11.6809936666973)) ;
#54755=CARTESIAN_POINT('Ctrl Pts',(-25.7483349852048,-16.1020900207684,
11.7084699878918)) ;
#54756=CARTESIAN_POINT('Ctrl Pts',(-25.6999268634434,-16.1080799337539,
11.737374333437)) ;
#54757=CARTESIAN_POINT('Ctrl Pts',(-25.6393170501245,-16.1155796568301,
11.7735642727251)) ;
#54758=CARTESIAN_POINT('Ctrl Pts',(-25.5795426451758,-16.1227292229208,
11.8119992908194)) ;
#54759=CARTESIAN_POINT('Ctrl Pts',(-25.5208990848898,-16.1294814162036,
11.8525638995912)) ;
#54760=CARTESIAN_POINT('Ctrl Pts',(-25.4623714735797,-16.1362202591733,
11.8930483047598)) ;
#54761=CARTESIAN_POINT('Ctrl Pts',(-25.4049706927747,-16.1425632136359,
11.9356536650492)) ;
#54762=CARTESIAN_POINT('Ctrl Pts',(-25.3489677425815,-16.1484717649151,
11.9802192443856)) ;
#54763=CARTESIAN_POINT('Ctrl Pts',(-25.3067328562967,-16.1529277264407,
12.0138285840543)) ;
#54764=CARTESIAN_POINT('Ctrl Pts',(-25.265292558521,-16.1571367885212,12.0485518192378)) ;
#54765=CARTESIAN_POINT('Ctrl Pts',(-25.2247522453195,-16.1610860188908,
12.0843040286216)) ;
#54766=CARTESIAN_POINT('Ctrl Pts',(-25.1686695573967,-16.166549308068,12.1337629460074)) ;
#54767=CARTESIAN_POINT('Ctrl Pts',(-25.1142729171279,-16.171518536629,12.1852262705141)) ;
#54768=CARTESIAN_POINT('Ctrl Pts',(-25.0618137930884,-16.1759680067789,
12.2384379313129)) ;
#54769=CARTESIAN_POINT('Ctrl Pts',(-25.0093546690776,-16.1804174769265,
12.2916495920825)) ;
#54770=CARTESIAN_POINT('Ctrl Pts',(-24.9588334568666,-16.184347145014,12.3466090927105)) ;
#54771=CARTESIAN_POINT('Ctrl Pts',(-24.9104561815128,-16.1877442734702,
12.403020579521)) ;
#54772=CARTESIAN_POINT('',(-26.2271102382868,-15.9108618782028,13.0799631938038)) ;
#54773=CARTESIAN_POINT('Ctrl Pts',(-26.2271102382867,-15.9108618782028,
13.0799631938041)) ;
#54774=CARTESIAN_POINT('Ctrl Pts',(-25.5603084370629,-16.0510971568938,
12.7369988462526)) ;
#54775=CARTESIAN_POINT('Ctrl Pts',(-24.9104561817574,-16.1877442737198,
12.4030205793021)) ;
#54776=CARTESIAN_POINT('',(-25.5444566593682,-15.9108618782028,14.3675844378995)) ;
#54777=CARTESIAN_POINT('Origin',(-2.92277791062251E-15,-15.9108618782028,
0.)) ;
#54778=CARTESIAN_POINT('',(-24.2452694789224,-16.1877442736409,13.657695799973)) ;
#54779=CARTESIAN_POINT('Ctrl Pts',(-24.2452694788804,-16.1877442737198,
13.6576958001824)) ;
#54780=CARTESIAN_POINT('Ctrl Pts',(-24.8863882954023,-16.0510971570495,
14.0081470784022)) ;
#54781=CARTESIAN_POINT('Ctrl Pts',(-25.5444566593684,-15.9108618782028,
14.3675844378992)) ;
#54782=CARTESIAN_POINT('',(-24.530675536546,-15.9108618883339,16.0372283765163)) ;
#54783=CARTESIAN_POINT('Ctrl Pts',(-24.2452694789243,-16.1877442734701,
13.6576957998571)) ;
#54784=CARTESIAN_POINT('Ctrl Pts',(-24.2257270131077,-16.184347145014,13.7293945351642)) ;
#54785=CARTESIAN_POINT('Ctrl Pts',(-24.2085894899129,-16.1804174769265,
13.8020529475559)) ;
#54786=CARTESIAN_POINT('Ctrl Pts',(-24.1939861655753,-16.1759680067789,
13.8753344831029)) ;
#54787=CARTESIAN_POINT('Ctrl Pts',(-24.1793828412297,-16.171518536629,13.9486160186902)) ;
#54788=CARTESIAN_POINT('Ctrl Pts',(-24.167313904645,-16.166549308068,14.0225200714308)) ;
#54789=CARTESIAN_POINT('Ctrl Pts',(-24.1578501819171,-16.1610860188908,
14.0966947999152)) ;
#54790=CARTESIAN_POINT('Ctrl Pts',(-24.1487823852938,-16.155851292919,14.1677663403465)) ;
#54791=CARTESIAN_POINT('Ctrl Pts',(-24.1421001553184,-16.1501596984486,
14.2391321853203)) ;
#54792=CARTESIAN_POINT('Ctrl Pts',(-24.13782314754,-16.1440425621066,14.3104779035662)) ;
#54793=CARTESIAN_POINT('Ctrl Pts',(-24.1335373035436,-16.1379127878754,
14.3819710207296)) ;
#54794=CARTESIAN_POINT('Ctrl Pts',(-24.1316666312436,-16.1313557844549,
14.4534434155352)) ;
#54795=CARTESIAN_POINT('Ctrl Pts',(-24.1321793281619,-16.1244124680045,
14.5245800063717)) ;
#54796=CARTESIAN_POINT('Ctrl Pts',(-24.1325656537547,-16.1191805644222,
14.5781826020598)) ;
#54797=CARTESIAN_POINT('Ctrl Pts',(-24.134304147278,-16.1137295207044,14.6315945130223)) ;
#54798=CARTESIAN_POINT('Ctrl Pts',(-24.1373621395585,-16.108079933754,14.6846840610676)) ;
#54799=CARTESIAN_POINT('Ctrl Pts',(-24.1413025515743,-16.1008000918638,
14.7530932242828)) ;
#54800=CARTESIAN_POINT('Ctrl Pts',(-24.1474363277936,-16.0931892946346,
14.8209763136315)) ;
#54801=CARTESIAN_POINT('Ctrl Pts',(-24.1556518745863,-16.0853002129683,
14.8880364584972)) ;
#54802=CARTESIAN_POINT('Ctrl Pts',(-24.1639344141002,-16.0773468007026,
14.9556434375189)) ;
#54803=CARTESIAN_POINT('Ctrl Pts',(-24.1743326201581,-16.0691106491237,
15.0224135316151)) ;
#54804=CARTESIAN_POINT('Ctrl Pts',(-24.1866833139219,-16.0606518030576,
15.0880629082488)) ;
#54805=CARTESIAN_POINT('Ctrl Pts',(-24.1967977432917,-16.053724548385,15.1418255547714)) ;
#54806=CARTESIAN_POINT('Ctrl Pts',(-24.2082206267189,-16.0466480826284,
15.1948368796874)) ;
#54807=CARTESIAN_POINT('Ctrl Pts',(-24.2208399697526,-16.0394576303854,
15.2469540989219)) ;
#54808=CARTESIAN_POINT('Ctrl Pts',(-24.23627468645,-16.0306629892539,15.3106986624695)) ;
#54809=CARTESIAN_POINT('Ctrl Pts',(-24.2538964166868,-16.021472015069,15.3747401594769)) ;
#54810=CARTESIAN_POINT('Ctrl Pts',(-24.2737630817652,-16.0119118209667,
15.4387470329595)) ;
#54811=CARTESIAN_POINT('Ctrl Pts',(-24.2934670332299,-16.0024299275618,
15.5022296720201)) ;
#54812=CARTESIAN_POINT('Ctrl Pts',(-24.3153793437887,-15.9925848997553,
15.5656777628575)) ;
#54813=CARTESIAN_POINT('Ctrl Pts',(-24.3395061544923,-15.9824119250024,
15.6287677350517)) ;
#54814=CARTESIAN_POINT('Ctrl Pts',(-24.3593166603049,-15.9740589032147,
15.6805708629588)) ;
#54815=CARTESIAN_POINT('Ctrl Pts',(-24.3806192654345,-15.9654849570552,
15.7321324161385)) ;
#54816=CARTESIAN_POINT('Ctrl Pts',(-24.4033915883005,-15.9567135267634,
15.7832767754878)) ;
#54817=CARTESIAN_POINT('Ctrl Pts',(-24.4319201697606,-15.9457249040799,
15.8473491158683)) ;
#54818=CARTESIAN_POINT('Ctrl Pts',(-24.4627607439619,-15.9344245943031,
15.9107757288349)) ;
#54819=CARTESIAN_POINT('Ctrl Pts',(-24.4958354560159,-15.9228603613588,
15.9732492358817)) ;
#54820=CARTESIAN_POINT('Ctrl Pts',(-24.5071875390631,-15.918891222261,15.9946917336754)) ;
#54821=CARTESIAN_POINT('Ctrl Pts',(-24.5188023846988,-15.9148910460673,
16.0160220870393)) ;
#54822=CARTESIAN_POINT('Ctrl Pts',(-24.5306755198089,-15.9108619232992,
16.0372283458231)) ;
#54823=CARTESIAN_POINT('',(-23.9779507369461,-15.910861895147,16.8524363944926)) ;
#54824=CARTESIAN_POINT('Origin',(-2.92277791062251E-15,-15.9108618782028,
0.)) ;
#54825=CARTESIAN_POINT('',(-21.6617807651637,-16.1877442736408,17.4680565820063)) ;
#54826=CARTESIAN_POINT('Ctrl Pts',(-23.9779507384798,-15.9108619285364,
16.8524363584598)) ;
#54827=CARTESIAN_POINT('Ctrl Pts',(-23.9077495898749,-15.9226009260419,
16.8431695039185)) ;
#54828=CARTESIAN_POINT('Ctrl Pts',(-23.8373814663715,-15.9340937840903,
16.8363331931147)) ;
#54829=CARTESIAN_POINT('Ctrl Pts',(-23.7671616573665,-15.9452906645258,
16.831903730605)) ;
#54830=CARTESIAN_POINT('Ctrl Pts',(-23.7430604420255,-15.9491337172248,
16.8303834269855)) ;
#54831=CARTESIAN_POINT('Ctrl Pts',(-23.7189766846033,-15.9529419533942,
16.8291462092394)) ;
#54832=CARTESIAN_POINT('Ctrl Pts',(-23.6949230333843,-15.9567135267634,
16.8281897192057)) ;
#54833=CARTESIAN_POINT('Ctrl Pts',(-23.6268850269974,-15.9673817754483,
16.825484197519)) ;
#54834=CARTESIAN_POINT('Ctrl Pts',(-23.5590787032743,-15.9777576912911,
16.825028161963)) ;
#54835=CARTESIAN_POINT('Ctrl Pts',(-23.491811591325,-15.9877997661733,16.826737552496)) ;
#54836=CARTESIAN_POINT('Ctrl Pts',(-23.42399642205,-15.9979236586412,16.8284608702511)) ;
#54837=CARTESIAN_POINT('Ctrl Pts',(-23.3567297702322,-16.0077081692747,
16.8323848898801)) ;
#54838=CARTESIAN_POINT('Ctrl Pts',(-23.2903131026374,-16.0171189356809,
16.8383726499909)) ;
#54839=CARTESIAN_POINT('Ctrl Pts',(-23.2359620767902,-16.0248200870139,
16.8432726384477)) ;
#54840=CARTESIAN_POINT('Ctrl Pts',(-23.182180099954,-16.0322710948775,16.8495536282054)) ;
#54841=CARTESIAN_POINT('Ctrl Pts',(-23.1291224332011,-16.0394576303853,
16.8571170015809)) ;
#54842=CARTESIAN_POINT('Ctrl Pts',(-23.0642044765904,-16.048250614111,16.8663710599419)) ;
#54843=CARTESIAN_POINT('Ctrl Pts',(-22.9987063980747,-16.0568730319551,
16.8777835360754)) ;
#54844=CARTESIAN_POINT('Ctrl Pts',(-22.9329474911557,-16.0652608298868,
16.8914434186426)) ;
#54845=CARTESIAN_POINT('Ctrl Pts',(-22.8677276159361,-16.0735798722813,
16.9049913299185)) ;
#54846=CARTESIAN_POINT('Ctrl Pts',(-22.8022516466988,-16.0816680200513,
16.9207500442982)) ;
#54847=CARTESIAN_POINT('Ctrl Pts',(-22.7368378236097,-16.0894673869316,
16.9387559320863)) ;
#54848=CARTESIAN_POINT('Ctrl Pts',(-22.683086943236,-16.0958761674671,16.953551464205)) ;
#54849=CARTESIAN_POINT('Ctrl Pts',(-22.6293782743638,-16.1020900207686,
16.9698633725608)) ;
#54850=CARTESIAN_POINT('Ctrl Pts',(-22.5758883277042,-16.1080799337539,
16.9876856353241)) ;
#54851=CARTESIAN_POINT('Ctrl Pts',(-22.5089157709591,-16.1155796568301,
17.0100001556925)) ;
#54852=CARTESIAN_POINT('Ctrl Pts',(-22.4422764656216,-16.1227292229208,
17.0346868542773)) ;
#54853=CARTESIAN_POINT('Ctrl Pts',(-22.3762837673814,-16.1294814162037,
17.0616964530681)) ;
#54854=CARTESIAN_POINT('Ctrl Pts',(-22.3104215486986,-16.1362202591734,
17.0886526489736)) ;
#54855=CARTESIAN_POINT('Ctrl Pts',(-22.2452038731938,-16.1425632136359,
17.1179224484975)) ;
#54856=CARTESIAN_POINT('Ctrl Pts',(-22.1809299586464,-16.1484717649151,
17.1494071304985)) ;
#54857=CARTESIAN_POINT('Ctrl Pts',(-22.132457485989,-16.1529277264407,17.1731514503858)) ;
#54858=CARTESIAN_POINT('Ctrl Pts',(-22.0845215701936,-16.1571367885212,
17.1981544365714)) ;
#54859=CARTESIAN_POINT('Ctrl Pts',(-22.0372433987965,-16.1610860188908,
17.2243558101924)) ;
#54860=CARTESIAN_POINT('Ctrl Pts',(-21.9718396877092,-16.166549308068,17.2606022854633)) ;
#54861=CARTESIAN_POINT('Ctrl Pts',(-21.9076517171375,-16.171518536629,17.299168756337)) ;
#54862=CARTESIAN_POINT('Ctrl Pts',(-21.8449801241199,-16.1759680067789,
17.3398591970886)) ;
#54863=CARTESIAN_POINT('Ctrl Pts',(-21.7823085311368,-16.1804174769263,
17.3805496378177)) ;
#54864=CARTESIAN_POINT('Ctrl Pts',(-21.7211538087488,-16.1843471450139,
17.4233636486333)) ;
#54865=CARTESIAN_POINT('Ctrl Pts',(-21.6617807650567,-16.1877442734701,
17.4680565820512)) ;
#54866=CARTESIAN_POINT('',(-22.8021295298701,-15.9108618782028,18.4122143563869)) ;
#54867=CARTESIAN_POINT('Ctrl Pts',(-22.8021295298702,-15.9108618782028,
18.4122143563868)) ;
#54868=CARTESIAN_POINT('Ctrl Pts',(-22.2246443787864,-16.0510971574266,
17.9339256461324)) ;
#54869=CARTESIAN_POINT('Ctrl Pts',(-21.6617807653427,-16.1877442737198,
17.4680565818894)) ;
#54870=CARTESIAN_POINT('',(-21.8586355065995,-15.9108618782028,19.5229813909695)) ;
#54871=CARTESIAN_POINT('Origin',(-2.92277791062251E-15,-15.9108618782028,
0.)) ;
#54872=CARTESIAN_POINT('',(-20.7424276734563,-16.1877442736408,18.55040271481)) ;
#54873=CARTESIAN_POINT('Ctrl Pts',(-20.7424276733699,-16.1877442737198,
18.5504027150055)) ;
#54874=CARTESIAN_POINT('Ctrl Pts',(-21.2932208186878,-16.0510971580414,
19.0304822278201)) ;
#54875=CARTESIAN_POINT('Ctrl Pts',(-21.8586355065993,-15.9108618782028,
19.5229813909696)) ;
#54876=CARTESIAN_POINT('',(-20.5096319469963,-15.910861895147,20.935656936733)) ;
#54877=CARTESIAN_POINT('Ctrl Pts',(-20.7424276734832,-16.18774427347,18.5504027146971)) ;
#54878=CARTESIAN_POINT('Ctrl Pts',(-20.7079289909662,-16.1843471450139,
18.6162241209367)) ;
#54879=CARTESIAN_POINT('Ctrl Pts',(-20.6755727226435,-16.1804174769264,
18.6834997591179)) ;
#54880=CARTESIAN_POINT('Ctrl Pts',(-20.6455574519581,-16.1759680067789,
18.7519287300254)) ;
#54881=CARTESIAN_POINT('Ctrl Pts',(-20.6155421812561,-16.171518536629,18.8203577009705)) ;
#54882=CARTESIAN_POINT('Ctrl Pts',(-20.587868222951,-16.166549308068,18.8899394534164)) ;
#54883=CARTESIAN_POINT('Ctrl Pts',(-20.5626803827667,-16.1610860188908,
18.9603455973273)) ;
#54884=CARTESIAN_POINT('Ctrl Pts',(-20.5385463058567,-16.1558512929191,
19.0278062164059)) ;
#54885=CARTESIAN_POINT('Ctrl Pts',(-20.5166787555948,-16.1501596984487,
19.0960670856629)) ;
#54886=CARTESIAN_POINT('Ctrl Pts',(-20.4971645214231,-16.1440425621068,
19.1648253504181)) ;
#54887=CARTESIAN_POINT('Ctrl Pts',(-20.4776099712092,-16.1379127878757,
19.2337256684603)) ;
#54888=CARTESIAN_POINT('Ctrl Pts',(-20.4604185820138,-16.1313557844551,
19.3031249391449)) ;
#54889=CARTESIAN_POINT('Ctrl Pts',(-20.4456270281159,-16.1244124680049,
19.3727086107004)) ;
#54890=CARTESIAN_POINT('Ctrl Pts',(-20.4344813480391,-16.1191805644225,
19.4251410560729)) ;
#54891=CARTESIAN_POINT('Ctrl Pts',(-20.4246972145375,-16.1137295207045,
19.4776779509581)) ;
#54892=CARTESIAN_POINT('Ctrl Pts',(-20.4162710291437,-16.1080799337539,
19.5301836728207)) ;
#54893=CARTESIAN_POINT('Ctrl Pts',(-20.4054133685855,-16.1008000918638,
19.597840539921)) ;
#54894=CARTESIAN_POINT('Ctrl Pts',(-20.3968108829253,-16.0931892946347,
19.665455140938)) ;
#54895=CARTESIAN_POINT('Ctrl Pts',(-20.390418405937,-16.0853002129684,19.732713556593)) ;
#54896=CARTESIAN_POINT('Ctrl Pts',(-20.3839738022381,-16.0773468007026,
19.8005204231803)) ;
#54897=CARTESIAN_POINT('Ctrl Pts',(-20.379775307496,-16.0691106491238,19.8679647765148)) ;
#54898=CARTESIAN_POINT('Ctrl Pts',(-20.3777245735084,-16.0606518030577,
19.9347343412799)) ;
#54899=CARTESIAN_POINT('Ctrl Pts',(-20.3760451533504,-16.0537245483851,
19.9894143503377)) ;
#54900=CARTESIAN_POINT('Ctrl Pts',(-20.3758051082575,-16.0466480826284,
20.0436418822154)) ;
#54901=CARTESIAN_POINT('Ctrl Pts',(-20.3769257565024,-16.0394576303854,
20.0972534155537)) ;
#54902=CARTESIAN_POINT('Ctrl Pts',(-20.3782964212137,-16.0306629892539,
20.1628256744722)) ;
#54903=CARTESIAN_POINT('Ctrl Pts',(-20.3817391363867,-16.021472015069,20.2291580679745)) ;
#54904=CARTESIAN_POINT('Ctrl Pts',(-20.3873817441066,-16.0119118209667,
20.295939242062)) ;
#54905=CARTESIAN_POINT('Ctrl Pts',(-20.3929781372712,-16.0024299275617,
20.3621734594199)) ;
#54906=CARTESIAN_POINT('Ctrl Pts',(-20.4007386861682,-15.9925848997551,
20.4288486681995)) ;
#54907=CARTESIAN_POINT('Ctrl Pts',(-20.4107389463496,-15.9824119250022,
20.4956501830215)) ;
#54908=CARTESIAN_POINT('Ctrl Pts',(-20.4189501523347,-15.9740589032146,
20.5505008557405)) ;
#54909=CARTESIAN_POINT('Ctrl Pts',(-20.4286705046094,-15.9654849570552,
20.6054363588621)) ;
#54910=CARTESIAN_POINT('Ctrl Pts',(-20.4399158977778,-15.9567135267634,
20.6602803677819)) ;
#54911=CARTESIAN_POINT('Ctrl Pts',(-20.454003837642,-15.9457249040784,20.7289875341744)) ;
#54912=CARTESIAN_POINT('Ctrl Pts',(-20.4704885294489,-15.9344245943001,
20.7975610799983)) ;
#54913=CARTESIAN_POINT('Ctrl Pts',(-20.4893600158069,-15.9228603613541,
20.8656840765868)) ;
#54914=CARTESIAN_POINT('Ctrl Pts',(-20.4958371874622,-15.9188912239776,
20.8890656128477)) ;
#54915=CARTESIAN_POINT('Ctrl Pts',(-20.5025950859566,-15.9148910495321,
20.9123941127885)) ;
#54916=CARTESIAN_POINT('Ctrl Pts',(-20.5096319116864,-15.9108619285364,
20.935656944076)) ;
#54917=CARTESIAN_POINT('',(-19.7945838954017,-15.910861895547,21.6129864201278)) ;
#54918=CARTESIAN_POINT('Origin',(-2.92277791062251E-15,-15.9108618782028,
0.)) ;
#54919=CARTESIAN_POINT('',(-17.400224555478,-16.1877442736409,21.7163056731368)) ;
#54920=CARTESIAN_POINT('Ctrl Pts',(-19.7945839053568,-15.9108619297779,
21.6129863845241)) ;
#54921=CARTESIAN_POINT('Ctrl Pts',(-19.7280161203445,-15.9226009272665,
21.588845012237)) ;
#54922=CARTESIAN_POINT('Ctrl Pts',(-19.6607627691677,-15.934093785296,21.5670414642609)) ;
#54923=CARTESIAN_POINT('Ctrl Pts',(-19.5931368637526,-15.945290665711,21.547620377037)) ;
#54924=CARTESIAN_POINT('Ctrl Pts',(-19.5699259441484,-15.9491337180078,
21.5409545691427)) ;
#54925=CARTESIAN_POINT('Ctrl Pts',(-19.5466712192221,-15.952941953782,21.5345689816102)) ;
#54926=CARTESIAN_POINT('Ctrl Pts',(-19.5233855484791,-15.9567135267635,
21.5284640304184)) ;
#54927=CARTESIAN_POINT('Ctrl Pts',(-19.4575198400606,-15.9673817754482,
21.5111956021413)) ;
#54928=CARTESIAN_POINT('Ctrl Pts',(-19.3913968246702,-15.9777576912909,
21.4961738731834)) ;
#54929=CARTESIAN_POINT('Ctrl Pts',(-19.3253349119823,-15.9877997661731,
21.4833828584483)) ;
#54930=CARTESIAN_POINT('Ctrl Pts',(-19.2587347613034,-15.997923658641,21.4704876291999)) ;
#54931=CARTESIAN_POINT('Ctrl Pts',(-19.1921972181978,-16.0077081692744,
21.4598595656779)) ;
#54932=CARTESIAN_POINT('Ctrl Pts',(-19.1260461439565,-16.0171189356805,
21.4514297150146)) ;
#54933=CARTESIAN_POINT('Ctrl Pts',(-19.0719124622137,-16.0248200870136,
21.4445312805117)) ;
#54934=CARTESIAN_POINT('Ctrl Pts',(-19.0180376509747,-16.0322710948774,
21.4391038889833)) ;
#54935=CARTESIAN_POINT('Ctrl Pts',(-18.9645945412809,-16.0394576303854,
21.4350846049139)) ;
#54936=CARTESIAN_POINT('Ctrl Pts',(-18.8992049814215,-16.0482506141109,
21.4301668668228)) ;
#54937=CARTESIAN_POINT('Ctrl Pts',(-18.8327848665661,-16.0568730319549,
21.4272323748349)) ;
#54938=CARTESIAN_POINT('Ctrl Pts',(-18.7656268953802,-16.0652608298865,
21.4264366757703)) ;
#54939=CARTESIAN_POINT('Ctrl Pts',(-18.6990194241494,-16.0735798722809,
21.4256474991228)) ;
#54940=CARTESIAN_POINT('Ctrl Pts',(-18.6316865889201,-16.0816680200509,
21.4269623855873)) ;
#54941=CARTESIAN_POINT('Ctrl Pts',(-18.5639313710398,-16.0894673869311,
21.4304852673795)) ;
#54942=CARTESIAN_POINT('Ctrl Pts',(-18.5082565543254,-16.0958761674669,
21.4333800377636)) ;
#54943=CARTESIAN_POINT('Ctrl Pts',(-18.4522969861638,-16.1020900207685,
21.4377648065762)) ;
#54944=CARTESIAN_POINT('Ctrl Pts',(-18.3962263450592,-16.1080799337539,
21.44367163736)) ;
#54945=CARTESIAN_POINT('Ctrl Pts',(-18.3260226072069,-16.1155796568301,
21.4510673366371)) ;
#54946=CARTESIAN_POINT('Ctrl Pts',(-18.2556343813341,-16.1227292229208,
21.4608513931238)) ;
#54947=CARTESIAN_POINT('Ctrl Pts',(-18.185378290364,-16.1294814162037,21.4730430431129)) ;
#54948=CARTESIAN_POINT('Ctrl Pts',(-18.1152611084535,-16.1362202591734,
21.4852105879945)) ;
#54949=CARTESIAN_POINT('Ctrl Pts',(-18.0452760442714,-16.1425632136359,
21.4997762034582)) ;
#54950=CARTESIAN_POINT('Ctrl Pts',(-17.9757365421789,-16.1484717649151,
21.5167077993861)) ;
#54951=CARTESIAN_POINT('Ctrl Pts',(-17.9232930020967,-16.1529277264407,
21.5294768414841)) ;
#54952=CARTESIAN_POINT('Ctrl Pts',(-17.8711028984271,-16.1571367885211,
21.5435904668266)) ;
#54953=CARTESIAN_POINT('Ctrl Pts',(-17.8192975435827,-16.1610860188907,
21.5590158575752)) ;
#54954=CARTESIAN_POINT('Ctrl Pts',(-17.7476310141697,-16.166549308068,21.580355045833)) ;
#54955=CARTESIAN_POINT('Ctrl Pts',(-17.6766530714589,-16.171518536629,21.6042213377595)) ;
#54956=CARTESIAN_POINT('Ctrl Pts',(-17.6066994634978,-16.1759680067789,
21.6304879186787)) ;
#54957=CARTESIAN_POINT('Ctrl Pts',(-17.5367458555753,-16.1804174769264,
21.6567544995834)) ;
#54958=CARTESIAN_POINT('Ctrl Pts',(-17.46781714986,-16.184347145014,21.6854210850257)) ;
#54959=CARTESIAN_POINT('Ctrl Pts',(-17.4002245553638,-16.1877442734701,
21.7163056731577)) ;
#54960=CARTESIAN_POINT('',(-18.3109465873826,-15.9108618782028,22.883530839373)) ;
#54961=CARTESIAN_POINT('Ctrl Pts',(-18.3109465873823,-15.9108618782028,
22.8835308393732)) ;
#54962=CARTESIAN_POINT('Ctrl Pts',(-17.8497806514479,-16.05109715784,22.2922820144884)) ;
#54963=CARTESIAN_POINT('Ctrl Pts',(-17.4002245556779,-16.1877442737199,
21.716305673061)) ;
#54964=CARTESIAN_POINT('',(-17.1507288516715,-15.9108618782028,23.765505432432)) ;
#54965=CARTESIAN_POINT('Origin',(-2.92277791062251E-15,-15.9108618782028,
0.)) ;
#54966=CARTESIAN_POINT('',(-16.2696930035337,-16.1877442736409,22.5757134159908)) ;
#54967=CARTESIAN_POINT('Ctrl Pts',(-16.2696930034074,-16.1877442737198,
22.5757134161632)) ;
#54968=CARTESIAN_POINT('Ctrl Pts',(-16.7044060067849,-16.051097158066,23.1629731815623)) ;
#54969=CARTESIAN_POINT('Ctrl Pts',(-17.1507288516718,-15.9108618782028,
23.7655054324318)) ;
#54970=CARTESIAN_POINT('',(-15.5295807620181,-15.910861895547,24.8551575119669)) ;
#54971=CARTESIAN_POINT('Ctrl Pts',(-16.2696930035843,-16.1877442734701,
22.5757134158863)) ;
#54972=CARTESIAN_POINT('Ctrl Pts',(-16.2218512244183,-16.1843471450139,
22.6325797572584)) ;
#54973=CARTESIAN_POINT('Ctrl Pts',(-16.1757891541129,-16.1804174769264,
22.69132688716)) ;
#54974=CARTESIAN_POINT('Ctrl Pts',(-16.131765417777,-16.1759680067789,22.7517036308022)) ;
#54975=CARTESIAN_POINT('Ctrl Pts',(-16.0877416814168,-16.171518536629,22.8120803744776)) ;
#54976=CARTESIAN_POINT('Ctrl Pts',(-16.0457567049241,-16.166549308068,22.8740862612196)) ;
#54977=CARTESIAN_POINT('Ctrl Pts',(-16.0060225026959,-16.1610860188908,
22.9374317075191)) ;
#54978=CARTESIAN_POINT('Ctrl Pts',(-15.9679506281116,-16.155851292919,22.9981270216757)) ;
#54979=CARTESIAN_POINT('Ctrl Pts',(-15.931920259909,-16.1501596984485,23.0600911128376)) ;
#54980=CARTESIAN_POINT('Ctrl Pts',(-15.898081263245,-16.1440425621064,23.1230468640632)) ;
#54981=CARTESIAN_POINT('Ctrl Pts',(-15.8641723558478,-16.1379127878752,
23.1861326806915)) ;
#54982=CARTESIAN_POINT('Ctrl Pts',(-15.8324641000085,-16.1313557844547,
23.2502137944912)) ;
#54983=CARTESIAN_POINT('Ctrl Pts',(-15.8030599319149,-16.1244124680043,
23.3149908916223)) ;
#54984=CARTESIAN_POINT('Ctrl Pts',(-15.7809034057824,-16.1191805644221,
23.3638015038048)) ;
#54985=CARTESIAN_POINT('Ctrl Pts',(-15.7600541404651,-16.1137295207043,
23.4130068157949)) ;
#54986=CARTESIAN_POINT('Ctrl Pts',(-15.7405377764617,-16.108079933754,23.4624736022728)) ;
#54987=CARTESIAN_POINT('Ctrl Pts',(-15.7153897354694,-16.1008000918637,
23.5262146133492)) ;
#54988=CARTESIAN_POINT('Ctrl Pts',(-15.6924532305976,-16.0931892946344,
23.5903991424404)) ;
#54989=CARTESIAN_POINT('Ctrl Pts',(-15.6717516349474,-16.0853002129679,
23.6547109001225)) ;
#54990=CARTESIAN_POINT('Ctrl Pts',(-15.6508812305419,-16.0773468007021,
23.7195470805569)) ;
#54991=CARTESIAN_POINT('Ctrl Pts',(-15.6322823519474,-16.069110649123,23.784512070128)) ;
#54992=CARTESIAN_POINT('Ctrl Pts',(-15.6159260802505,-16.0606518030568,
23.8492797523866)) ;
#54993=CARTESIAN_POINT('Ctrl Pts',(-15.6025313383852,-16.0537245483845,
23.902320347526)) ;
#54994=CARTESIAN_POINT('Ctrl Pts',(-15.5906395890145,-16.0466480826281,
23.9552284672416)) ;
#54995=CARTESIAN_POINT('Ctrl Pts',(-15.5802091422045,-16.0394576303854,
24.0078274989672)) ;
#54996=CARTESIAN_POINT('Ctrl Pts',(-15.567451664171,-16.0306629892537,24.0721613673087)) ;
#54997=CARTESIAN_POINT('Ctrl Pts',(-15.5565543867448,-16.0214720150687,
24.1376830283097)) ;
#54998=CARTESIAN_POINT('Ctrl Pts',(-15.5477090950404,-16.0119118209662,
24.2041158895244)) ;
#54999=CARTESIAN_POINT('Ctrl Pts',(-15.5389362487803,-16.0024299275611,
24.2700046467905)) ;
#55000=CARTESIAN_POINT('Ctrl Pts',(-15.5321821613742,-15.9925848997544,
24.3367893148545)) ;
#55001=CARTESIAN_POINT('Ctrl Pts',(-15.5275882699818,-15.9824119250013,
24.4041788077167)) ;
#55002=CARTESIAN_POINT('Ctrl Pts',(-15.523816229274,-15.974058903214,24.4595122687521)) ;
#55003=CARTESIAN_POINT('Ctrl Pts',(-15.5214998158251,-15.9654849570548,
24.5152529987445)) ;
#55004=CARTESIAN_POINT('Ctrl Pts',(-15.52069245721,-15.9567135267634,24.571232212331)) ;
#55005=CARTESIAN_POINT('Ctrl Pts',(-15.5196810190638,-15.9457249040781,
24.6413615339908)) ;
#55006=CARTESIAN_POINT('Ctrl Pts',(-15.5210390226046,-15.9344245942994,
24.7118755898769)) ;
#55007=CARTESIAN_POINT('Ctrl Pts',(-15.5248248735337,-15.922860361353,24.7824627203936)) ;
#55008=CARTESIAN_POINT('Ctrl Pts',(-15.5261242732388,-15.9188912243845,
24.8066900072817)) ;
#55009=CARTESIAN_POINT('Ctrl Pts',(-15.5277092377278,-15.9148910503535,
24.8309258457799)) ;
#55010=CARTESIAN_POINT('Ctrl Pts',(-15.5295807250488,-15.9108619297779,
24.855157512034)) ;
#55011=CARTESIAN_POINT('',(-14.6856444869839,-15.9108618855281,25.36293728564)) ;
#55012=CARTESIAN_POINT('Origin',(-2.92277791062251E-15,-15.9108618782028,
0.)) ;
#55013=CARTESIAN_POINT('',(-12.3250531845394,-16.1877442736409,24.9491244469309)) ;
#55014=CARTESIAN_POINT('Ctrl Pts',(-14.6856444555744,-15.9108619063809,
25.3629372648498)) ;
#55015=CARTESIAN_POINT('Ctrl Pts',(-14.625822671402,-15.9226009041889,25.3250501955733)) ;
#55016=CARTESIAN_POINT('Ctrl Pts',(-14.5648287859113,-15.9340937625731,
25.2892989170221)) ;
#55017=CARTESIAN_POINT('Ctrl Pts',(-14.5029588974541,-15.9452906433744,
25.2557943104058)) ;
#55018=CARTESIAN_POINT('Ctrl Pts',(-14.4817235471669,-15.9491337032516,
25.2442946604876)) ;
#55019=CARTESIAN_POINT('Ctrl Pts',(-14.460385176184,-15.9529419464749,25.233059263703)) ;
#55020=CARTESIAN_POINT('Ctrl Pts',(-14.4389562540117,-15.9567135267634,
25.2220912907379)) ;
#55021=CARTESIAN_POINT('Ctrl Pts',(-14.3783426508824,-15.9673817754482,
25.1910674083842)) ;
#55022=CARTESIAN_POINT('Ctrl Pts',(-14.3169947825335,-15.9777576912909,
25.1621823853752)) ;
#55023=CARTESIAN_POINT('Ctrl Pts',(-14.2552270507214,-15.987799766173,25.1354890590048)) ;
#55024=CARTESIAN_POINT('Ctrl Pts',(-14.1929560676633,-15.9979236586409,
25.1085782493407)) ;
#55025=CARTESIAN_POINT('Ctrl Pts',(-14.130258854834,-16.0077081692743,25.0838950591058)) ;
#55026=CARTESIAN_POINT('Ctrl Pts',(-14.0674665246557,-16.0171189356804,
25.0614417681163)) ;
#55027=CARTESIAN_POINT('Ctrl Pts',(-14.016081417811,-16.0248200870136,25.043067473784)) ;
#55028=CARTESIAN_POINT('Ctrl Pts',(-13.9646328984659,-16.0322710948774,
25.0261854797651)) ;
#55029=CARTESIAN_POINT('Ctrl Pts',(-13.9133032862434,-16.0394576303854,
25.0107714755065)) ;
#55030=CARTESIAN_POINT('Ctrl Pts',(-13.8504996662784,-16.0482506141108,
24.991911888931)) ;
#55031=CARTESIAN_POINT('Ctrl Pts',(-13.7862632458327,-16.0568730319548,
24.9747676424058)) ;
#55032=CARTESIAN_POINT('Ctrl Pts',(-13.7208464424711,-16.0652608298864,
24.9595535677136)) ;
#55033=CARTESIAN_POINT('Ctrl Pts',(-13.6559658665551,-16.0735798722808,
24.9444642041659)) ;
#55034=CARTESIAN_POINT('Ctrl Pts',(-13.5899245738745,-16.0816680200507,
24.9312737800857)) ;
#55035=CARTESIAN_POINT('Ctrl Pts',(-13.5229961198868,-16.0894673869308,
24.9201489298451)) ;
#55036=CARTESIAN_POINT('Ctrl Pts',(-13.4680006593836,-16.0958761674666,
24.9110075822483)) ;
#55037=CARTESIAN_POINT('Ctrl Pts',(-13.4124067991456,-16.1020900207684,
24.9032601846009)) ;
#55038=CARTESIAN_POINT('Ctrl Pts',(-13.3563772644563,-16.1080799337539,
24.8969753865622)) ;
#55039=CARTESIAN_POINT('Ctrl Pts',(-13.286224994253,-16.1155796568301,24.8891064500695)) ;
#55040=CARTESIAN_POINT('Ctrl Pts',(-13.2153791230557,-16.1227292229208,
24.883530372851)) ;
#55041=CARTESIAN_POINT('Ctrl Pts',(-13.1441447360857,-16.1294814162036,
24.8803340060351)) ;
#55042=CARTESIAN_POINT('Ctrl Pts',(-13.0730511924442,-16.1362202591733,
24.8771439590173)) ;
#55043=CARTESIAN_POINT('Ctrl Pts',(-13.0015711634035,-16.1425632136358,
24.8763243184304)) ;
#55044=CARTESIAN_POINT('Ctrl Pts',(-12.9300176635963,-16.1484717649149,
24.8779111256775)) ;
#55045=CARTESIAN_POINT('Ctrl Pts',(-12.8760552577365,-16.1529277264406,
24.8791078237695)) ;
#55046=CARTESIAN_POINT('Ctrl Pts',(-12.8220513174348,-16.1571367885211,
24.8816721508341)) ;
#55047=CARTESIAN_POINT('Ctrl Pts',(-12.7681411399577,-16.1610860188908,
24.8856002845828)) ;
#55048=CARTESIAN_POINT('Ctrl Pts',(-12.6935628394831,-16.166549308068,24.8910343891013)) ;
#55049=CARTESIAN_POINT('Ctrl Pts',(-12.6191137743479,-16.171518536629,24.8990845407954)) ;
#55050=CARTESIAN_POINT('Ctrl Pts',(-12.5451491044039,-16.1759680067789,
24.9096990657516)) ;
#55051=CARTESIAN_POINT('Ctrl Pts',(-12.4711844345007,-16.1804174769264,
24.920313590702)) ;
#55052=CARTESIAN_POINT('Ctrl Pts',(-12.3977047751287,-16.184347145014,24.9334923330962)) ;
#55053=CARTESIAN_POINT('Ctrl Pts',(-12.3250531844235,-16.1877442734701,
24.9491244469266)) ;
#55054=CARTESIAN_POINT('',(-12.9635641336241,-15.9108618782028,26.2848388535279)) ;
#55055=CARTESIAN_POINT('Ctrl Pts',(-12.9635641336243,-15.9108618782028,
26.2848388535278)) ;
#55056=CARTESIAN_POINT('Ctrl Pts',(-12.6402810210044,-16.0510971579062,
25.6082760530286)) ;
#55057=CARTESIAN_POINT('Ctrl Pts',(-12.3250531847509,-16.1877442737199,
24.9491244468999)) ;
#55058=CARTESIAN_POINT('',(-11.6408731773057,-15.9108618782028,26.8967808533363)) ;
#55059=CARTESIAN_POINT('Origin',(-2.92277791062251E-15,-15.9108618782028,
0.)) ;
#55060=CARTESIAN_POINT('',(-11.0362055712307,-16.1877442736409,25.545408848944)) ;
#55061=CARTESIAN_POINT('Ctrl Pts',(-11.0362055710702,-16.1877442737199,
25.5454088490852)) ;
#55062=CARTESIAN_POINT('Ctrl Pts',(-11.3345117375303,-16.0510971572356,
26.2123892572703)) ;
#55063=CARTESIAN_POINT('Ctrl Pts',(-11.6408731773055,-15.9108618782028,
26.8967808533364)) ;
#55064=CARTESIAN_POINT('',(-9.82338358164157,-15.9108618855281,27.6124587235785)) ;
#55065=CARTESIAN_POINT('Ctrl Pts',(-11.0362055713025,-16.1877442734701,
25.5454088488529)) ;
#55066=CARTESIAN_POINT('Ctrl Pts',(-10.9772577239093,-16.184347145014,25.5906611184371)) ;
#55067=CARTESIAN_POINT('Ctrl Pts',(-10.9196436628343,-16.1804174769264,
25.6381327895575)) ;
#55068=CARTESIAN_POINT('Ctrl Pts',(-10.8636699618301,-16.1759680067789,
25.6876341565055)) ;
#55069=CARTESIAN_POINT('Ctrl Pts',(-10.8076962607951,-16.171518536629,25.7371355234807)) ;
#55070=CARTESIAN_POINT('Ctrl Pts',(-10.7533634369526,-16.166549308068,25.7886662181691)) ;
#55071=CARTESIAN_POINT('Ctrl Pts',(-10.7009407998154,-16.1610860188908,
25.8419890041916)) ;
#55072=CARTESIAN_POINT('Ctrl Pts',(-10.6507113260991,-16.155851292919,25.893080967993)) ;
#55073=CARTESIAN_POINT('Ctrl Pts',(-10.6022028799284,-16.1501596984485,
25.9458509090239)) ;
#55074=CARTESIAN_POINT('Ctrl Pts',(-10.5556213946471,-16.1440425621065,
26.0000604057616)) ;
#55075=CARTESIAN_POINT('Ctrl Pts',(-10.5089436728898,-16.1379127878753,
26.0543818983042)) ;
#55076=CARTESIAN_POINT('Ctrl Pts',(-10.4642011932089,-16.1313557844548,
26.1101484935574)) ;
#55077=CARTESIAN_POINT('Ctrl Pts',(-10.4215593171393,-16.1244124680044,
26.1670901111956)) ;
#55078=CARTESIAN_POINT('Ctrl Pts',(-10.3894279594871,-16.1191805644222,
26.2099965602139)) ;
#55079=CARTESIAN_POINT('Ctrl Pts',(-10.3584884508272,-16.1137295207043,
26.2535695036106)) ;
#55080=CARTESIAN_POINT('Ctrl Pts',(-10.3287944717036,-16.1080799337539,
26.2976843427492)) ;
#55081=CARTESIAN_POINT('Ctrl Pts',(-10.2905319447247,-16.1008000918638,
26.3545290389645)) ;
#55082=CARTESIAN_POINT('Ctrl Pts',(-10.254333906118,-16.0931892946347,26.4122822988833)) ;
#55083=CARTESIAN_POINT('Ctrl Pts',(-10.2202911754108,-16.0853002129684,
26.4706402522785)) ;
#55084=CARTESIAN_POINT('Ctrl Pts',(-10.1859708472133,-16.0773468007026,
26.529474078821)) ;
#55085=CARTESIAN_POINT('Ctrl Pts',(-10.1538412476587,-16.0691106491238,
26.5889220139178)) ;
#55086=CARTESIAN_POINT('Ctrl Pts',(-10.1239442393385,-16.0606518030577,
26.6486593488293)) ;
#55087=CARTESIAN_POINT('Ctrl Pts',(-10.0994604990071,-16.0537245483851,
26.6975804107763)) ;
#55088=CARTESIAN_POINT('Ctrl Pts',(-10.0764730903414,-16.0466480826284,
26.7466951934594)) ;
#55089=CARTESIAN_POINT('Ctrl Pts',(-10.0549792645758,-16.0394576303854,
26.7958222513128)) ;
#55090=CARTESIAN_POINT('Ctrl Pts',(-10.0286901692914,-16.0306629892537,
26.8559095488947)) ;
#55091=CARTESIAN_POINT('Ctrl Pts',(-10.003962443847,-16.0214720150687,26.9175567573472)) ;
#55092=CARTESIAN_POINT('Ctrl Pts',(-9.98104284872743,-16.0119118209662,
26.9805349789327)) ;
#55093=CARTESIAN_POINT('Ctrl Pts',(-9.95831097158325,-16.0024299275611,
27.0429973910465)) ;
#55094=CARTESIAN_POINT('Ctrl Pts',(-9.93735806149429,-15.9925848997544,
27.1067687415412)) ;
#55095=CARTESIAN_POINT('Ctrl Pts',(-9.91838482378365,-15.9824119250013,
27.1715951546544)) ;
#55096=CARTESIAN_POINT('Ctrl Pts',(-9.9028059128142,-15.974058903214,27.2248240728686)) ;
#55097=CARTESIAN_POINT('Ctrl Pts',(-9.88856104656038,-15.9654849570548,
27.2787636551505)) ;
#55098=CARTESIAN_POINT('Ctrl Pts',(-9.87573868735372,-15.9567135267634,
27.3332605475946)) ;
#55099=CARTESIAN_POINT('Ctrl Pts',(-9.85967516493002,-15.9457249040846,
27.4015328553414)) ;
#55100=CARTESIAN_POINT('Ctrl Pts',(-9.84584298147462,-15.9344245943129,
27.4706902623636)) ;
#55101=CARTESIAN_POINT('Ctrl Pts',(-9.83436617479649,-15.9228603613737,
27.5404409509933)) ;
#55102=CARTESIAN_POINT('Ctrl Pts',(-9.83042703709848,-15.9188912167155,
27.5643811962853)) ;
#55103=CARTESIAN_POINT('Ctrl Pts',(-9.82676495056885,-15.9148910348745,
27.588391181513)) ;
#55104=CARTESIAN_POINT('Ctrl Pts',(-9.82338358613012,-15.9108619063809,
27.61245868618)) ;
#55105=CARTESIAN_POINT('',(-8.89001990812047,-15.9108619763187,27.92694497988)) ;
#55106=CARTESIAN_POINT('Origin',(-2.92277791062251E-15,-15.9108618782028,
0.)) ;
#55107=CARTESIAN_POINT('',(-6.67357602500529,-16.1877442736409,27.0153498905465)) ;
#55108=CARTESIAN_POINT('Ctrl Pts',(-8.89002000637734,-15.9108620123611,
27.9269448892862)) ;
#55109=CARTESIAN_POINT('Ctrl Pts',(-8.83974141393214,-15.922601008379,27.8770836956966)) ;
#55110=CARTESIAN_POINT('Ctrl Pts',(-8.78785899221147,-15.9340938648278,
27.8290563925788)) ;
#55111=CARTESIAN_POINT('Ctrl Pts',(-8.73463808083946,-15.9452907435693,
27.7830349210544)) ;
#55112=CARTESIAN_POINT('Ctrl Pts',(-8.71637144205948,-15.9491337694432,
27.7672392953354)) ;
#55113=CARTESIAN_POINT('Ctrl Pts',(-8.69794738737287,-15.952941979252,27.7516795942054)) ;
#55114=CARTESIAN_POINT('Ctrl Pts',(-8.67937741285404,-15.9567135267634,
27.7363615946437)) ;
#55115=CARTESIAN_POINT('Ctrl Pts',(-8.62685013972879,-15.9673817754482,
27.6930329004715)) ;
#55116=CARTESIAN_POINT('Ctrl Pts',(-8.5731459765618,-15.977757691291,27.6516352149836)) ;
#55117=CARTESIAN_POINT('Ctrl Pts',(-8.51856061611486,-15.9877997661731,
27.6122877272514)) ;
#55118=CARTESIAN_POINT('Ctrl Pts',(-8.46353052263586,-15.997923658641,27.5726196567222)) ;
#55119=CARTESIAN_POINT('Ctrl Pts',(-8.4076052920716,-16.0077081692744,27.5350354983163)) ;
#55120=CARTESIAN_POINT('Ctrl Pts',(-8.35110780552667,-16.0171189356805,
27.4996086579324)) ;
#55121=CARTESIAN_POINT('Ctrl Pts',(-8.30487398406619,-16.0248200870136,
27.4706176653522)) ;
#55122=CARTESIAN_POINT('Ctrl Pts',(-8.25825743219905,-16.0322710948774,
27.4430704521203)) ;
#55123=CARTESIAN_POINT('Ctrl Pts',(-8.21144143306706,-16.0394576303853,
27.4169824693803)) ;
#55124=CARTESIAN_POINT('Ctrl Pts',(-8.15416038046395,-16.0482506141109,
27.3850628876275)) ;
#55125=CARTESIAN_POINT('Ctrl Pts',(-8.09511127805334,-16.056873031955,27.3545105324776)) ;
#55126=CARTESIAN_POINT('Ctrl Pts',(-8.03449445953493,-16.0652608298866,
27.3255894753811)) ;
#55127=CARTESIAN_POINT('Ctrl Pts',(-7.97437452255286,-16.0735798722811,
27.2969054868018)) ;
#55128=CARTESIAN_POINT('Ctrl Pts',(-7.91271278986576,-16.0816680200511,
27.2698265217467)) ;
#55129=CARTESIAN_POINT('Ctrl Pts',(-7.84974059989247,-16.0894673869313,
27.244574125106)) ;
#55130=CARTESIAN_POINT('Ctrl Pts',(-7.79799602221246,-16.095876167467,27.2238240987827)) ;
#55131=CARTESIAN_POINT('Ctrl Pts',(-7.74536737701679,-16.1020900207685,
27.204306794379)) ;
#55132=CARTESIAN_POINT('Ctrl Pts',(-7.69199882751462,-16.1080799337539,
27.1861242376894)) ;
#55133=CARTESIAN_POINT('Ctrl Pts',(-7.62517826714627,-16.1155796568301,
27.1633586081517)) ;
#55134=CARTESIAN_POINT('Ctrl Pts',(-7.55718742482217,-16.1227292229207,
27.1426831284015)) ;
#55135=CARTESIAN_POINT('Ctrl Pts',(-7.48830558261541,-16.1294814162036,
27.1242482033404)) ;
#55136=CARTESIAN_POINT('Ctrl Pts',(-7.41955993232838,-16.1362202591733,
27.1058497274763)) ;
#55137=CARTESIAN_POINT('Ctrl Pts',(-7.34992726514201,-16.1425632136358,
27.0896831563216)) ;
#55138=CARTESIAN_POINT('Ctrl Pts',(-7.27970552974461,-16.148471764915,27.0758509775448)) ;
#55139=CARTESIAN_POINT('Ctrl Pts',(-7.22674748023081,-16.1529277264407,
27.0654193753579)) ;
#55140=CARTESIAN_POINT('Ctrl Pts',(-7.17345486752508,-16.1571367885211,
27.0563144990611)) ;
#55141=CARTESIAN_POINT('Ctrl Pts',(-7.11996064739795,-16.1610860188908,
27.0485617006416)) ;
#55142=CARTESIAN_POINT('Ctrl Pts',(-7.04595777430401,-16.166549308068,27.037836628733)) ;
#55143=CARTESIAN_POINT('Ctrl Pts',(-6.97151874228637,-16.171518536629,27.0296942240487)) ;
#55144=CARTESIAN_POINT('Ctrl Pts',(-6.89700151612033,-16.1759680067789,
27.0241603696521)) ;
#55145=CARTESIAN_POINT('Ctrl Pts',(-6.82248428999535,-16.1804174769264,
27.0186265152585)) ;
#55146=CARTESIAN_POINT('Ctrl Pts',(-6.74788950417224,-16.184347145014,27.0157011912573)) ;
#55147=CARTESIAN_POINT('Ctrl Pts',(-6.6735760249974,-16.1877442734653,27.0153498905179)) ;
#55148=CARTESIAN_POINT('',(-7.01001982894532,-15.9108618782028,28.4570970163913)) ;
#55149=CARTESIAN_POINT('Ctrl Pts',(-7.01001982894662,-15.9108618782028,
28.457097016391)) ;
#55150=CARTESIAN_POINT('Ctrl Pts',(-6.83973590004788,-16.0510971569625,
27.7268555700758)) ;
#55151=CARTESIAN_POINT('Ctrl Pts',(-6.67357602521852,-16.1877442737199,
27.0153498905617)) ;
#55152=CARTESIAN_POINT('',(-5.58670321106903,-15.9108618782028,28.7703926951639)) ;
#55153=CARTESIAN_POINT('Origin',(-2.92277791062251E-15,-15.9108618782028,
0.)) ;
#55154=CARTESIAN_POINT('',(-5.28667743227751,-16.1877442736409,27.3206293558041)) ;
#55155=CARTESIAN_POINT('Ctrl Pts',(-5.28667743209039,-16.1877442737198,
27.3206293559074)) ;
#55156=CARTESIAN_POINT('Ctrl Pts',(-5.43462829436583,-16.0510971570733,
28.0361431415679)) ;
#55157=CARTESIAN_POINT('Ctrl Pts',(-5.58670321106773,-15.9108618782028,
28.7703926951642)) ;
#55158=CARTESIAN_POINT('',(-3.65785625118289,-15.9108619763187,29.0786312869383)) ;
#55159=CARTESIAN_POINT('Ctrl Pts',(-5.28667743236728,-16.1877442734701,
27.3206293557305)) ;
#55160=CARTESIAN_POINT('Ctrl Pts',(-5.21937985257516,-16.184347145014,27.3521516076954)) ;
#55161=CARTESIAN_POINT('Ctrl Pts',(-5.15290777019315,-16.1804174769264,
27.3861280974538)) ;
#55162=CARTESIAN_POINT('Ctrl Pts',(-5.08760137256953,-16.1759680067789,
27.4224394588058)) ;
#55163=CARTESIAN_POINT('Ctrl Pts',(-5.02229497490993,-16.171518536629,27.4587508201778)) ;
#55164=CARTESIAN_POINT('Ctrl Pts',(-4.95815484617409,-16.166549308068,27.4973968048012)) ;
#55165=CARTESIAN_POINT('Ctrl Pts',(-4.89549499837687,-16.1610860188908,
27.5382036163359)) ;
#55166=CARTESIAN_POINT('Ctrl Pts',(-4.83545659989313,-16.155851292919,27.5773032263399)) ;
#55167=CARTESIAN_POINT('Ctrl Pts',(-4.77673827678375,-16.1501596984485,
27.6184115534471)) ;
#55168=CARTESIAN_POINT('Ctrl Pts',(-4.7195924013649,-16.1440425621064,27.6613400198796)) ;
#55169=CARTESIAN_POINT('Ctrl Pts',(-4.66232846363785,-16.1379127878752,
27.7043571757196)) ;
#55170=CARTESIAN_POINT('Ctrl Pts',(-4.60664386873717,-16.1313557844547,
27.7492016684129)) ;
#55171=CARTESIAN_POINT('Ctrl Pts',(-4.55275817142329,-16.1244124680042,
27.7956452798039)) ;
#55172=CARTESIAN_POINT('Ctrl Pts',(-4.5121544088245,-16.119180564422,27.8306413077882)) ;
#55173=CARTESIAN_POINT('Ctrl Pts',(-4.47257135386096,-16.1137295207043,
27.8665444601852)) ;
#55174=CARTESIAN_POINT('Ctrl Pts',(-4.43408821707906,-16.108079933754,27.9032445911354)) ;
#55175=CARTESIAN_POINT('Ctrl Pts',(-4.38450031734832,-16.1008000918637,
27.9505349776748)) ;
#55176=CARTESIAN_POINT('Ctrl Pts',(-4.33673332505971,-16.0931892946345,
27.9991564901773)) ;
#55177=CARTESIAN_POINT('Ctrl Pts',(-4.29094125954683,-16.085300212968,28.0488318862468)) ;
#55178=CARTESIAN_POINT('Ctrl Pts',(-4.24477578795872,-16.0773468007022,
28.0989123545592)) ;
#55179=CARTESIAN_POINT('Ctrl Pts',(-4.20061781180921,-16.0691106491232,
28.1500635158098)) ;
#55180=CARTESIAN_POINT('Ctrl Pts',(-4.15857801774614,-16.0606518030571,
28.2019772519887)) ;
#55181=CARTESIAN_POINT('Ctrl Pts',(-4.12415011143668,-16.0537245483847,
28.244491286255)) ;
#55182=CARTESIAN_POINT('Ctrl Pts',(-4.09114190915792,-16.0466480826282,
28.2875161792511)) ;
#55183=CARTESIAN_POINT('Ctrl Pts',(-4.05958973184235,-16.0394576303854,
28.3308741366043)) ;
#55184=CARTESIAN_POINT('Ctrl Pts',(-4.02099826818466,-16.0306629892538,
28.3839052481734)) ;
#55185=CARTESIAN_POINT('Ctrl Pts',(-3.98359633568106,-16.0214720150688,
28.4387954491257)) ;
#55186=CARTESIAN_POINT('Ctrl Pts',(-3.94767413194106,-16.0119118209664,
28.4953742394354)) ;
#55187=CARTESIAN_POINT('Ctrl Pts',(-3.9120461412236,-16.0024299275614,28.5514896334282)) ;
#55188=CARTESIAN_POINT('Ctrl Pts',(-3.87787414324033,-15.9925848997548,
28.6092657888807)) ;
#55189=CARTESIAN_POINT('Ctrl Pts',(-3.84540872671965,-15.9824119250018,
28.6684979112166)) ;
#55190=CARTESIAN_POINT('Ctrl Pts',(-3.81875139805034,-15.9740589032143,
28.7171333615545)) ;
#55191=CARTESIAN_POINT('Ctrl Pts',(-3.79324415310512,-15.965484957055,28.766749641209)) ;
#55192=CARTESIAN_POINT('Ctrl Pts',(-3.76900635257193,-15.9567135267634,
28.8172159983899)) ;
#55193=CARTESIAN_POINT('Ctrl Pts',(-3.73864185824403,-15.9457249040552,
28.8804389552036)) ;
#55194=CARTESIAN_POINT('Ctrl Pts',(-3.71026626524916,-15.9344245942524,
28.9450059900909)) ;
#55195=CARTESIAN_POINT('Ctrl Pts',(-3.68406344363511,-15.9228603612808,
29.0106587723793)) ;
#55196=CARTESIAN_POINT('Ctrl Pts',(-3.67507003447375,-15.918891251378,29.0331923125605)) ;
#55197=CARTESIAN_POINT('Ctrl Pts',(-3.66633220267684,-15.914891104836,29.0558535177718)) ;
#55198=CARTESIAN_POINT('Ctrl Pts',(-3.65785616022794,-15.9108620121299,
29.0786312426591)) ;
#55199=CARTESIAN_POINT('',(-2.67870907039602,-15.9108618818335,29.1851206195401)) ;
#55200=CARTESIAN_POINT('Origin',(-2.92277791062251E-15,-15.9108618782028,
0.)) ;
#55201=CARTESIAN_POINT('',(-0.710049867689416,-16.1877442736409,27.8183675986852)) ;
#55202=CARTESIAN_POINT('Ctrl Pts',(-2.67870905771656,-15.9108618853164,
29.1851205952931)) ;
#55203=CARTESIAN_POINT('Ctrl Pts',(-2.6403246466816,-15.9226008834121,29.1256167055889)) ;
#55204=CARTESIAN_POINT('Ctrl Pts',(-2.59997966993281,-15.9340937421158,
29.0675590543327)) ;
#55205=CARTESIAN_POINT('Ctrl Pts',(-2.55789630122123,-15.945290623265,29.0111726030762)) ;
#55206=CARTESIAN_POINT('Ctrl Pts',(-2.54345217246438,-15.9491336899668,
28.9918192768804)) ;
#55207=CARTESIAN_POINT('Ctrl Pts',(-2.52880358691511,-15.9529419398965,
28.9726625237371)) ;
#55208=CARTESIAN_POINT('Ctrl Pts',(-2.51396053030637,-15.9567135267635,
28.9537104571357)) ;
#55209=CARTESIAN_POINT('Ctrl Pts',(-2.47197570409715,-15.9673817754481,
28.9001029527286)) ;
#55210=CARTESIAN_POINT('Ctrl Pts',(-2.42842639309452,-15.9777576912908,
28.8481283145256)) ;
#55211=CARTESIAN_POINT('Ctrl Pts',(-2.38357575480059,-15.9877997661729,
28.7979665102268)) ;
#55212=CARTESIAN_POINT('Ctrl Pts',(-2.33835969691063,-15.9979236586407,
28.7473960137229)) ;
#55213=CARTESIAN_POINT('Ctrl Pts',(-2.29182145023647,-16.0077081692741,
28.6986682806216)) ;
#55214=CARTESIAN_POINT('Ctrl Pts',(-2.24426056700373,-16.0171189356801,
28.6519244105256)) ;
#55215=CARTESIAN_POINT('Ctrl Pts',(-2.20533987303285,-16.0248200870134,
28.6136723062887)) ;
#55216=CARTESIAN_POINT('Ctrl Pts',(-2.16573502679743,-16.0322710948773,
28.5767479509172)) ;
#55217=CARTESIAN_POINT('Ctrl Pts',(-2.12562170484212,-16.0394576303854,
28.5412058347734)) ;
#55218=CARTESIAN_POINT('Ctrl Pts',(-2.07654161795819,-16.0482506141109,
28.4977187820102)) ;
#55219=CARTESIAN_POINT('Ctrl Pts',(-2.02544090398406,-16.0568730319549,
28.4551869124065)) ;
#55220=CARTESIAN_POINT('Ctrl Pts',(-1.9724584453729,-16.0652608298865,28.4139111893922)) ;
#55221=CARTESIAN_POINT('Ctrl Pts',(-1.9199102887603,-16.0735798722809,28.3729738072076)) ;
#55222=CARTESIAN_POINT('Ctrl Pts',(-1.86551135015594,-16.0816680200509,
28.3332724834876)) ;
#55223=CARTESIAN_POINT('Ctrl Pts',(-1.80943993381238,-16.0894673869311,
28.2950733144478)) ;
#55224=CARTESIAN_POINT('Ctrl Pts',(-1.76336575789626,-16.0958761674669,
28.2636848575662)) ;
#55225=CARTESIAN_POINT('Ctrl Pts',(-1.71616318469793,-16.1020900207685,
28.2333102538678)) ;
#55226=CARTESIAN_POINT('Ctrl Pts',(-1.66795107444097,-16.108079933754,28.2040801346692)) ;
#55227=CARTESIAN_POINT('Ctrl Pts',(-1.60758667904453,-16.1155796568301,
28.1674823076214)) ;
#55228=CARTESIAN_POINT('Ctrl Pts',(-1.54563004181418,-16.1227292229208,
28.1326741877935)) ;
#55229=CARTESIAN_POINT('Ctrl Pts',(-1.48232158275546,-16.1294814162036,
28.0998627010941)) ;
#55230=CARTESIAN_POINT('Ctrl Pts',(-1.41913829602524,-16.1362202591733,
28.0671160886667)) ;
#55231=CARTESIAN_POINT('Ctrl Pts',(-1.35460893682001,-16.1425632136358,
28.0363585178435)) ;
#55232=CARTESIAN_POINT('Ctrl Pts',(-1.28900245613401,-16.148471764915,28.0077541303492)) ;
#55233=CARTESIAN_POINT('Ctrl Pts',(-1.23952502250277,-16.1529277264407,
27.9861819980077)) ;
#55234=CARTESIAN_POINT('Ctrl Pts',(-1.18943564073249,-16.1571367885211,
27.9658336522457)) ;
#55235=CARTESIAN_POINT('Ctrl Pts',(-1.13885870823377,-16.1610860188908,
27.9467624338955)) ;
#55236=CARTESIAN_POINT('Ctrl Pts',(-1.06889155461827,-16.166549308068,27.9203796780022)) ;
#55237=CARTESIAN_POINT('Ctrl Pts',(-0.997943242122202,-16.171518536629,
27.896425446733)) ;
#55238=CARTESIAN_POINT('Ctrl Pts',(-0.926357802409802,-16.1759680067789,
27.8750019698647)) ;
#55239=CARTESIAN_POINT('Ctrl Pts',(-0.854772362736824,-16.1804174769264,
27.8535784930083)) ;
#55240=CARTESIAN_POINT('Ctrl Pts',(-0.782550419741656,-16.1843471450139,
27.8346858875108)) ;
#55241=CARTESIAN_POINT('Ctrl Pts',(-0.71004986758597,-16.1877442734701,
27.8183675986327)) ;
#55242=CARTESIAN_POINT('',(-0.72869478814225,-15.9108618782028,29.2987329505603)) ;
#55243=CARTESIAN_POINT('Ctrl Pts',(-0.72869478814245,-15.9108618782028,
29.2987329505603)) ;
#55244=CARTESIAN_POINT('Ctrl Pts',(-0.719372328009428,-16.0510971575387,
28.5489581292205)) ;
#55245=CARTESIAN_POINT('Ctrl Pts',(-0.710049867894285,-16.1877442737198,
27.818367598746)) ;
#55246=CARTESIAN_POINT('',(0.728694788142244,-15.9108618782028,29.2987329505603)) ;
#55247=CARTESIAN_POINT('Origin',(-2.92277791062251E-15,-15.9108618782028,
0.)) ;
#55248=CARTESIAN_POINT('',(0.710049867689371,-16.1877442736409,27.8183675986852)) ;
#55249=CARTESIAN_POINT('Ctrl Pts',(0.710049867894279,-16.1877442737198,
27.818367598746)) ;
#55250=CARTESIAN_POINT('Ctrl Pts',(0.71937232800943,-16.0510971575386,28.548958129221)) ;
#55251=CARTESIAN_POINT('Ctrl Pts',(0.728694788142444,-15.9108618782028,
29.2987329505603)) ;
#55252=CARTESIAN_POINT('',(2.67870907039602,-15.9108618818335,29.1851206195401)) ;
#55253=CARTESIAN_POINT('Ctrl Pts',(0.710049867585909,-16.1877442734701,
27.8183675986327)) ;
#55254=CARTESIAN_POINT('Ctrl Pts',(0.782550419741599,-16.1843471450139,
27.8346858875108)) ;
#55255=CARTESIAN_POINT('Ctrl Pts',(0.854772362736772,-16.1804174769264,
27.8535784930083)) ;
#55256=CARTESIAN_POINT('Ctrl Pts',(0.926357802409753,-16.1759680067789,
27.8750019698647)) ;
#55257=CARTESIAN_POINT('Ctrl Pts',(0.99794324212217,-16.171518536629,27.8964254467329)) ;
#55258=CARTESIAN_POINT('Ctrl Pts',(1.06889155461827,-16.166549308068,27.9203796780022)) ;
#55259=CARTESIAN_POINT('Ctrl Pts',(1.13885870823377,-16.1610860188908,27.9467624338955)) ;
#55260=CARTESIAN_POINT('Ctrl Pts',(1.20589870269909,-16.155851292919,27.9720414357938)) ;
#55261=CARTESIAN_POINT('Ctrl Pts',(1.27208129921876,-16.1501596984486,27.9995659692902)) ;
#55262=CARTESIAN_POINT('Ctrl Pts',(1.33711948715304,-16.1440425621066,28.029206118038)) ;
#55263=CARTESIAN_POINT('Ctrl Pts',(1.40229204276538,-16.1379127878754,28.0589075027779)) ;
#55264=CARTESIAN_POINT('Ctrl Pts',(1.46631500311679,-16.1313557844549,28.0907330142736)) ;
#55265=CARTESIAN_POINT('Ctrl Pts',(1.52892488635768,-16.1244124680045,28.1245069677666)) ;
#55266=CARTESIAN_POINT('Ctrl Pts',(1.57610246709302,-16.1191805644222,28.1499561993445)) ;
#55267=CARTESIAN_POINT('Ctrl Pts',(1.62247820870467,-16.1137295207044,28.1765107692402)) ;
#55268=CARTESIAN_POINT('Ctrl Pts',(1.66795107444096,-16.108079933754,28.2040801346692)) ;
#55269=CARTESIAN_POINT('Ctrl Pts',(1.72654567184455,-16.1008000918637,28.2396049656167)) ;
#55270=CARTESIAN_POINT('Ctrl Pts',(1.78364808634439,-16.0931892946345,28.2768212428165)) ;
#55271=CARTESIAN_POINT('Ctrl Pts',(1.83904830057331,-16.0853002129681,28.3154913152495)) ;
#55272=CARTESIAN_POINT('Ctrl Pts',(1.89490026940932,-16.0773468007023,28.354476718293)) ;
#55273=CARTESIAN_POINT('Ctrl Pts',(1.94902184426688,-16.0691106491233,28.3949393342471)) ;
#55274=CARTESIAN_POINT('Ctrl Pts',(2.00123869002606,-16.0606518030571,28.4366020430871)) ;
#55275=CARTESIAN_POINT('Ctrl Pts',(2.04400095167941,-16.0537245483847,28.4707211406828)) ;
#55276=CARTESIAN_POINT('Ctrl Pts',(2.08548652071937,-16.0466480826282,28.5056443478157)) ;
#55277=CARTESIAN_POINT('Ctrl Pts',(2.12562170484212,-16.0394576303854,28.5412058347734)) ;
#55278=CARTESIAN_POINT('Ctrl Pts',(2.17471104292392,-16.0306629892538,28.5847010844929)) ;
#55279=CARTESIAN_POINT('Ctrl Pts',(2.22303830969206,-16.0214720150689,28.6302676731548)) ;
#55280=CARTESIAN_POINT('Ctrl Pts',(2.27028343973035,-16.0119118209665,28.677801470837)) ;
#55281=CARTESIAN_POINT('Ctrl Pts',(2.31714161877286,-16.0024299275614,28.7249459532537)) ;
#55282=CARTESIAN_POINT('Ctrl Pts',(2.36293486000431,-15.9925848997548,28.7740253648491)) ;
#55283=CARTESIAN_POINT('Ctrl Pts',(2.40737440854123,-15.9824119250019,28.8248935681996)) ;
#55284=CARTESIAN_POINT('Ctrl Pts',(2.44386368784915,-15.9740589032144,28.866661411057)) ;
#55285=CARTESIAN_POINT('Ctrl Pts',(2.47944062106131,-15.965484957055,28.9096343859912)) ;
#55286=CARTESIAN_POINT('Ctrl Pts',(2.5139605303064,-15.9567135267634,28.9537104571357)) ;
#55287=CARTESIAN_POINT('Ctrl Pts',(2.55720618635062,-15.9457249040902,29.0089278274643)) ;
#55288=CARTESIAN_POINT('Ctrl Pts',(2.59879837753547,-15.9344245943244,29.0658854070521)) ;
#55289=CARTESIAN_POINT('Ctrl Pts',(2.63850199913644,-15.9228603613915,29.1243704314812)) ;
#55290=CARTESIAN_POINT('Ctrl Pts',(2.65212933554176,-15.9188912098105,29.1444440436715)) ;
#55291=CARTESIAN_POINT('Ctrl Pts',(2.66553450938055,-15.9148910209383,29.1646972815063)) ;
#55292=CARTESIAN_POINT('Ctrl Pts',(2.67870905771655,-15.9108618853164,29.1851205952931)) ;
#55293=CARTESIAN_POINT('',(3.65785625118284,-15.9108619763187,29.0786312869383)) ;
#55294=CARTESIAN_POINT('Origin',(-2.92277791062251E-15,-15.9108618782028,
0.)) ;
#55295=CARTESIAN_POINT('',(5.28667743227854,-16.1877442736409,27.3206293558036)) ;
#55296=CARTESIAN_POINT('Ctrl Pts',(3.65785616022789,-15.9108620121299,29.0786312426591)) ;
#55297=CARTESIAN_POINT('Ctrl Pts',(3.68255160322085,-15.9226010082282,29.0122670155031)) ;
#55298=CARTESIAN_POINT('Ctrl Pts',(3.70947267289441,-15.9340938647544,28.9468937518395)) ;
#55299=CARTESIAN_POINT('Ctrl Pts',(3.7384507497277,-15.9452907435695,28.8827789144254)) ;
#55300=CARTESIAN_POINT('Ctrl Pts',(3.74839669099248,-15.9491337694433,28.860773230239)) ;
#55301=CARTESIAN_POINT('Ctrl Pts',(3.75858456122854,-15.9529419792521,28.838915568187)) ;
#55302=CARTESIAN_POINT('Ctrl Pts',(3.76900635257187,-15.9567135267634,28.8172159983899)) ;
#55303=CARTESIAN_POINT('Ctrl Pts',(3.79848556805471,-15.9673817754481,28.7558363110733)) ;
#55304=CARTESIAN_POINT('Ctrl Pts',(3.82984370951264,-15.9777576912908,28.6957149964714)) ;
#55305=CARTESIAN_POINT('Ctrl Pts',(3.86286245965529,-15.9877997661729,28.6370843858239)) ;
#55306=CARTESIAN_POINT('Ctrl Pts',(3.89615022934365,-15.9979236586407,28.5779760835566)) ;
#55307=CARTESIAN_POINT('Ctrl Pts',(3.93112541543707,-16.0077081692741,28.5203832304025)) ;
#55308=CARTESIAN_POINT('Ctrl Pts',(3.96752580131824,-16.0171189356801,28.4645080220079)) ;
#55309=CARTESIAN_POINT('Ctrl Pts',(3.99731347940591,-16.0248200870134,28.4187834319947)) ;
#55310=CARTESIAN_POINT('Ctrl Pts',(4.02805474141638,-16.0322710948773,28.3742084763029)) ;
#55311=CARTESIAN_POINT('Ctrl Pts',(4.05958973184228,-16.0394576303853,28.3308741366044)) ;
#55312=CARTESIAN_POINT('Ctrl Pts',(4.09817392269338,-16.0482506141109,28.2778530190853)) ;
#55313=CARTESIAN_POINT('Ctrl Pts',(4.13893683564045,-16.056873031955,28.2253303779792)) ;
#55314=CARTESIAN_POINT('Ctrl Pts',(4.18180753346602,-16.0652608298866,28.1736299959803)) ;
#55315=CARTESIAN_POINT('Ctrl Pts',(4.22432681630937,-16.0735798722811,28.1223534066824)) ;
#55316=CARTESIAN_POINT('Ctrl Pts',(4.26891932692231,-16.0816680200511,28.0718861140696)) ;
#55317=CARTESIAN_POINT('Ctrl Pts',(4.31546813252718,-16.0894673869313,28.0225263233196)) ;
#55318=CARTESIAN_POINT('Ctrl Pts',(4.35371752942058,-16.0958761674669,27.9819671252383)) ;
#55319=CARTESIAN_POINT('Ctrl Pts',(4.39328689075978,-16.1020900207685,27.9421555049558)) ;
#55320=CARTESIAN_POINT('Ctrl Pts',(4.43408821707899,-16.1080799337539,27.9032445911354)) ;
#55321=CARTESIAN_POINT('Ctrl Pts',(4.48517387546492,-16.1155796568301,27.8545258402948)) ;
#55322=CARTESIAN_POINT('Ctrl Pts',(4.53819928410433,-16.1227292229207,27.8072126693859)) ;
#55323=CARTESIAN_POINT('Ctrl Pts',(4.59297412683163,-16.1294814162036,27.761558849699)) ;
#55324=CARTESIAN_POINT('Ctrl Pts',(4.64764066974046,-16.1362202591732,27.7159952959104)) ;
#55325=CARTESIAN_POINT('Ctrl Pts',(4.70404939984709,-16.1425632136357,27.6720849152461)) ;
#55326=CARTESIAN_POINT('Ctrl Pts',(4.76197293970087,-16.1484717649149,27.6300458284021)) ;
#55327=CARTESIAN_POINT('Ctrl Pts',(4.80565624764355,-16.1529277264406,27.5983418548384)) ;
#55328=CARTESIAN_POINT('Ctrl Pts',(4.85020027465751,-16.1571367885211,27.5677015056432)) ;
#55329=CARTESIAN_POINT('Ctrl Pts',(4.89549499837679,-16.1610860188908,27.538203616336)) ;
#55330=CARTESIAN_POINT('Ctrl Pts',(4.95815484617414,-16.166549308068,27.4973968048011)) ;
#55331=CARTESIAN_POINT('Ctrl Pts',(5.02229497491018,-16.171518536629,27.4587508201776)) ;
#55332=CARTESIAN_POINT('Ctrl Pts',(5.08760137256992,-16.1759680067789,27.4224394588056)) ;
#55333=CARTESIAN_POINT('Ctrl Pts',(5.1529077701937,-16.1804174769265,27.3861280974535)) ;
#55334=CARTESIAN_POINT('Ctrl Pts',(5.21937985257595,-16.184347145014,27.352151607695)) ;
#55335=CARTESIAN_POINT('Ctrl Pts',(5.28667743236823,-16.1877442734702,27.32062935573)) ;
#55336=CARTESIAN_POINT('',(5.58670321107024,-15.9108618782028,28.7703926951637)) ;
#55337=CARTESIAN_POINT('Ctrl Pts',(5.58670321107023,-15.9108618782028,28.7703926951638)) ;
#55338=CARTESIAN_POINT('Ctrl Pts',(5.43462829348381,-16.0510971578892,28.0361431372959)) ;
#55339=CARTESIAN_POINT('Ctrl Pts',(5.2866774320916,-16.1877442737199,27.3206293559071)) ;
#55340=CARTESIAN_POINT('',(7.01001982894394,-15.9108618782028,28.4570970163916)) ;
#55341=CARTESIAN_POINT('Origin',(-2.92277791062251E-15,-15.9108618782028,
0.)) ;
#55342=CARTESIAN_POINT('',(6.67357602500404,-16.1877442736409,27.0153498905466)) ;
#55343=CARTESIAN_POINT('Ctrl Pts',(6.67357602521708,-16.1877442737199,27.015349890562)) ;
#55344=CARTESIAN_POINT('Ctrl Pts',(6.83973589941515,-16.0510971574815,27.726855567374)) ;
#55345=CARTESIAN_POINT('Ctrl Pts',(7.01001982894397,-15.9108618782028,28.4570970163916)) ;
#55346=CARTESIAN_POINT('',(8.89001990812046,-15.9108619763187,27.92694497988)) ;
#55347=CARTESIAN_POINT('Ctrl Pts',(6.67357602499615,-16.1877442734654,27.0153498905179)) ;
#55348=CARTESIAN_POINT('Ctrl Pts',(6.74788950417132,-16.184347145014,27.0157011912573)) ;
#55349=CARTESIAN_POINT('Ctrl Pts',(6.82248428999461,-16.1804174769264,27.0186265152585)) ;
#55350=CARTESIAN_POINT('Ctrl Pts',(6.89700151611982,-16.1759680067789,27.024160369652)) ;
#55351=CARTESIAN_POINT('Ctrl Pts',(6.97151874228602,-16.171518536629,27.0296942240486)) ;
#55352=CARTESIAN_POINT('Ctrl Pts',(7.04595777430382,-16.166549308068,27.0378366287329)) ;
#55353=CARTESIAN_POINT('Ctrl Pts',(7.1199606473979,-16.1610860188908,27.0485617006416)) ;
#55354=CARTESIAN_POINT('Ctrl Pts',(7.19086752221375,-16.155851292919,27.0588380764014)) ;
#55355=CARTESIAN_POINT('Ctrl Pts',(7.26141976748762,-16.1501596984485,27.0714917996922)) ;
#55356=CARTESIAN_POINT('Ctrl Pts',(7.33130915455475,-16.1440425621065,27.0864576903428)) ;
#55357=CARTESIAN_POINT('Ctrl Pts',(7.40134293178645,-16.1379127878753,27.1014545002433)) ;
#55358=CARTESIAN_POINT('Ctrl Pts',(7.47071061511937,-16.1313557844548,27.1187729049957)) ;
#55359=CARTESIAN_POINT('Ctrl Pts',(7.53911711573318,-16.1244124680043,27.1382979680627)) ;
#55360=CARTESIAN_POINT('Ctrl Pts',(7.59066254336305,-16.1191805644221,27.1530104254499)) ;
#55361=CARTESIAN_POINT('Ctrl Pts',(7.6416624934871,-16.1137295207043,27.1689747506686)) ;
#55362=CARTESIAN_POINT('Ctrl Pts',(7.69199882751456,-16.1080799337539,27.1861242376894)) ;
#55363=CARTESIAN_POINT('Ctrl Pts',(7.75686030433953,-16.1008000918637,27.208222411433)) ;
#55364=CARTESIAN_POINT('Ctrl Pts',(7.82062809561323,-16.0931892946345,27.2322932615711)) ;
#55365=CARTESIAN_POINT('Ctrl Pts',(7.88304600611371,-16.0853002129681,27.2581498407593)) ;
#55366=CARTESIAN_POINT('Ctrl Pts',(7.94597289620977,-16.0773468007023,27.2842172644169)) ;
#55367=CARTESIAN_POINT('Ctrl Pts',(8.00752740508663,-16.0691106491234,27.3120993481233)) ;
#55368=CARTESIAN_POINT('Ctrl Pts',(8.06747970086894,-16.0606518030573,27.3415629276636)) ;
#55369=CARTESIAN_POINT('Ctrl Pts',(8.1165768020383,-16.0537245483848,27.3656917175059)) ;
#55370=CARTESIAN_POINT('Ctrl Pts',(8.16459991873938,-16.0466480826282,27.3908802684245)) ;
#55371=CARTESIAN_POINT('Ctrl Pts',(8.21144143306702,-16.0394576303854,27.4169824693804)) ;
#55372=CARTESIAN_POINT('Ctrl Pts',(8.26873328268348,-16.0306629892538,27.4489080677152)) ;
#55373=CARTESIAN_POINT('Ctrl Pts',(8.32572615443434,-16.0214720150688,27.4830204010448)) ;
#55374=CARTESIAN_POINT('Ctrl Pts',(8.3820850809998,-16.0119118209664,27.5192865785502)) ;
#55375=CARTESIAN_POINT('Ctrl Pts',(8.43798241199483,-16.0024299275613,27.5552557257907)) ;
#55376=CARTESIAN_POINT('Ctrl Pts',(8.49325565541029,-15.9925848997546,27.5933434947909)) ;
#55377=CARTESIAN_POINT('Ctrl Pts',(8.54759139206526,-15.9824119250015,27.6334692385036)) ;
#55378=CARTESIAN_POINT('Ctrl Pts',(8.59220642386558,-15.9740589032141,27.6664164559697)) ;
#55379=CARTESIAN_POINT('Ctrl Pts',(8.63618950748789,-15.9654849570549,27.700736757636)) ;
#55380=CARTESIAN_POINT('Ctrl Pts',(8.67937741285401,-15.9567135267634,27.7363615946437)) ;
#55381=CARTESIAN_POINT('Ctrl Pts',(8.73348211207143,-15.9457249040552,27.7809914759642)) ;
#55382=CARTESIAN_POINT('Ctrl Pts',(8.78634609706161,-15.9344245942523,27.8276763275003)) ;
#55383=CARTESIAN_POINT('Ctrl Pts',(8.83769402165478,-15.9228603612807,27.8762588997127)) ;
#55384=CARTESIAN_POINT('Ctrl Pts',(8.85531780635308,-15.9188912514538,27.8929335520875)) ;
#55385=CARTESIAN_POINT('Ctrl Pts',(8.87276324047922,-15.914891104989,27.909831384247)) ;
#55386=CARTESIAN_POINT('Ctrl Pts',(8.89002000637735,-15.9108620123611,27.9269448892862)) ;
#55387=CARTESIAN_POINT('',(9.82338358164146,-15.9108618855281,27.6124587235785)) ;
#55388=CARTESIAN_POINT('Origin',(-2.92277791062251E-15,-15.9108618782028,
0.)) ;
#55389=CARTESIAN_POINT('',(11.0362055712312,-16.1877442736409,25.5454088489437)) ;
#55390=CARTESIAN_POINT('Ctrl Pts',(9.82338358613002,-15.9108619063809,27.61245868618)) ;
#55391=CARTESIAN_POINT('Ctrl Pts',(9.83323530215201,-15.922600904189,27.5423372231927)) ;
#55392=CARTESIAN_POINT('Ctrl Pts',(9.84547363914043,-15.9340937625734,27.4727051106785)) ;
#55393=CARTESIAN_POINT('Ctrl Pts',(9.85999141653387,-15.9452906433748,27.4038598065403)) ;
#55394=CARTESIAN_POINT('Ctrl Pts',(9.86497429424729,-15.9491337032519,27.3802303126882)) ;
#55395=CARTESIAN_POINT('Ctrl Pts',(9.8702252698575,-15.952941946475,27.3566933742252)) ;
#55396=CARTESIAN_POINT('Ctrl Pts',(9.87573868735361,-15.9567135267634,27.3332605475947)) ;
#55397=CARTESIAN_POINT('Ctrl Pts',(9.89133387675787,-15.9673817754481,27.2669787233288)) ;
#55398=CARTESIAN_POINT('Ctrl Pts',(9.90903457682846,-15.9777576912908,27.2015219381791)) ;
#55399=CARTESIAN_POINT('Ctrl Pts',(9.92867751876087,-15.9877997661728,27.1371640233736)) ;
#55400=CARTESIAN_POINT('Ctrl Pts',(9.94848050113368,-15.9979236586406,27.0722817538628)) ;
#55401=CARTESIAN_POINT('Ctrl Pts',(9.9702572258167,-16.007708169274,27.0085167584596)) ;
#55402=CARTESIAN_POINT('Ctrl Pts',(9.99379507275848,-16.01711893568,26.9461228744104)) ;
#55403=CARTESIAN_POINT('Ctrl Pts',(10.0130568962422,-16.0248200870133,26.8950638296305)) ;
#55404=CARTESIAN_POINT('Ctrl Pts',(10.0334971467828,-16.0322710948773,26.8449225490046)) ;
#55405=CARTESIAN_POINT('Ctrl Pts',(10.0549792645757,-16.0394576303854,26.7958222513128)) ;
#55406=CARTESIAN_POINT('Ctrl Pts',(10.0812634055125,-16.0482506141108,26.7357462775652)) ;
#55407=CARTESIAN_POINT('Ctrl Pts',(10.1097824889273,-16.0568730319548,26.6756887652808)) ;
#55408=CARTESIAN_POINT('Ctrl Pts',(10.1405368397836,-16.0652608298864,26.6159811766996)) ;
#55409=CARTESIAN_POINT('Ctrl Pts',(10.1710390944484,-16.0735798722808,26.5567630166145)) ;
#55410=CARTESIAN_POINT('Ctrl Pts',(10.2037400808343,-16.0816680200508,26.4978895496216)) ;
#55411=CARTESIAN_POINT('Ctrl Pts',(10.2385897052852,-16.089467386931,26.4396771461177)) ;
#55412=CARTESIAN_POINT('Ctrl Pts',(10.2672258238691,-16.0958761674667,26.3918437098595)) ;
#55413=CARTESIAN_POINT('Ctrl Pts',(10.2973117539923,-16.1020900207684,26.3444566201085)) ;
#55414=CARTESIAN_POINT('Ctrl Pts',(10.3287944717035,-16.1080799337539,26.2976843427491)) ;
#55415=CARTESIAN_POINT('Ctrl Pts',(10.3682126844706,-16.1155796568301,26.2391227027578)) ;
#55416=CARTESIAN_POINT('Ctrl Pts',(10.4098274553449,-16.1227292229208,26.1815167920545)) ;
#55417=CARTESIAN_POINT('Ctrl Pts',(10.4535074709729,-16.1294814162037,26.1251553612478)) ;
#55418=CARTESIAN_POINT('Ctrl Pts',(10.497101123272,-16.1362202591734,26.0689053672325)) ;
#55419=CARTESIAN_POINT('Ctrl Pts',(10.5427516147545,-16.1425632136358,26.0138953773238)) ;
#55420=CARTESIAN_POINT('Ctrl Pts',(10.5902837734305,-16.148471764915,25.9603872921075)) ;
#55421=CARTESIAN_POINT('Ctrl Pts',(10.626130372755,-16.1529277264407,25.9200339198896)) ;
#55422=CARTESIAN_POINT('Ctrl Pts',(10.6630462158159,-16.1571367885211,25.8805342759359)) ;
#55423=CARTESIAN_POINT('Ctrl Pts',(10.7009407998153,-16.1610860188908,25.8419890041916)) ;
#55424=CARTESIAN_POINT('Ctrl Pts',(10.7533634369525,-16.166549308068,25.7886662181691)) ;
#55425=CARTESIAN_POINT('Ctrl Pts',(10.8076962607951,-16.171518536629,25.7371355234806)) ;
#55426=CARTESIAN_POINT('Ctrl Pts',(10.8636699618301,-16.1759680067789,25.6876341565054)) ;
#55427=CARTESIAN_POINT('Ctrl Pts',(10.9196436628344,-16.1804174769265,25.6381327895573)) ;
#55428=CARTESIAN_POINT('Ctrl Pts',(10.9772577239095,-16.184347145014,25.5906611184369)) ;
#55429=CARTESIAN_POINT('Ctrl Pts',(11.0362055713028,-16.1877442734702,25.5454088488525)) ;
#55430=CARTESIAN_POINT('',(11.6408731773052,-15.9108618782029,26.8967808533365)) ;
#55431=CARTESIAN_POINT('Ctrl Pts',(11.6408731773062,-15.9108618782028,26.8967808533361)) ;
#55432=CARTESIAN_POINT('Ctrl Pts',(11.3345117375673,-16.051097157219,26.2123892573509)) ;
#55433=CARTESIAN_POINT('Ctrl Pts',(11.0362055710711,-16.1877442737198,25.5454088490849)) ;
#55434=CARTESIAN_POINT('',(12.9635641336247,-15.9108618782029,26.2848388535276)) ;
#55435=CARTESIAN_POINT('Origin',(-2.92277791062251E-15,-15.9108618782028,
0.)) ;
#55436=CARTESIAN_POINT('',(12.325053184539,-16.1877442736409,24.9491244469311)) ;
#55437=CARTESIAN_POINT('Ctrl Pts',(12.3250531847502,-16.1877442737198,24.9491244469006)) ;
#55438=CARTESIAN_POINT('Ctrl Pts',(12.6402810223916,-16.0510971573044,25.6082760559321)) ;
#55439=CARTESIAN_POINT('Ctrl Pts',(12.9635641336236,-15.9108618782028,26.2848388535281)) ;
#55440=CARTESIAN_POINT('',(14.6856444869838,-15.9108618855281,25.36293728564)) ;
#55441=CARTESIAN_POINT('Ctrl Pts',(12.3250531844232,-16.1877442734702,24.9491244469267)) ;
#55442=CARTESIAN_POINT('Ctrl Pts',(12.3977047751286,-16.184347145014,24.9334923330962)) ;
#55443=CARTESIAN_POINT('Ctrl Pts',(12.4711844345007,-16.1804174769265,24.920313590702)) ;
#55444=CARTESIAN_POINT('Ctrl Pts',(12.545149104404,-16.1759680067789,24.9096990657516)) ;
#55445=CARTESIAN_POINT('Ctrl Pts',(12.6191137743479,-16.171518536629,24.8990845407954)) ;
#55446=CARTESIAN_POINT('Ctrl Pts',(12.693562839483,-16.1665493080681,24.8910343891013)) ;
#55447=CARTESIAN_POINT('Ctrl Pts',(12.7681411399577,-16.1610860188908,24.8856002845829)) ;
#55448=CARTESIAN_POINT('Ctrl Pts',(12.8395993684648,-16.155851292919,24.8803935222949)) ;
#55449=CARTESIAN_POINT('Ctrl Pts',(12.9112223179169,-16.1501596984485,24.8775847613426)) ;
#55450=CARTESIAN_POINT('Ctrl Pts',(12.982694954054,-16.1440425621065,24.8771766054826)) ;
#55451=CARTESIAN_POINT('Ctrl Pts',(13.0543152513185,-16.1379127878753,24.8767676063803)) ;
#55452=CARTESIAN_POINT('Ctrl Pts',(13.1257841018569,-16.1313557844548,24.8787691150311)) ;
#55453=CARTESIAN_POINT('Ctrl Pts',(13.1967886079032,-16.1244124680043,24.8831323174237)) ;
#55454=CARTESIAN_POINT('Ctrl Pts',(13.2502916755205,-16.1191805644221,24.8864200624646)) ;
#55455=CARTESIAN_POINT('Ctrl Pts',(13.3035311331718,-16.1137295207043,24.8910476689023)) ;
#55456=CARTESIAN_POINT('Ctrl Pts',(13.3563772644564,-16.1080799337539,24.8969753865622)) ;
#55457=CARTESIAN_POINT('Ctrl Pts',(13.4244727701354,-16.1008000918637,24.9046136170581)) ;
#55458=CARTESIAN_POINT('Ctrl Pts',(13.4919242271365,-16.0931892946344,24.9144135139351)) ;
#55459=CARTESIAN_POINT('Ctrl Pts',(13.5584412417866,-16.0853002129679,24.9262475749734)) ;
#55460=CARTESIAN_POINT('Ctrl Pts',(13.6255006617006,-16.0773468007021,24.9381781354869)) ;
#55461=CARTESIAN_POINT('Ctrl Pts',(13.6916098841753,-16.0691106491231,24.9521759517005)) ;
#55462=CARTESIAN_POINT('Ctrl Pts',(13.7564943272627,-16.0606518030569,24.9680627177085)) ;
#55463=CARTESIAN_POINT('Ctrl Pts',(13.8096305420636,-16.0537245483846,24.9810729644013)) ;
#55464=CARTESIAN_POINT('Ctrl Pts',(13.8619456988614,-16.0466480826281,24.9953490704592)) ;
#55465=CARTESIAN_POINT('Ctrl Pts',(13.9133032862433,-16.0394576303854,25.0107714755065)) ;
#55466=CARTESIAN_POINT('Ctrl Pts',(13.9761187441819,-16.0306629892537,25.0296346169612)) ;
#55467=CARTESIAN_POINT('Ctrl Pts',(14.0391122975756,-16.0214720150687,25.0506976401651)) ;
#55468=CARTESIAN_POINT('Ctrl Pts',(14.1019497399007,-16.0119118209662,25.0740004313405)) ;
#55469=CARTESIAN_POINT('Ctrl Pts',(14.1642725257765,-16.002429927561,25.0971123660564)) ;
#55470=CARTESIAN_POINT('Ctrl Pts',(14.2264412559457,-15.9925848997543,25.1224275507145)) ;
#55471=CARTESIAN_POINT('Ctrl Pts',(14.2881325020626,-15.9824119250012,25.1499345996097)) ;
#55472=CARTESIAN_POINT('Ctrl Pts',(14.3387871370542,-15.9740589032139,25.1725206164141)) ;
#55473=CARTESIAN_POINT('Ctrl Pts',(14.3891197709798,-15.9654849570548,25.1965834656511)) ;
#55474=CARTESIAN_POINT('Ctrl Pts',(14.4389562540117,-15.9567135267634,25.222091290738)) ;
#55475=CARTESIAN_POINT('Ctrl Pts',(14.5013901204959,-15.9457249040844,25.2540468391412)) ;
#55476=CARTESIAN_POINT('Ctrl Pts',(14.5630540378178,-15.9344245943125,25.2882760305698)) ;
#55477=CARTESIAN_POINT('Ctrl Pts',(14.623645293248,-15.9228603613731,25.3246844831794)) ;
#55478=CARTESIAN_POINT('Ctrl Pts',(14.6444417835184,-15.9188912167151,25.3371808083518)) ;
#55479=CARTESIAN_POINT('Ctrl Pts',(14.6651120677952,-15.9148910348743,25.3499334400899)) ;
#55480=CARTESIAN_POINT('Ctrl Pts',(14.6856444555743,-15.9108619063809,25.3629372648498)) ;
#55481=CARTESIAN_POINT('',(15.5295807620182,-15.910861895547,24.8551575119669)) ;
#55482=CARTESIAN_POINT('Origin',(-2.92277791062251E-15,-15.9108618782028,
0.)) ;
#55483=CARTESIAN_POINT('',(16.2696930035343,-16.1877442736409,22.5757134159901)) ;
#55484=CARTESIAN_POINT('Ctrl Pts',(15.5295807250489,-15.910861929778,24.855157512034)) ;
#55485=CARTESIAN_POINT('Ctrl Pts',(15.5241280748862,-15.9226009272666,24.7845576220652)) ;
#55486=CARTESIAN_POINT('Ctrl Pts',(15.5211114436977,-15.9340937852961,24.7139225890774)) ;
#55487=CARTESIAN_POINT('Ctrl Pts',(15.5204901013657,-15.9452906657112,24.6435659572226)) ;
#55488=CARTESIAN_POINT('Ctrl Pts',(15.5202768409764,-15.9491337180079,24.6194177833012)) ;
#55489=CARTESIAN_POINT('Ctrl Pts',(15.5203453060798,-15.952941953782,24.5953023676499)) ;
#55490=CARTESIAN_POINT('Ctrl Pts',(15.52069245721,-15.9567135267634,24.571232212331)) ;
#55491=CARTESIAN_POINT('Ctrl Pts',(15.521674406812,-15.9673817754482,24.5031475155512)) ;
#55492=CARTESIAN_POINT('Ctrl Pts',(15.524890000433,-15.9777576912909,24.4354159463767)) ;
#55493=CARTESIAN_POINT('Ctrl Pts',(15.530238652022,-15.987799766173,24.3683400319804)) ;
#55494=CARTESIAN_POINT('Ctrl Pts',(15.5356308816331,-15.9979236586409,24.3007176180363)) ;
#55495=CARTESIAN_POINT('Ctrl Pts',(15.5431908894628,-16.0077081692743,24.233762060699)) ;
#55496=CARTESIAN_POINT('Ctrl Pts',(15.5527655939029,-16.0171189356804,24.1677669696667)) ;
#55497=CARTESIAN_POINT('Ctrl Pts',(15.5606009013244,-16.0248200870136,24.113760934307)) ;
#55498=CARTESIAN_POINT('Ctrl Pts',(15.5697843769972,-16.0322710948774,24.0603978793023)) ;
#55499=CARTESIAN_POINT('Ctrl Pts',(15.5802091422045,-16.0394576303854,24.0078274989672)) ;
#55500=CARTESIAN_POINT('Ctrl Pts',(15.5929642160101,-16.048250614111,23.9435057547523)) ;
#55501=CARTESIAN_POINT('Ctrl Pts',(15.6079059492495,-16.0568730319551,23.8787215938134)) ;
#55502=CARTESIAN_POINT('Ctrl Pts',(15.6251059138724,-16.0652608298868,23.8137986591302)) ;
#55503=CARTESIAN_POINT('Ctrl Pts',(15.6421648888317,-16.0735798722812,23.7494079036065)) ;
#55504=CARTESIAN_POINT('Ctrl Pts',(15.6614452892122,-16.0816680200513,23.6848811201159)) ;
#55505=CARTESIAN_POINT('Ctrl Pts',(15.6829662028032,-16.0894673869315,23.6205380511466)) ;
#55506=CARTESIAN_POINT('Ctrl Pts',(15.7006500499983,-16.0958761674671,23.5676670150303)) ;
#55507=CARTESIAN_POINT('Ctrl Pts',(15.7198457642496,-16.1020900207686,23.5149202234632)) ;
#55508=CARTESIAN_POINT('Ctrl Pts',(15.7405377764617,-16.1080799337539,23.4624736022729)) ;
#55509=CARTESIAN_POINT('Ctrl Pts',(15.7664453917911,-16.1155796568301,23.3968073503301)) ;
#55510=CARTESIAN_POINT('Ctrl Pts',(15.7947036644655,-16.1227292229208,23.3316022881925)) ;
#55511=CARTESIAN_POINT('Ctrl Pts',(15.8252464240103,-16.1294814162038,23.2671686441292)) ;
#55512=CARTESIAN_POINT('Ctrl Pts',(15.8557287949689,-16.1362202591735,23.2028623970899)) ;
#55513=CARTESIAN_POINT('Ctrl Pts',(15.8884864815826,-16.142563213636,23.1393250039253)) ;
#55514=CARTESIAN_POINT('Ctrl Pts',(15.9234047081693,-16.1484717649152,23.0768498989313)) ;
#55515=CARTESIAN_POINT('Ctrl Pts',(15.9497384517319,-16.1529277264408,23.0297340068949)) ;
#55516=CARTESIAN_POINT('Ctrl Pts',(15.9772999670473,-16.1571367885212,22.9832220276334)) ;
#55517=CARTESIAN_POINT('Ctrl Pts',(16.0060225026959,-16.1610860188908,22.9374317075191)) ;
#55518=CARTESIAN_POINT('Ctrl Pts',(16.0457567049241,-16.1665493080681,22.8740862612195)) ;
#55519=CARTESIAN_POINT('Ctrl Pts',(16.0877416814169,-16.171518536629,22.8120803744774)) ;
#55520=CARTESIAN_POINT('Ctrl Pts',(16.1317654177772,-16.1759680067789,22.7517036308018)) ;
#55521=CARTESIAN_POINT('Ctrl Pts',(16.1757891541133,-16.1804174769265,22.6913268871595)) ;
#55522=CARTESIAN_POINT('Ctrl Pts',(16.2218512244188,-16.184347145014,22.6325797572578)) ;
#55523=CARTESIAN_POINT('Ctrl Pts',(16.2696930035848,-16.1877442734701,22.5757134158856)) ;
#55524=CARTESIAN_POINT('',(17.1507288516716,-15.9108618782029,23.7655054324319)) ;
#55525=CARTESIAN_POINT('Ctrl Pts',(17.150728851672,-15.9108618782028,23.7655054324317)) ;
#55526=CARTESIAN_POINT('Ctrl Pts',(16.7044060094453,-16.05109715723,23.1629731851543)) ;
#55527=CARTESIAN_POINT('Ctrl Pts',(16.269693003408,-16.1877442737199,22.5757134161625)) ;
#55528=CARTESIAN_POINT('',(18.3109465873825,-15.9108618782029,22.883530839373)) ;
#55529=CARTESIAN_POINT('Origin',(-2.92277791062251E-15,-15.9108618782028,
0.)) ;
#55530=CARTESIAN_POINT('',(17.4002245554774,-16.1877442736409,21.7163056731371)) ;
#55531=CARTESIAN_POINT('Ctrl Pts',(17.4002245556773,-16.1877442737199,21.7163056730615)) ;
#55532=CARTESIAN_POINT('Ctrl Pts',(17.849780652129,-16.0510971576328,22.2922820153621)) ;
#55533=CARTESIAN_POINT('Ctrl Pts',(18.3109465873822,-15.9108618782028,22.8835308393733)) ;
#55534=CARTESIAN_POINT('',(19.7945838954017,-15.910861895547,21.6129864201279)) ;
#55535=CARTESIAN_POINT('Ctrl Pts',(17.4002245553632,-16.1877442734701,21.7163056731579)) ;
#55536=CARTESIAN_POINT('Ctrl Pts',(17.4678171498596,-16.184347145014,21.6854210850259)) ;
#55537=CARTESIAN_POINT('Ctrl Pts',(17.5367458555749,-16.1804174769265,21.6567544995836)) ;
#55538=CARTESIAN_POINT('Ctrl Pts',(17.6066994634976,-16.1759680067789,21.6304879186788)) ;
#55539=CARTESIAN_POINT('Ctrl Pts',(17.6766530714588,-16.171518536629,21.6042213377595)) ;
#55540=CARTESIAN_POINT('Ctrl Pts',(17.7476310141696,-16.166549308068,21.580355045833)) ;
#55541=CARTESIAN_POINT('Ctrl Pts',(17.8192975435826,-16.1610860188908,21.5590158575752)) ;
#55542=CARTESIAN_POINT('Ctrl Pts',(17.8879658184361,-16.155851292919,21.5385694196573)) ;
#55543=CARTESIAN_POINT('Ctrl Pts',(17.9573104625531,-16.1501596984486,21.5204295090022)) ;
#55544=CARTESIAN_POINT('Ctrl Pts',(18.0270243667303,-16.1440425621066,21.5046663915461)) ;
#55545=CARTESIAN_POINT('Ctrl Pts',(18.0968822985277,-16.1379127878754,21.4888707077845)) ;
#55546=CARTESIAN_POINT('Ctrl Pts',(18.1671105122519,-16.1313557844549,21.4754617320138)) ;
#55547=CARTESIAN_POINT('Ctrl Pts',(18.2373929319436,-16.1244124680045,21.4644590552373)) ;
#55548=CARTESIAN_POINT('Ctrl Pts',(18.2903518955713,-16.1191805644222,21.4561683566278)) ;
#55549=CARTESIAN_POINT('Ctrl Pts',(18.3433414428818,-16.1137295207044,21.4492428625507)) ;
#55550=CARTESIAN_POINT('Ctrl Pts',(18.3962263450592,-16.108079933754,21.44367163736)) ;
#55551=CARTESIAN_POINT('Ctrl Pts',(18.4643718094286,-16.1008000918637,21.4364927694394)) ;
#55552=CARTESIAN_POINT('Ctrl Pts',(18.5323529769938,-16.0931892946345,21.4315634807689)) ;
#55553=CARTESIAN_POINT('Ctrl Pts',(18.5998588341161,-16.0853002129681,21.4288216761156)) ;
#55554=CARTESIAN_POINT('Ctrl Pts',(18.6679151599034,-16.0773468007023,21.4260575137349)) ;
#55555=CARTESIAN_POINT('Ctrl Pts',(18.7354879022073,-16.0691106491233,21.4255165401268)) ;
#55556=CARTESIAN_POINT('Ctrl Pts',(18.8022705681543,-16.0606518030571,21.4270836450806)) ;
#55557=CARTESIAN_POINT('Ctrl Pts',(18.8569613062411,-16.0537245483847,21.4283670039488)) ;
#55558=CARTESIAN_POINT('Ctrl Pts',(18.9111223045493,-16.0466480826282,21.4310631302938)) ;
#55559=CARTESIAN_POINT('Ctrl Pts',(18.9645945412809,-16.0394576303854,21.4350846049139)) ;
#55560=CARTESIAN_POINT('Ctrl Pts',(19.0299964265421,-16.0306629892537,21.4400032699587)) ;
#55561=CARTESIAN_POINT('Ctrl Pts',(19.0960451530338,-16.0214720150687,21.4470320994815)) ;
#55562=CARTESIAN_POINT('Ctrl Pts',(19.1624229021537,-16.0119118209663,21.4562818917105)) ;
#55563=CARTESIAN_POINT('Ctrl Pts',(19.2282569987086,-16.0024299275612,21.4654559255213)) ;
#55564=CARTESIAN_POINT('Ctrl Pts',(19.2944142749039,-15.9925848997545,21.476814815938)) ;
#55565=CARTESIAN_POINT('Ctrl Pts',(19.3605764163785,-15.9824119250015,21.4904169709809)) ;
#55566=CARTESIAN_POINT('Ctrl Pts',(19.4149021001289,-15.9740589032141,21.501585690081)) ;
#55567=CARTESIAN_POINT('Ctrl Pts',(19.4692307863376,-15.9654849570549,21.5142659348029)) ;
#55568=CARTESIAN_POINT('Ctrl Pts',(19.5233855484792,-15.9567135267635,21.5284640304184)) ;
#55569=CARTESIAN_POINT('Ctrl Pts',(19.591229244208,-15.9457249040779,21.5462510401065)) ;
#55570=CARTESIAN_POINT('Ctrl Pts',(19.6588097578,-15.934424594299,21.5664240526226)) ;
#55571=CARTESIAN_POINT('Ctrl Pts',(19.7258111644737,-15.9228603613524,21.5889559670063)) ;
#55572=CARTESIAN_POINT('Ctrl Pts',(19.7488077403279,-15.9188912243841,21.5966894893902)) ;
#55573=CARTESIAN_POINT('Ctrl Pts',(19.7717361594137,-15.9148910503533,21.6047004555176)) ;
#55574=CARTESIAN_POINT('Ctrl Pts',(19.7945839053567,-15.910861929778,21.612986384524)) ;
#55575=CARTESIAN_POINT('',(20.5096319469963,-15.910861895147,20.935656936733)) ;
#55576=CARTESIAN_POINT('Origin',(-2.92277791062251E-15,-15.9108618782028,
0.)) ;
#55577=CARTESIAN_POINT('',(20.742427673457,-16.1877442736409,18.5504027148089)) ;
#55578=CARTESIAN_POINT('Ctrl Pts',(20.5096319116864,-15.9108619285365,20.935656944076)) ;
#55579=CARTESIAN_POINT('Ctrl Pts',(20.4891298518627,-15.922600926042,20.8678797989487)) ;
#55580=CARTESIAN_POINT('Ctrl Pts',(20.470999303531,-15.9340937840905,20.7995446603445)) ;
#55581=CARTESIAN_POINT('Ctrl Pts',(20.4552678915474,-15.9452906645261,20.7309664976985)) ;
#55582=CARTESIAN_POINT('Ctrl Pts',(20.4498684728762,-15.949133717225,20.7074287369299)) ;
#55583=CARTESIAN_POINT('Ctrl Pts',(20.4447512352301,-15.9529419533943,20.683862405901)) ;
#55584=CARTESIAN_POINT('Ctrl Pts',(20.4399158977778,-15.9567135267634,20.660280367782)) ;
#55585=CARTESIAN_POINT('Ctrl Pts',(20.4262386927054,-15.9673817754482,20.5935763632393)) ;
#55586=CARTESIAN_POINT('Ctrl Pts',(20.4148188222928,-15.9777576912909,20.5267370629366)) ;
#55587=CARTESIAN_POINT('Ctrl Pts',(20.4056230865347,-15.987799766173,20.4600795441574)) ;
#55588=CARTESIAN_POINT('Ctrl Pts',(20.3963524287203,-15.9979236586409,20.3928789346997)) ;
#55589=CARTESIAN_POINT('Ctrl Pts',(20.3893422221328,-16.0077081692743,20.3258635828738)) ;
#55590=CARTESIAN_POINT('Ctrl Pts',(20.3845060815328,-16.0171189356804,20.2593531419674)) ;
#55591=CARTESIAN_POINT('Ctrl Pts',(20.3805485026257,-16.0248200870136,20.2049253782172)) ;
#55592=CARTESIAN_POINT('Ctrl Pts',(20.3780457943152,-16.0322710948774,20.1508357459762)) ;
#55593=CARTESIAN_POINT('Ctrl Pts',(20.3769257565024,-16.0394576303854,20.0972534155538)) ;
#55594=CARTESIAN_POINT('Ctrl Pts',(20.3755553501015,-16.0482506141109,20.0316935141443)) ;
#55595=CARTESIAN_POINT('Ctrl Pts',(20.3762210743253,-16.0568730319549,19.9652119399159)) ;
#55596=CARTESIAN_POINT('Ctrl Pts',(20.3790624014848,-16.0652608298864,19.8981093834015)) ;
#55597=CARTESIAN_POINT('Ctrl Pts',(20.3818804380289,-16.0735798722808,19.8315568726035)) ;
#55598=CARTESIAN_POINT('Ctrl Pts',(20.3868387223103,-16.0816680200508,19.7643939732964)) ;
#55599=CARTESIAN_POINT('Ctrl Pts',(20.3940246310398,-16.0894673869309,19.6969288492561)) ;
#55600=CARTESIAN_POINT('Ctrl Pts',(20.3999293298064,-16.0958761674667,19.6414924041653)) ;
#55601=CARTESIAN_POINT('Ctrl Pts',(20.407337257923,-16.1020900207684,19.5858522921285)) ;
#55602=CARTESIAN_POINT('Ctrl Pts',(20.4162710291438,-16.108079933754,19.5301836728207)) ;
#55603=CARTESIAN_POINT('Ctrl Pts',(20.4274566357367,-16.1155796568302,19.4604832898847)) ;
#55604=CARTESIAN_POINT('Ctrl Pts',(20.4410370847878,-16.1227292229209,19.3907279925483)) ;
#55605=CARTESIAN_POINT('Ctrl Pts',(20.4570144427586,-16.1294814162038,19.3212349808121)) ;
#55606=CARTESIAN_POINT('Ctrl Pts',(20.4729602105892,-16.1362202591735,19.2518793693892)) ;
#55607=CARTESIAN_POINT('Ctrl Pts',(20.4912933793152,-16.142563213636,19.1827855108568)) ;
#55608=CARTESIAN_POINT('Ctrl Pts',(20.511964936346,-16.1484717649152,19.1142646525586)) ;
#55609=CARTESIAN_POINT('Ctrl Pts',(20.527554487566,-16.1529277264408,19.0625893274493)) ;
#55610=CARTESIAN_POINT('Ctrl Pts',(20.5444729293125,-16.1571367885212,19.0112398613358)) ;
#55611=CARTESIAN_POINT('Ctrl Pts',(20.5626803827667,-16.1610860188908,18.9603455973274)) ;
#55612=CARTESIAN_POINT('Ctrl Pts',(20.587868222951,-16.166549308068,18.8899394534163)) ;
#55613=CARTESIAN_POINT('Ctrl Pts',(20.6155421812562,-16.171518536629,18.8203577009702)) ;
#55614=CARTESIAN_POINT('Ctrl Pts',(20.6455574519583,-16.1759680067789,18.7519287300249)) ;
#55615=CARTESIAN_POINT('Ctrl Pts',(20.6755727226438,-16.1804174769264,18.6834997591173)) ;
#55616=CARTESIAN_POINT('Ctrl Pts',(20.7079289909665,-16.184347145014,18.6162241209359)) ;
#55617=CARTESIAN_POINT('Ctrl Pts',(20.7424276734838,-16.1877442734701,18.550402714696)) ;
#55618=CARTESIAN_POINT('',(21.8586355065996,-15.9108618782029,19.5229813909693)) ;
#55619=CARTESIAN_POINT('Ctrl Pts',(21.858635506599,-15.9108618782028,19.5229813909701)) ;
#55620=CARTESIAN_POINT('Ctrl Pts',(21.293220824393,-16.0510971566263,19.0304822327909)) ;
#55621=CARTESIAN_POINT('Ctrl Pts',(20.7424276733708,-16.1877442737198,18.5504027150044)) ;
#55622=CARTESIAN_POINT('',(22.80212952987,-15.9108618782029,18.412214356387)) ;
#55623=CARTESIAN_POINT('Origin',(-2.92277791062251E-15,-15.9108618782028,
0.)) ;
#55624=CARTESIAN_POINT('',(21.6617807651629,-16.1877442736409,17.4680565820071)) ;
#55625=CARTESIAN_POINT('Ctrl Pts',(21.6617807653418,-16.1877442737198,17.4680565818904)) ;
#55626=CARTESIAN_POINT('Ctrl Pts',(22.2246443813642,-16.0510971568007,17.9339256482671)) ;
#55627=CARTESIAN_POINT('Ctrl Pts',(22.8021295298706,-15.9108618782028,18.4122143563863)) ;
#55628=CARTESIAN_POINT('',(23.977950736946,-15.910861895147,16.8524363944926)) ;
#55629=CARTESIAN_POINT('Ctrl Pts',(21.6617807650558,-16.1877442734701,17.4680565820518)) ;
#55630=CARTESIAN_POINT('Ctrl Pts',(21.7211538087481,-16.184347145014,17.4233636486337)) ;
#55631=CARTESIAN_POINT('Ctrl Pts',(21.7823085311363,-16.1804174769264,17.380549637818)) ;
#55632=CARTESIAN_POINT('Ctrl Pts',(21.8449801241196,-16.1759680067789,17.3398591970888)) ;
#55633=CARTESIAN_POINT('Ctrl Pts',(21.9076517171373,-16.171518536629,17.2991687563371)) ;
#55634=CARTESIAN_POINT('Ctrl Pts',(21.9718396877089,-16.166549308068,17.2606022854635)) ;
#55635=CARTESIAN_POINT('Ctrl Pts',(22.0372433987964,-16.1610860188908,17.2243558101925)) ;
#55636=CARTESIAN_POINT('Ctrl Pts',(22.0999108677834,-16.155851292919,17.189625749357)) ;
#55637=CARTESIAN_POINT('Ctrl Pts',(22.1637347280774,-16.1501596984486,17.1570028910605)) ;
#55638=CARTESIAN_POINT('Ctrl Pts',(22.228430155617,-16.1440425621066,17.126621877861)) ;
#55639=CARTESIAN_POINT('Ctrl Pts',(22.293259242698,-16.1379127878754,17.0961780980572)) ;
#55640=CARTESIAN_POINT('Ctrl Pts',(22.3589630263876,-16.1313557844549,17.067985626669)) ;
#55641=CARTESIAN_POINT('Ctrl Pts',(22.4252370318935,-16.1244124680045,17.042131543661)) ;
#55642=CARTESIAN_POINT('Ctrl Pts',(22.4751755892518,-16.1191805644222,17.0226500652536)) ;
#55643=CARTESIAN_POINT('Ctrl Pts',(22.5254374938827,-16.1137295207044,17.0044952990674)) ;
#55644=CARTESIAN_POINT('Ctrl Pts',(22.5758883277042,-16.108079933754,16.9876856353241)) ;
#55645=CARTESIAN_POINT('Ctrl Pts',(22.6408973445889,-16.1008000918637,16.9660253448722)) ;
#55646=CARTESIAN_POINT('Ctrl Pts',(22.7062294988791,-16.0931892946344,16.9465973587139)) ;
#55647=CARTESIAN_POINT('Ctrl Pts',(22.7715676996226,-16.085300212968,16.9294078921073)) ;
#55648=CARTESIAN_POINT('Ctrl Pts',(22.8374386931289,-16.0773468007022,16.9120782559934)) ;
#55649=CARTESIAN_POINT('Ctrl Pts',(22.9033153289341,-16.069110649123,16.8970237878882)) ;
#55650=CARTESIAN_POINT('Ctrl Pts',(22.968873534505,-16.0606518030569,16.8841979557019)) ;
#55651=CARTESIAN_POINT('Ctrl Pts',(23.0225615177478,-16.0537245483846,16.8736944183111)) ;
#55652=CARTESIAN_POINT('Ctrl Pts',(23.0760358494802,-16.0466480826281,16.8646844970719)) ;
#55653=CARTESIAN_POINT('Ctrl Pts',(23.1291224332011,-16.0394576303853,16.857117001581)) ;
#55654=CARTESIAN_POINT('Ctrl Pts',(23.1940526263188,-16.0306629892538,16.8478611989052)) ;
#55655=CARTESIAN_POINT('Ctrl Pts',(23.2600681608652,-16.0214720150689,16.8405271744905)) ;
#55656=CARTESIAN_POINT('Ctrl Pts',(23.3268824670043,-16.0119118209665,16.8352914577688)) ;
#55657=CARTESIAN_POINT('Ctrl Pts',(23.3931495450529,-16.0024299275614,16.83009862305)) ;
#55658=CARTESIAN_POINT('Ctrl Pts',(23.4602019265677,-15.9925848997549,16.8269700901341)) ;
#55659=CARTESIAN_POINT('Ctrl Pts',(23.5277412951986,-15.9824119250019,16.8260313296728)) ;
#55660=CARTESIAN_POINT('Ctrl Pts',(23.5831978191147,-15.9740589032144,16.8252605141762)) ;
#55661=CARTESIAN_POINT('Ctrl Pts',(23.6389822086216,-15.9654849570551,16.8259652402328)) ;
#55662=CARTESIAN_POINT('Ctrl Pts',(23.6949230333843,-15.9567135267635,16.8281897192057)) ;
#55663=CARTESIAN_POINT('Ctrl Pts',(23.7650042625084,-15.9457249040783,16.8309764893552)) ;
#55664=CARTESIAN_POINT('Ctrl Pts',(23.835341382626,-15.9344245942998,16.8361500552922)) ;
#55665=CARTESIAN_POINT('Ctrl Pts',(23.9056200291962,-15.9228603613537,16.8437518641509)) ;
#55666=CARTESIAN_POINT('Ctrl Pts',(23.9297414390779,-15.9188912239773,16.8463609973126)) ;
#55667=CARTESIAN_POINT('Ctrl Pts',(23.9538559278607,-15.914891049532,16.8492557394864)) ;
#55668=CARTESIAN_POINT('Ctrl Pts',(23.9779507384798,-15.9108619285365,16.8524363584598)) ;
#55669=CARTESIAN_POINT('',(24.5306755365459,-15.9108618883339,16.0372283765163)) ;
#55670=CARTESIAN_POINT('Origin',(-2.92277791062251E-15,-15.9108618782028,
0.)) ;
#55671=CARTESIAN_POINT('',(24.2452694789222,-16.1877442736409,13.6576957999734)) ;
#55672=CARTESIAN_POINT('Ctrl Pts',(24.5306755198089,-15.9108619232992,16.0372283458231)) ;
#55673=CARTESIAN_POINT('Ctrl Pts',(24.4960827033786,-15.9226009208764,15.9754431298308)) ;
#55674=CARTESIAN_POINT('Ctrl Pts',(24.4636860016978,-15.9340937790044,15.912603161026)) ;
#55675=CARTESIAN_POINT('Ctrl Pts',(24.4335801028943,-15.9452906595266,15.8490101065037)) ;
#55676=CARTESIAN_POINT('Ctrl Pts',(24.4232469921228,-15.9491337139222,15.8271833515223)) ;
#55677=CARTESIAN_POINT('Ctrl Pts',(24.4131833236117,-15.9529419517588,15.8052680335759)) ;
#55678=CARTESIAN_POINT('Ctrl Pts',(24.4033915883005,-15.9567135267634,15.7832767754878)) ;
#55679=CARTESIAN_POINT('Ctrl Pts',(24.3756947594617,-15.9673817754482,15.7210724682984)) ;
#55680=CARTESIAN_POINT('Ctrl Pts',(24.3501734054637,-15.9777576912909,15.6582507682632)) ;
#55681=CARTESIAN_POINT('Ctrl Pts',(24.3268632647421,-15.9877997661731,15.5951284765947)) ;
#55682=CARTESIAN_POINT('Ctrl Pts',(24.303363205158,-15.997923658641,15.5314918974333)) ;
#55683=CARTESIAN_POINT('Ctrl Pts',(24.2821105736219,-16.0077081692744,15.467550314488)) ;
#55684=CARTESIAN_POINT('Ctrl Pts',(24.2630897205414,-16.0171189356805,15.4036344780031)) ;
#55685=CARTESIAN_POINT('Ctrl Pts',(24.2475243072968,-16.0248200870136,15.3513299676034)) ;
#55686=CARTESIAN_POINT('Ctrl Pts',(24.2334524388622,-16.0322710948774,15.2990429292134)) ;
#55687=CARTESIAN_POINT('Ctrl Pts',(24.2208399697526,-16.0394576303854,15.2469540989219)) ;
#55688=CARTESIAN_POINT('Ctrl Pts',(24.2054081618257,-16.0482506141109,15.1832215484423)) ;
#55689=CARTESIAN_POINT('Ctrl Pts',(24.1917667485092,-16.0568730319549,15.1181511654454)) ;
#55690=CARTESIAN_POINT('Ctrl Pts',(24.1801165809055,-16.0652608298864,15.0520066280625)) ;
#55691=CARTESIAN_POINT('Ctrl Pts',(24.1685619107778,-16.0735798722808,14.9864042834267)) ;
#55692=CARTESIAN_POINT('Ctrl Pts',(24.1589662350982,-16.0816680200508,14.9197457308275)) ;
#55693=CARTESIAN_POINT('Ctrl Pts',(24.151481133861,-16.0894673869309,14.8523131459332)) ;
#55694=CARTESIAN_POINT('Ctrl Pts',(24.1453305870469,-16.0958761674667,14.796903438429)) ;
#55695=CARTESIAN_POINT('Ctrl Pts',(24.1406043425428,-16.1020900207685,14.7409716757236)) ;
#55696=CARTESIAN_POINT('Ctrl Pts',(24.1373621395585,-16.108079933754,14.6846840610676)) ;
#55697=CARTESIAN_POINT('Ctrl Pts',(24.1333027108827,-16.1155796568301,14.6142086595785)) ;
#55698=CARTESIAN_POINT('Ctrl Pts',(24.1315703296063,-16.1227292229208,14.5431648072197)) ;
#55699=CARTESIAN_POINT('Ctrl Pts',(24.132235202502,-16.1294814162037,14.4718618438038)) ;
#55700=CARTESIAN_POINT('Ctrl Pts',(24.1328987608232,-16.1362202591734,14.4006998593048)) ;
#55701=CARTESIAN_POINT('Ctrl Pts',(24.1359501730677,-16.1425632136358,14.3292802874376)) ;
#55702=CARTESIAN_POINT('Ctrl Pts',(24.1414084815104,-16.148471764915,14.2579176350146)) ;
#55703=CARTESIAN_POINT('Ctrl Pts',(24.1455248902993,-16.1529277264407,14.2040991576006)) ;
#55704=CARTESIAN_POINT('Ctrl Pts',(24.1510091709447,-16.1571367885211,14.1503132485985)) ;
#55705=CARTESIAN_POINT('Ctrl Pts',(24.1578501819171,-16.1610860188908,14.0966947999152)) ;
#55706=CARTESIAN_POINT('Ctrl Pts',(24.167313904645,-16.1665493080681,14.0225200714308)) ;
#55707=CARTESIAN_POINT('Ctrl Pts',(24.1793828412297,-16.171518536629,13.9486160186902)) ;
#55708=CARTESIAN_POINT('Ctrl Pts',(24.1939861655753,-16.1759680067789,13.8753344831029)) ;
#55709=CARTESIAN_POINT('Ctrl Pts',(24.2085894899129,-16.1804174769265,13.8020529475559)) ;
#55710=CARTESIAN_POINT('Ctrl Pts',(24.2257270131076,-16.184347145014,13.7293945351644)) ;
#55711=CARTESIAN_POINT('Ctrl Pts',(24.2452694789242,-16.1877442734701,13.6576957998574)) ;
#55712=CARTESIAN_POINT('',(25.5444566593685,-15.9108618782029,14.367584437899)) ;
#55713=CARTESIAN_POINT('Ctrl Pts',(25.5444566593687,-15.9108618782028,14.3675844378987)) ;
#55714=CARTESIAN_POINT('Ctrl Pts',(24.8863882921944,-16.0510971577332,14.0081470766494)) ;
#55715=CARTESIAN_POINT('Ctrl Pts',(24.2452694788798,-16.1877442737199,13.6576958001829)) ;
#55716=CARTESIAN_POINT('',(26.2271102382866,-15.9108618782029,13.0799631938043)) ;
#55717=CARTESIAN_POINT('Origin',(-2.92277791062251E-15,-15.9108618782028,
0.)) ;
#55718=CARTESIAN_POINT('',(24.9104561816079,-16.1877442736409,12.403020579454)) ;
#55719=CARTESIAN_POINT('Ctrl Pts',(24.9104561817576,-16.1877442737199,12.4030205793014)) ;
#55720=CARTESIAN_POINT('Ctrl Pts',(25.5603084332828,-16.0510971576887,12.7369988443091)) ;
#55721=CARTESIAN_POINT('Ctrl Pts',(26.2271102382865,-15.9108618782028,13.0799631938046)) ;
#55722=CARTESIAN_POINT('',(27.040135303883,-15.9108618883339,11.303885129792)) ;
#55723=CARTESIAN_POINT('Ctrl Pts',(24.9104561815129,-16.1877442734702,12.4030205795208)) ;
#55724=CARTESIAN_POINT('Ctrl Pts',(24.9588334568668,-16.184347145014,12.3466090927103)) ;
#55725=CARTESIAN_POINT('Ctrl Pts',(25.0093546690776,-16.1804174769265,12.2916495920824)) ;
#55726=CARTESIAN_POINT('Ctrl Pts',(25.0618137930884,-16.1759680067789,12.2384379313129)) ;
#55727=CARTESIAN_POINT('Ctrl Pts',(25.114272917128,-16.171518536629,12.185226270514)) ;
#55728=CARTESIAN_POINT('Ctrl Pts',(25.1686695573966,-16.166549308068,12.1337629460074)) ;
#55729=CARTESIAN_POINT('Ctrl Pts',(25.2247522453194,-16.1610860188908,12.0843040286217)) ;
#55730=CARTESIAN_POINT('Ctrl Pts',(25.2784886472403,-16.155851292919,12.0369142839135)) ;
#55731=CARTESIAN_POINT('Ctrl Pts',(25.3338073909395,-16.1501596984485,11.9913338865715)) ;
#55732=CARTESIAN_POINT('Ctrl Pts',(25.3904592555537,-16.1440425621065,11.9477555600397)) ;
#55733=CARTESIAN_POINT('Ctrl Pts',(25.447228161859,-16.1379127878753,11.9040872015014)) ;
#55734=CARTESIAN_POINT('Ctrl Pts',(25.5053352796135,-16.1313557844548,11.862429483124)) ;
#55735=CARTESIAN_POINT('Ctrl Pts',(25.5645019720945,-16.1244124680043,11.8229329020711)) ;
#55736=CARTESIAN_POINT('Ctrl Pts',(25.6090850517435,-16.1191805644221,11.7931715761443)) ;
#55737=CARTESIAN_POINT('Ctrl Pts',(25.6542691228957,-16.1137295207043,11.7646364345387)) ;
#55738=CARTESIAN_POINT('Ctrl Pts',(25.6999268634434,-16.1080799337539,11.737374333437)) ;
#55739=CARTESIAN_POINT('Ctrl Pts',(25.7587596834656,-16.1008000918637,11.7022454315618)) ;
#55740=CARTESIAN_POINT('Ctrl Pts',(25.8183879655569,-16.0931892946345,11.6692271789562)) ;
#55741=CARTESIAN_POINT('Ctrl Pts',(25.8785033682724,-16.0853002129681,11.6383938107501)) ;
#55742=CARTESIAN_POINT('Ctrl Pts',(25.9391089750513,-16.0773468007024,11.6073090154273)) ;
#55743=CARTESIAN_POINT('Ctrl Pts',(26.0002091860835,-16.0691106491234,11.578444983022)) ;
#55744=CARTESIAN_POINT('Ctrl Pts',(26.0614775024479,-16.0606518030573,11.5518259353539)) ;
#55745=CARTESIAN_POINT('Ctrl Pts',(26.1116523404216,-16.0537245483848,11.5300266354382)) ;
#55746=CARTESIAN_POINT('Ctrl Pts',(26.1619396052601,-16.0466480826282,11.5097319605179)) ;
#55747=CARTESIAN_POINT('Ctrl Pts',(26.2121582663181,-16.0394576303853,11.490929342594)) ;
#55748=CARTESIAN_POINT('Ctrl Pts',(26.273580703628,-16.0306629892537,11.4679318632436)) ;
#55749=CARTESIAN_POINT('Ctrl Pts',(26.3364762332058,-16.0214720150687,11.4465779157217)) ;
#55750=CARTESIAN_POINT('Ctrl Pts',(26.400602933669,-16.0119118209662,11.4271015063442)) ;
#55751=CARTESIAN_POINT('Ctrl Pts',(26.4642044182933,-16.0024299275611,11.4077846142756)) ;
#55752=CARTESIAN_POINT('Ctrl Pts',(26.5290166102924,-15.9925848997544,11.3903149447492)) ;
#55753=CARTESIAN_POINT('Ctrl Pts',(26.5947751402681,-15.9824119250013,11.3748791641796)) ;
#55754=CARTESIAN_POINT('Ctrl Pts',(26.6487694189249,-15.974058903214,11.3622048565625)) ;
#55755=CARTESIAN_POINT('Ctrl Pts',(26.7034010956744,-15.9654849570548,11.3509011117465)) ;
#55756=CARTESIAN_POINT('Ctrl Pts',(26.7585122522638,-15.9567135267634,11.3410479599125)) ;
#55757=CARTESIAN_POINT('Ctrl Pts',(26.827554094393,-15.9457249040797,11.3287041842507)) ;
#55758=CARTESIAN_POINT('Ctrl Pts',(26.8973589354675,-15.9344245943026,11.3186363934173)) ;
#55759=CARTESIAN_POINT('Ctrl Pts',(26.9676286705233,-15.922860361358,11.310952644619)) ;
#55760=CARTESIAN_POINT('Ctrl Pts',(26.9917470322096,-15.9188912222604,11.3083153864527)) ;
#55761=CARTESIAN_POINT('Ctrl Pts',(27.0159200321511,-15.914891046067,11.3059585479934)) ;
#55762=CARTESIAN_POINT('Ctrl Pts',(27.040135269086,-15.9108619232992,11.3038851331635)) ;
#55763=CARTESIAN_POINT('',(27.4046920069319,-15.9108618948274,10.3889167040556)) ;
#55764=CARTESIAN_POINT('Origin',(-2.92277791062251E-15,-15.9108618782028,
0.)) ;
#55765=CARTESIAN_POINT('',(26.6144294302344,-16.1877442736409,8.1263702089704)) ;
#55766=CARTESIAN_POINT('Ctrl Pts',(27.4046919783062,-15.9108619275541,10.3889167248043)) ;
#55767=CARTESIAN_POINT('Ctrl Pts',(27.3576259280778,-15.9226009250732,10.3360124454355)) ;
#55768=CARTESIAN_POINT('Ctrl Pts',(27.3124779080023,-15.9340937831366,10.2816059730657)) ;
#55769=CARTESIAN_POINT('Ctrl Pts',(27.2694052419543,-15.9452906635885,10.2259715668355)) ;
#55770=CARTESIAN_POINT('Ctrl Pts',(27.254621611824,-15.9491337166056,10.2068764292532)) ;
#55771=CARTESIAN_POINT('Ctrl Pts',(27.2400820859543,-15.9529419530876,10.1876368772434)) ;
#55772=CARTESIAN_POINT('Ctrl Pts',(27.2257918105759,-15.9567135267635,10.168264703024)) ;
#55773=CARTESIAN_POINT('Ctrl Pts',(27.1853704309042,-15.9673817754483,10.1134686974568)) ;
#55774=CARTESIAN_POINT('Ctrl Pts',(27.1469409434687,-15.977757691291,10.0576020705611)) ;
#55775=CARTESIAN_POINT('Ctrl Pts',(27.1106063540562,-15.9877997661732,10.0009665342062)) ;
#55776=CARTESIAN_POINT('Ctrl Pts',(27.07397572937,-15.9979236586412,9.94386956105565)) ;
#55777=CARTESIAN_POINT('Ctrl Pts',(27.0394744223152,-16.0077081692747,9.88599158434337)) ;
#55778=CARTESIAN_POINT('Ctrl Pts',(27.0071582507039,-16.0171189356808,9.82765898575631)) ;
#55779=CARTESIAN_POINT('Ctrl Pts',(26.9807128245458,-16.0248200870138,9.77992342948141)) ;
#55780=CARTESIAN_POINT('Ctrl Pts',(26.9557297809157,-16.0322710948775,9.73188386874515)) ;
#55781=CARTESIAN_POINT('Ctrl Pts',(26.9322146255475,-16.0394576303853,9.6837241543968)) ;
#55782=CARTESIAN_POINT('Ctrl Pts',(26.9034429902816,-16.0482506141109,9.62479901807348)) ;
#55783=CARTESIAN_POINT('Ctrl Pts',(26.8761322967502,-16.056873031955,9.56418244509614)) ;
#55784=CARTESIAN_POINT('Ctrl Pts',(26.850535383272,-16.0652608298866,9.50208877189789)) ;
#55785=CARTESIAN_POINT('Ctrl Pts',(26.8251482900055,-16.073579872281,9.44050408614717)) ;
#55786=CARTESIAN_POINT('Ctrl Pts',(26.8014473374946,-16.0816680200511,9.3774667600895)) ;
#55787=CARTESIAN_POINT('Ctrl Pts',(26.7796412213054,-16.0894673869313,9.31321978706453)) ;
#55788=CARTESIAN_POINT('Ctrl Pts',(26.761723021644,-16.0958761674669,9.26042771348703)) ;
#55789=CARTESIAN_POINT('Ctrl Pts',(26.7450835984599,-16.1020900207685,9.20681960717438)) ;
#55790=CARTESIAN_POINT('Ctrl Pts',(26.7298170230788,-16.1080799337539,9.1525449434731)) ;
#55791=CARTESIAN_POINT('Ctrl Pts',(26.7107023735074,-16.1155796568301,9.08458987487628)) ;
#55792=CARTESIAN_POINT('Ctrl Pts',(26.6937381661266,-16.1227292229208,9.01557939907129)) ;
#55793=CARTESIAN_POINT('Ctrl Pts',(26.6790594652296,-16.1294814162037,8.94580053129722)) ;
#55794=CARTESIAN_POINT('Ctrl Pts',(26.664409786792,-16.1362202591734,8.87615962902581)) ;
#55795=CARTESIAN_POINT('Ctrl Pts',(26.6520367619099,-16.1425632136359,8.80575384362681)) ;
#55796=CARTESIAN_POINT('Ctrl Pts',(26.6420265973284,-16.1484717649151,8.73488623539158)) ;
#55797=CARTESIAN_POINT('Ctrl Pts',(26.6344773849863,-16.1529277264407,8.68144109786278)) ;
#55798=CARTESIAN_POINT('Ctrl Pts',(26.6282710656625,-16.1571367885211,8.62773371529949)) ;
#55799=CARTESIAN_POINT('Ctrl Pts',(26.6234257560832,-16.1610860188908,8.57389822101004)) ;
#55800=CARTESIAN_POINT('Ctrl Pts',(26.6167228481979,-16.166549308068,8.49942323581703)) ;
#55801=CARTESIAN_POINT('Ctrl Pts',(26.6126224330011,-16.171518536629,8.42465255414971)) ;
#55802=CARTESIAN_POINT('Ctrl Pts',(26.6111309757742,-16.1759680067789,8.34994501707801)) ;
#55803=CARTESIAN_POINT('Ctrl Pts',(26.6096395185481,-16.1804174769265,8.2752374800475)) ;
#55804=CARTESIAN_POINT('Ctrl Pts',(26.6107569650772,-16.184347145014,8.2005937200553)) ;
#55805=CARTESIAN_POINT('Ctrl Pts',(26.6144294302114,-16.1877442734701,8.12637020885662)) ;
#55806=CARTESIAN_POINT('',(28.0358474093688,-15.9108618782029,8.54037520493671)) ;
#55807=CARTESIAN_POINT('Ctrl Pts',(28.0358474093689,-15.9108618782028,8.54037520493676)) ;
#55808=CARTESIAN_POINT('Ctrl Pts',(27.3158959072615,-16.0510971577111,8.33080653606366)) ;
#55809=CARTESIAN_POINT('Ctrl Pts',(26.614429430238,-16.1877442737199,8.12637020918415)) ;
#55810=CARTESIAN_POINT('',(28.4257404213013,-15.9108618782029,7.1361074896129)) ;
#55811=CARTESIAN_POINT('Origin',(-2.92277791062251E-15,-15.9108618782028,
0.)) ;
#55812=CARTESIAN_POINT('',(26.9943463529853,-16.1877442736409,6.75803311957223)) ;
#55813=CARTESIAN_POINT('Ctrl Pts',(26.9943463530987,-16.1877442737199,6.75803311939104)) ;
#55814=CARTESIAN_POINT('Ctrl Pts',(27.7008008740359,-16.0510971578292,6.9445041333834)) ;
#55815=CARTESIAN_POINT('Ctrl Pts',(28.4257404213014,-15.9108618782028,7.13610748961287)) ;
#55816=CARTESIAN_POINT('',(28.8379530854688,-15.9108618948274,5.22677683844473)) ;
#55817=CARTESIAN_POINT('Ctrl Pts',(26.994346352907,-16.1877442734701,6.75803311965786)) ;
#55818=CARTESIAN_POINT('Ctrl Pts',(27.0294657922942,-16.184347145014,6.69254081788165)) ;
#55819=CARTESIAN_POINT('Ctrl Pts',(27.0669911785949,-16.1804174769264,6.62800567260791)) ;
#55820=CARTESIAN_POINT('Ctrl Pts',(27.1067849032983,-16.1759680067789,6.56476090991527)) ;
#55821=CARTESIAN_POINT('Ctrl Pts',(27.1465786280237,-16.171518536629,6.50151614718779)) ;
#55822=CARTESIAN_POINT('Ctrl Pts',(27.1886404115476,-16.166549308068,6.43956233690494)) ;
#55823=CARTESIAN_POINT('Ctrl Pts',(27.2327797121498,-16.1610860188908,6.37920362141187)) ;
#55824=CARTESIAN_POINT('Ctrl Pts',(27.275072392574,-16.155851292919,6.32137008462396)) ;
#55825=CARTESIAN_POINT('Ctrl Pts',(27.3192993767049,-16.1501596984486,6.26496343695771)) ;
#55826=CARTESIAN_POINT('Ctrl Pts',(27.365258700168,-16.1440425621066,6.21022547120853)) ;
#55827=CARTESIAN_POINT('Ctrl Pts',(27.4113129747325,-16.1379127878754,6.15537441784739)) ;
#55828=CARTESIAN_POINT('Ctrl Pts',(27.4591064023066,-16.1313557844549,6.10219932109308)) ;
#55829=CARTESIAN_POINT('Ctrl Pts',(27.508399212981,-16.1244124680045,6.05090705822831)) ;
#55830=CARTESIAN_POINT('Ctrl Pts',(27.5455421596677,-16.1191805644222,6.0122574913044)) ;
#55831=CARTESIAN_POINT('Ctrl Pts',(27.5835356403936,-16.1137295207044,5.97467624578577)) ;
#55832=CARTESIAN_POINT('Ctrl Pts',(27.6222653824652,-16.108079933754,5.93823645287308)) ;
#55833=CARTESIAN_POINT('Ctrl Pts',(27.6721710483487,-16.1008000918638,5.89128152798355)) ;
#55834=CARTESIAN_POINT('Ctrl Pts',(27.7233073060428,-16.0931892946346,5.84621690572527)) ;
#55835=CARTESIAN_POINT('Ctrl Pts',(27.7753889813127,-16.0853002129683,5.80318136994858)) ;
#55836=CARTESIAN_POINT('Ctrl Pts',(27.8278953505494,-16.0773468007026,5.75979490589796)) ;
#55837=CARTESIAN_POINT('Ctrl Pts',(27.881362158849,-16.0691106491237,5.71847095926792)) ;
#55838=CARTESIAN_POINT('Ctrl Pts',(27.9354757476287,-16.0606518030576,5.67930337320214)) ;
#55839=CARTESIAN_POINT('Ctrl Pts',(27.9797913206747,-16.053724548385,5.64722762179708)) ;
#55840=CARTESIAN_POINT('Ctrl Pts',(28.0245401420056,-16.0466480826283,5.61659714963857)) ;
#55841=CARTESIAN_POINT('Ctrl Pts',(28.0695427116236,-16.0394576303853,5.58743859879812)) ;
#55842=CARTESIAN_POINT('Ctrl Pts',(28.1245853482227,-16.0306629892537,5.55177477934753)) ;
#55843=CARTESIAN_POINT('Ctrl Pts',(28.1814199477719,-16.0214720150686,5.51739939557131)) ;
#55844=CARTESIAN_POINT('Ctrl Pts',(28.2398605493166,-16.0119118209661,5.48459298879387)) ;
#55845=CARTESIAN_POINT('Ctrl Pts',(28.297822505783,-16.0024299275609,5.45205527577939)) ;
#55846=CARTESIAN_POINT('Ctrl Pts',(28.3573639622018,-15.9925848997542,5.42106133197323)) ;
#55847=CARTESIAN_POINT('Ctrl Pts',(28.4182668577455,-15.9824119250011,5.39185029123897)) ;
#55848=CARTESIAN_POINT('Ctrl Pts',(28.4682741786843,-15.9740589032138,5.36786512803923)) ;
#55849=CARTESIAN_POINT('Ctrl Pts',(28.5191986261912,-15.9654849570548,5.34508146289537)) ;
#55850=CARTESIAN_POINT('Ctrl Pts',(28.5709031781777,-15.9567135267634,5.32361140268334)) ;
#55851=CARTESIAN_POINT('Ctrl Pts',(28.6356773135241,-15.9457249040785,5.29671426243865)) ;
#55852=CARTESIAN_POINT('Ctrl Pts',(28.7016858787851,-15.9344245943003,5.27187587354305)) ;
#55853=CARTESIAN_POINT('Ctrl Pts',(28.7686609676306,-15.9228603613544,5.24926585064139)) ;
#55854=CARTESIAN_POINT('Ctrl Pts',(28.7916485147756,-15.9188912236552,5.24150551801081)) ;
#55855=CARTESIAN_POINT('Ctrl Pts',(28.8147497046315,-15.914891048882,5.23400730323592)) ;
#55856=CARTESIAN_POINT('Ctrl Pts',(28.8379530716378,-15.9108619275541,5.22677680590791)) ;
#55857=CARTESIAN_POINT('',(28.9972957403971,-15.9108618818335,4.25483109005223)) ;
#55858=CARTESIAN_POINT('Origin',(-2.92277791062251E-15,-15.9108618782028,
0.)) ;
#55859=CARTESIAN_POINT('',(27.7391282412025,-16.1877442736409,2.21506457880764)) ;
#55860=CARTESIAN_POINT('Ctrl Pts',(28.9972957168721,-15.9108618853164,4.25483107607865)) ;
#55861=CARTESIAN_POINT('Ctrl Pts',(28.9399571848693,-15.9226008834119,4.21328148344468)) ;
#55862=CARTESIAN_POINT('Ctrl Pts',(28.8841689131692,-15.9340937421155,4.16985249820661)) ;
#55863=CARTESIAN_POINT('Ctrl Pts',(28.8301435051533,-15.9452906232646,4.12477814745126)) ;
#55864=CARTESIAN_POINT('Ctrl Pts',(28.8116005516433,-15.9491336899665,4.10930743429519)) ;
#55865=CARTESIAN_POINT('Ctrl Pts',(28.793264951962,-15.9529419398963,4.0936432064508)) ;
#55866=CARTESIAN_POINT('Ctrl Pts',(28.775144267083,-15.9567135267634,4.0777958742614)) ;
#55867=CARTESIAN_POINT('Ctrl Pts',(28.7238883953676,-15.9673817754481,4.03297037063621)) ;
#55868=CARTESIAN_POINT('Ctrl Pts',(28.6743476946165,-15.9777576912908,3.98667107826351)) ;
#55869=CARTESIAN_POINT('Ctrl Pts',(28.6266876215316,-15.9877997661729,3.93917051195709)) ;
#55870=CARTESIAN_POINT('Ctrl Pts',(28.5786392390422,-15.9979236586407,3.89128293582399)) ;
#55871=CARTESIAN_POINT('Ctrl Pts',(28.5325024992417,-16.0077081692741,3.84217487520988)) ;
#55872=CARTESIAN_POINT('Ctrl Pts',(28.4884020773677,-16.0171189356801,3.79215308199961)) ;
#55873=CARTESIAN_POINT('Ctrl Pts',(28.4523131970299,-16.0248200870134,3.75121854140485)) ;
#55874=CARTESIAN_POINT('Ctrl Pts',(28.4175871575564,-16.0322710948773,3.70967273478831)) ;
#55875=CARTESIAN_POINT('Ctrl Pts',(28.3842688584582,-16.0394576303854,3.6676940310985)) ;
#55876=CARTESIAN_POINT('Ctrl Pts',(28.3435027255416,-16.0482506141109,3.61633158281616)) ;
#55877=CARTESIAN_POINT('Ctrl Pts',(28.3037997694713,-16.0568730319549,3.56300318344106)) ;
#55878=CARTESIAN_POINT('Ctrl Pts',(28.2654529933442,-16.0652608298864,3.50786380557492)) ;
#55879=CARTESIAN_POINT('Ctrl Pts',(28.2274205492046,-16.0735798722808,3.45317641016946)) ;
#55880=CARTESIAN_POINT('Ctrl Pts',(28.1907225500605,-16.0816680200508,3.39670786595972)) ;
#55881=CARTESIAN_POINT('Ctrl Pts',(28.1556150486768,-16.0894673869309,3.33865062185837)) ;
#55882=CARTESIAN_POINT('Ctrl Pts',(28.126767031269,-16.0958761674667,3.2909446808922)) ;
#55883=CARTESIAN_POINT('Ctrl Pts',(28.0989924703388,-16.1020900207684,3.24216688644051)) ;
#55884=CARTESIAN_POINT('Ctrl Pts',(28.0724153706577,-16.1080799337539,3.19244299664488)) ;
#55885=CARTESIAN_POINT('Ctrl Pts',(28.0391392799602,-16.1155796568301,3.13018576442147)) ;
#55886=CARTESIAN_POINT('Ctrl Pts',(28.0077364739579,-16.1227292229208,3.06643551831957)) ;
#55887=CARTESIAN_POINT('Ctrl Pts',(27.9784005590081,-16.1294814162037,3.00144352849088)) ;
#55888=CARTESIAN_POINT('Ctrl Pts',(27.9491226464934,-16.1362202591733,2.93658003963727)) ;
#55889=CARTESIAN_POINT('Ctrl Pts',(27.9219037333767,-16.1425632136358,2.87048013698147)) ;
#55890=CARTESIAN_POINT('Ctrl Pts',(27.8968931599413,-16.148471764915,2.80342126353177)) ;
#55891=CARTESIAN_POINT('Ctrl Pts',(27.8780313192468,-16.1529277264407,2.75284850111858)) ;
#55892=CARTESIAN_POINT('Ctrl Pts',(27.8604246005476,-16.1571367885212,2.70173094251072)) ;
#55893=CARTESIAN_POINT('Ctrl Pts',(27.8441195317072,-16.1610860188909,2.65019569049381)) ;
#55894=CARTESIAN_POINT('Ctrl Pts',(27.8215634137318,-16.1665493080681,2.57890281612689)) ;
#55895=CARTESIAN_POINT('Ctrl Pts',(27.8014853776107,-16.171518536629,2.50676169950606)) ;
#55896=CARTESIAN_POINT('Ctrl Pts',(27.7839688776935,-16.1759680067789,2.43412140235199)) ;
#55897=CARTESIAN_POINT('Ctrl Pts',(27.766452377786,-16.1804174769265,2.36148110523793)) ;
#55898=CARTESIAN_POINT('Ctrl Pts',(27.7514974970917,-16.184347145014,2.28834225690174)) ;
#55899=CARTESIAN_POINT('Ctrl Pts',(27.7391282411555,-16.1877442734701,2.21506457870152)) ;
#55900=CARTESIAN_POINT('',(29.2163130941136,-15.9108618782029,2.31382751933678)) ;
#55901=CARTESIAN_POINT('Ctrl Pts',(29.2163130941136,-15.9108618782028,2.31382751933756)) ;
#55902=CARTESIAN_POINT('Ctrl Pts',(28.4681425925364,-16.0510971570555,2.26392674105533)) ;
#55903=CARTESIAN_POINT('Ctrl Pts',(27.7391282412521,-16.1877442737199,2.21506457901549)) ;
#55904=CARTESIAN_POINT('',(29.2952145751572,-15.9108618782029,0.858575330421187)) ;
#55905=CARTESIAN_POINT('Origin',(-2.92277791062251E-15,-15.9108618782028,
0.)) ;
#55906=CARTESIAN_POINT('',(27.8160108909581,-16.1877442736409,0.79704754203402)) ;
#55907=CARTESIAN_POINT('Ctrl Pts',(27.8160108910298,-16.1877442737199,0.797047541832666)) ;
#55908=CARTESIAN_POINT('Ctrl Pts',(28.546034658842,-16.0510971568885,0.827292127995152)) ;
#55909=CARTESIAN_POINT('Ctrl Pts',(29.2952145751573,-15.9108618782028,0.85857533042041)) ;
#55910=CARTESIAN_POINT('',(29.2873405113753,-15.9108618818335,-1.09472993550084)) ;
#55911=CARTESIAN_POINT('Ctrl Pts',(27.8160108909,-16.1877442734702,0.797047542134493)) ;
#55912=CARTESIAN_POINT('Ctrl Pts',(27.8362303483673,-16.184347145014,0.725536772633904)) ;
#55913=CARTESIAN_POINT('Ctrl Pts',(27.859005263401,-16.1804174769265,0.654443574381639)) ;
#55914=CARTESIAN_POINT('Ctrl Pts',(27.8842728784575,-16.1759680067789,0.584122964577792)) ;
#55915=CARTESIAN_POINT('Ctrl Pts',(27.909540493528,-16.171518536629,0.513802354735197)) ;
#55916=CARTESIAN_POINT('Ctrl Pts',(27.9373006580581,-16.1665493080681,0.444254949988175)) ;
#55917=CARTESIAN_POINT('Ctrl Pts',(27.9674326667007,-16.1610860188908,0.375818742840304)) ;
#55918=CARTESIAN_POINT('Ctrl Pts',(27.996304066897,-16.155851292919,0.310245645875013)) ;
#55919=CARTESIAN_POINT('Ctrl Pts',(28.0273712868368,-16.1501596984485,0.245650260037327)) ;
#55920=CARTESIAN_POINT('Ctrl Pts',(28.0604890622642,-16.1440425621065,0.182312141511965)) ;
#55921=CARTESIAN_POINT('Ctrl Pts',(28.0936752583953,-16.1379127878753,0.118843167620128)) ;
#55922=CARTESIAN_POINT('Ctrl Pts',(28.1289202282347,-16.1313557844548,0.056637100912983)) ;
#55923=CARTESIAN_POINT('Ctrl Pts',(28.1660342800607,-16.1244124680043,-0.00405247455977011)) ;
#55924=CARTESIAN_POINT('Ctrl Pts',(28.1940003308787,-16.1191805644221,-0.0497830716863816)) ;
#55925=CARTESIAN_POINT('Ctrl Pts',(28.2230266882454,-16.1137295207043,-0.0946531638453065)) ;
#55926=CARTESIAN_POINT('Ctrl Pts',(28.2530174721459,-16.1080799337539,-0.138566764351555)) ;
#55927=CARTESIAN_POINT('Ctrl Pts',(28.2916624504208,-16.1008000918637,-0.195152152154858)) ;
#55928=CARTESIAN_POINT('Ctrl Pts',(28.3319156091424,-16.0931892946345,-0.250155972415166)) ;
#55929=CARTESIAN_POINT('Ctrl Pts',(28.3735282757164,-16.0853002129681,-0.30338138194066)) ;
#55930=CARTESIAN_POINT('Ctrl Pts',(28.4154802679428,-16.0773468007024,-0.357040811881018)) ;
#55931=CARTESIAN_POINT('Ctrl Pts',(28.4588136249783,-16.0691106491234,-0.40889241092005)) ;
#55932=CARTESIAN_POINT('Ctrl Pts',(28.5032421949055,-16.0606518030573,-0.458777102591018)) ;
#55933=CARTESIAN_POINT('Ctrl Pts',(28.5396263560801,-16.0537245483848,-0.499629478998345)) ;
#55934=CARTESIAN_POINT('Ctrl Pts',(28.5767443287514,-16.0466480826283,-0.539163501559296)) ;
#55935=CARTESIAN_POINT('Ctrl Pts',(28.6144265367895,-16.0394576303854,-0.577314563885697)) ;
#55936=CARTESIAN_POINT('Ctrl Pts',(28.6605156401652,-16.0306629892538,-0.623977122875787)) ;
#55937=CARTESIAN_POINT('Ctrl Pts',(28.7086317869771,-16.0214720150689,-0.669766588165793)) ;
#55938=CARTESIAN_POINT('Ctrl Pts',(28.7586536720263,-16.0119118209665,-0.714369001223339)) ;
#55939=CARTESIAN_POINT('Ctrl Pts',(28.8082658636697,-16.0024299275614,-0.758606107885602)) ;
#55940=CARTESIAN_POINT('Ctrl Pts',(28.8597524921807,-15.9925848997548,-0.801675083605944)) ;
#55941=CARTESIAN_POINT('Ctrl Pts',(28.9129520015845,-15.9824119250019,-0.843295508705367)) ;
#55942=CARTESIAN_POINT('Ctrl Pts',(28.9566340780589,-15.9740589032144,-0.877470007915371)) ;
#55943=CARTESIAN_POINT('Ctrl Pts',(29.0014701257582,-15.965484957055,-0.910668254528474)) ;
#55944=CARTESIAN_POINT('Ctrl Pts',(29.0473504257582,-15.9567135267634,-0.942751306966303)) ;
#55945=CARTESIAN_POINT('Ctrl Pts',(29.1048280876747,-15.9457249040904,-0.98294413136516)) ;
#55946=CARTESIAN_POINT('Ctrl Pts',(29.1639538899006,-15.9344245943248,-1.02139170282338)) ;
#55947=CARTESIAN_POINT('Ctrl Pts',(29.2245026517423,-15.922860361392,-1.05787078025111)) ;
#55948=CARTESIAN_POINT('Ctrl Pts',(29.245284593372,-15.9188912098109,-1.07039136753889)) ;
#55949=CARTESIAN_POINT('Ctrl Pts',(29.2662338695707,-15.9148910209385,-1.08268039334433)) ;
#55950=CARTESIAN_POINT('Ctrl Pts',(29.2873404864774,-15.9108618853164,-1.09472992415267)) ;
#55951=CARTESIAN_POINT('',(29.2340179925284,-15.9108618818335,-2.07820592662307)) ;
#55952=CARTESIAN_POINT('Origin',(-2.92277791062251E-15,-15.9108618782028,
0.)) ;
#55953=CARTESIAN_POINT('',(27.5667762454386,-16.1877442736409,-3.7998150091926)) ;
#55954=CARTESIAN_POINT('Ctrl Pts',(29.2340179665494,-15.9108618853164,-2.0782059352128)) ;
#55955=CARTESIAN_POINT('Ctrl Pts',(29.1690880433416,-15.922600883412,-2.10645803199504)) ;
#55956=CARTESIAN_POINT('Ctrl Pts',(29.1052681223567,-15.9340937421157,-2.1368788423665)) ;
#55957=CARTESIAN_POINT('Ctrl Pts',(29.0428161453331,-15.9452906232649,-2.16928551410604)) ;
#55958=CARTESIAN_POINT('Ctrl Pts',(29.0213809697546,-15.9491336899667,-2.18040834370659)) ;
#55959=CARTESIAN_POINT('Ctrl Pts',(29.0001067002499,-15.9529419398964,-2.19176473867345)) ;
#55960=CARTESIAN_POINT('Ctrl Pts',(28.9790029589372,-15.9567135267634,-2.20334615743714)) ;
#55961=CARTESIAN_POINT('Ctrl Pts',(28.9193092627717,-15.9673817754482,-2.23610516839168)) ;
#55962=CARTESIAN_POINT('Ctrl Pts',(28.8609738168107,-15.9777576912909,-2.27067222278905)) ;
#55963=CARTESIAN_POINT('Ctrl Pts',(28.8042167921,-15.987799766173,-2.30681674536044)) ;
#55964=CARTESIAN_POINT('Ctrl Pts',(28.7469973407702,-15.9979236586409,-2.34325575464003)) ;
#55965=CARTESIAN_POINT('Ctrl Pts',(28.6913824708994,-16.0077081692743,-2.38129766082209)) ;
#55966=CARTESIAN_POINT('Ctrl Pts',(28.6375598854752,-16.0171189356803,-2.42066968520106)) ;
#55967=CARTESIAN_POINT('Ctrl Pts',(28.5935150268936,-16.0248200870135,-2.45288915649125)) ;
#55968=CARTESIAN_POINT('Ctrl Pts',(28.5506697425885,-16.0322710948774,-2.48599857324384)) ;
#55969=CARTESIAN_POINT('Ctrl Pts',(28.5091062263966,-16.0394576303854,-2.51983338874485)) ;
#55970=CARTESIAN_POINT('Ctrl Pts',(28.4582517748961,-16.0482506141108,-2.56123149798998)) ;
#55971=CARTESIAN_POINT('Ctrl Pts',(28.4080130223862,-16.0568730319548,-2.60477814707854)) ;
#55972=CARTESIAN_POINT('Ctrl Pts',(28.3587094362426,-16.0652608298863,-2.65038497358669)) ;
#55973=CARTESIAN_POINT('Ctrl Pts',(28.3098099960476,-16.0735798722807,-2.695617956819)) ;
#55974=CARTESIAN_POINT('Ctrl Pts',(28.261830907923,-16.0816680200507,-2.74287731281456)) ;
#55975=CARTESIAN_POINT('Ctrl Pts',(28.21506360909,-16.0894673869309,-2.79203013578472)) ;
#55976=CARTESIAN_POINT('Ctrl Pts',(28.1766346751679,-16.0958761674667,-2.83241926736048)) ;
#55977=CARTESIAN_POINT('Ctrl Pts',(28.1390236840916,-16.1020900207684,-2.87408595449453)) ;
#55978=CARTESIAN_POINT('Ctrl Pts',(28.1023787757534,-16.1080799337539,-2.91693403656095)) ;
#55979=CARTESIAN_POINT('Ctrl Pts',(28.0564971969472,-16.1155796568301,-2.97058235342623)) ;
#55980=CARTESIAN_POINT('Ctrl Pts',(28.0121241526303,-16.1227292229208,-3.02609147917076)) ;
#55981=CARTESIAN_POINT('Ctrl Pts',(27.969502738406,-16.1294814162037,-3.0832576378432)) ;
#55982=CARTESIAN_POINT('Ctrl Pts',(27.9269655944633,-16.1362202591734,-3.14031076863114)) ;
#55983=CARTESIAN_POINT('Ctrl Pts',(27.8861735192375,-16.1425632136359,-3.19901403056068)) ;
#55984=CARTESIAN_POINT('Ctrl Pts',(27.8473320035648,-16.1484717649151,-3.2591285708333)) ;
#55985=CARTESIAN_POINT('Ctrl Pts',(27.8180394932255,-16.1529277264407,-3.30446423196756)) ;
#55986=CARTESIAN_POINT('Ctrl Pts',(27.789855645749,-16.1571367885212,-3.35060176639201)) ;
#55987=CARTESIAN_POINT('Ctrl Pts',(27.7628532245448,-16.1610860188908,-3.39742704502891)) ;
#55988=CARTESIAN_POINT('Ctrl Pts',(27.7254985954864,-16.1665493080681,-3.46220423300072)) ;
#55989=CARTESIAN_POINT('Ctrl Pts',(27.690381765095,-16.171518536629,-3.52834254614104)) ;
#55990=CARTESIAN_POINT('Ctrl Pts',(27.6576592745555,-16.175968006779,-3.59551902381645)) ;
#55991=CARTESIAN_POINT('Ctrl Pts',(27.624936784034,-16.1804174769265,-3.66269550145486)) ;
#55992=CARTESIAN_POINT('Ctrl Pts',(27.5946088497164,-16.184347145014,-3.73090954687479)) ;
#55993=CARTESIAN_POINT('Ctrl Pts',(27.56677624537,-16.1877442734702,-3.79981500928618)) ;
#55994=CARTESIAN_POINT('',(29.0306564501773,-15.9108618782029,-4.02091216943267)) ;
#55995=CARTESIAN_POINT('Ctrl Pts',(29.0306564501773,-15.9108618782028,-4.02091216943256)) ;
#55996=CARTESIAN_POINT('Ctrl Pts',(28.2892505645617,-16.0510971574954,-3.90881175282058)) ;
#55997=CARTESIAN_POINT('Ctrl Pts',(27.5667762455317,-16.1877442737199,-3.79981500900026)) ;
#55998=CARTESIAN_POINT('',(28.7948770547713,-15.9108618782029,-5.459102856983)) ;
#55999=CARTESIAN_POINT('Origin',(-2.92277791062251E-15,-15.9108618782028,
0.)) ;
#56000=CARTESIAN_POINT('',(27.3370296749455,-16.187744273641,-5.20120709271523)) ;
#56001=CARTESIAN_POINT('Ctrl Pts',(27.3370296749724,-16.1877442737199,-5.20120709292722)) ;
#56002=CARTESIAN_POINT('Ctrl Pts',(28.0564875803008,-16.0510971577385,-5.32860313832098)) ;
#56003=CARTESIAN_POINT('Ctrl Pts',(28.7948770547713,-15.9108618782028,-5.45910285698312)) ;
#56004=CARTESIAN_POINT('',(28.3672841893431,-15.9108618818335,-7.36504824030179)) ;
#56005=CARTESIAN_POINT('Ctrl Pts',(27.3370296749104,-16.1877442734702,-5.20120709260465)) ;
#56006=CARTESIAN_POINT('Ctrl Pts',(27.3414037110988,-16.184347145014,-5.27539256572612)) ;
#56007=CARTESIAN_POINT('Ctrl Pts',(27.348363225151,-16.1804174769265,-5.34971957802101)) ;
#56008=CARTESIAN_POINT('Ctrl Pts',(27.3579232449636,-16.1759680067789,-5.42382792137733)) ;
#56009=CARTESIAN_POINT('Ctrl Pts',(27.3674832647814,-16.171518536629,-5.49793626477445)) ;
#56010=CARTESIAN_POINT('Ctrl Pts',(27.3796437758774,-16.1665493080681,-5.57182530463607)) ;
#56011=CARTESIAN_POINT('Ctrl Pts',(27.3943595533256,-16.1610860188908,-5.64513900245385)) ;
#56012=CARTESIAN_POINT('Ctrl Pts',(27.4084596787088,-16.155851292919,-5.71538553446148)) ;
#56013=CARTESIAN_POINT('Ctrl Pts',(27.4249144657817,-16.1501596984485,-5.78514925002124)) ;
#56014=CARTESIAN_POINT('Ctrl Pts',(27.443642142802,-16.1440425621065,-5.85412590129558)) ;
#56015=CARTESIAN_POINT('Ctrl Pts',(27.4624085108522,-16.1379127878753,-5.92324505703946)) ;
#56016=CARTESIAN_POINT('Ctrl Pts',(27.4834570073389,-16.1313557844548,-5.99157340715721)) ;
#56017=CARTESIAN_POINT('Ctrl Pts',(27.5066568885023,-16.1244124680043,-6.05882251814029)) ;
#56018=CARTESIAN_POINT('Ctrl Pts',(27.5241383819977,-16.1191805644221,-6.1094958335742)) ;
#56019=CARTESIAN_POINT('Ctrl Pts',(27.5428403757957,-16.1137295207043,-6.15955669673402)) ;
#56020=CARTESIAN_POINT('Ctrl Pts',(27.5626898658027,-16.1080799337539,-6.20889075368092)) ;
#56021=CARTESIAN_POINT('Ctrl Pts',(27.5882671602353,-16.1008000918637,-6.2724607345541)) ;
#56022=CARTESIAN_POINT('Ctrl Pts',(27.6157550270204,-16.0931892946346,-6.33483183531309)) ;
#56023=CARTESIAN_POINT('Ctrl Pts',(27.6449529228583,-16.0853002129682,-6.39575835759351)) ;
#56024=CARTESIAN_POINT('Ctrl Pts',(27.6743889095439,-16.0773468007024,-6.4571816981176)) ;
#56025=CARTESIAN_POINT('Ctrl Pts',(27.7055625957016,-16.0691106491234,-6.51713642642337)) ;
#56026=CARTESIAN_POINT('Ctrl Pts',(27.738228716225,-16.0606518030573,-6.57540567095972)) ;
#56027=CARTESIAN_POINT('Ctrl Pts',(27.7649801825905,-16.0537245483848,-6.62312446065317)) ;
#56028=CARTESIAN_POINT('Ctrl Pts',(27.7927317114543,-16.0466480826283,-6.66971346666096)) ;
#56029=CARTESIAN_POINT('Ctrl Pts',(27.8213315797461,-16.0394576303854,-6.71507313920121)) ;
#56030=CARTESIAN_POINT('Ctrl Pts',(27.8563120746498,-16.0306629892537,-6.77055254833493)) ;
#56031=CARTESIAN_POINT('Ctrl Pts',(27.8934599111776,-16.0214720150688,-6.82561503063382)) ;
#56032=CARTESIAN_POINT('Ctrl Pts',(27.9327241119829,-16.0119118209663,-6.87992789070965)) ;
#56033=CARTESIAN_POINT('Ctrl Pts',(27.9716667278631,-16.0024299275612,-6.9337959130789)) ;
#56034=CARTESIAN_POINT('Ctrl Pts',(28.0126910709413,-15.9925848997546,-6.98692606327699)) ;
#56035=CARTESIAN_POINT('Ctrl Pts',(28.0556996442737,-15.9824119250015,-7.03900974792234)) ;
#56036=CARTESIAN_POINT('Ctrl Pts',(28.0910139509351,-15.9740589032141,-7.08177562154035)) ;
#56037=CARTESIAN_POINT('Ctrl Pts',(28.1276651150658,-15.9654849570549,-7.12383613650684)) ;
#56038=CARTESIAN_POINT('Ctrl Pts',(28.1655758512416,-15.9567135267634,-7.16503201329497)) ;
#56039=CARTESIAN_POINT('Ctrl Pts',(28.2130694482099,-15.9457249040902,-7.21664115008039)) ;
#56040=CARTESIAN_POINT('Ctrl Pts',(28.262547830676,-15.9344245943244,-7.26690013841677)) ;
#56041=CARTESIAN_POINT('Ctrl Pts',(28.3138390727814,-15.9228603613914,-7.31554254927431)) ;
#56042=CARTESIAN_POINT('Ctrl Pts',(28.3314435880026,-15.9188912098104,-7.33223791532878)) ;
#56043=CARTESIAN_POINT('Ctrl Pts',(28.3492613044774,-15.9148910209383,-7.3487431056656)) ;
#56044=CARTESIAN_POINT('Ctrl Pts',(28.3672841674668,-15.9108618853164,-7.36504822386662)) ;
#56045=CARTESIAN_POINT('',(28.1037900289265,-15.9108618823941,-8.31406834816463)) ;
#56046=CARTESIAN_POINT('Origin',(-2.92277791062251E-15,-15.9108618782028,
0.)) ;
#56047=CARTESIAN_POINT('',(26.1054324307097,-16.1877442736409,-9.63701947055319)) ;
#56048=CARTESIAN_POINT('Ctrl Pts',(28.1037899993503,-15.9108618900532,-8.3140683522349)) ;
#56049=CARTESIAN_POINT('Ctrl Pts',(28.034304736139,-15.9226008880843,-8.32770191715421)) ;
#56050=CARTESIAN_POINT('Ctrl Pts',(27.9654373146411,-15.9340937467164,-8.34369210999802)) ;
#56051=CARTESIAN_POINT('Ctrl Pts',(27.8974789538808,-15.9452906277875,-8.36191580337098)) ;
#56052=CARTESIAN_POINT('Ctrl Pts',(27.8741538504537,-15.9491336929544,-8.36817065601886)) ;
#56053=CARTESIAN_POINT('Ctrl Pts',(27.8509356814767,-15.9529419413759,-8.37468820324564)) ;
#56054=CARTESIAN_POINT('Ctrl Pts',(27.82783568028,-15.9567135267634,-8.38146217165719)) ;
#56055=CARTESIAN_POINT('Ctrl Pts',(27.7624953705522,-15.9673817754483,-8.40062291499775)) ;
#56056=CARTESIAN_POINT('Ctrl Pts',(27.698092879999,-15.9777576912911,-8.42184141437466)) ;
#56057=CARTESIAN_POINT('Ctrl Pts',(27.6348927990567,-15.9877997661733,-8.44493981550727)) ;
#56058=CARTESIAN_POINT('Ctrl Pts',(27.5711777968354,-15.9979236586412,-8.46822641035863)) ;
#56059=CARTESIAN_POINT('Ctrl Pts',(27.5086852863975,-16.0077081692746,-8.49342336485628)) ;
#56060=CARTESIAN_POINT('Ctrl Pts',(27.4476572216975,-16.0171189356807,-8.52030462830303)) ;
#56061=CARTESIAN_POINT('Ctrl Pts',(27.3977158735079,-16.0248200870138,-8.54230248362045)) ;
#56062=CARTESIAN_POINT('Ctrl Pts',(27.3487547422468,-16.0322710948775,-8.56542735098012)) ;
#56063=CARTESIAN_POINT('Ctrl Pts',(27.3008894727844,-16.0394576303854,-8.58953619992411)) ;
#56064=CARTESIAN_POINT('Ctrl Pts',(27.2423246003303,-16.048250614111,-8.61903424055521)) ;
#56065=CARTESIAN_POINT('Ctrl Pts',(27.1838991596106,-16.0568730319551,-8.65076294644521)) ;
#56066=CARTESIAN_POINT('Ctrl Pts',(27.1259441443405,-16.0652608298868,-8.68470469707721)) ;
#56067=CARTESIAN_POINT('Ctrl Pts',(27.0684641915654,-16.0735798722812,-8.71836822411347)) ;
#56068=CARTESIAN_POINT('Ctrl Pts',(27.011447463296,-16.0816680200512,-8.75420859693357)) ;
#56069=CARTESIAN_POINT('Ctrl Pts',(26.9552071539288,-16.0894673869314,-8.79215866740018)) ;
#56070=CARTESIAN_POINT('Ctrl Pts',(26.9089941977332,-16.095876167467,-8.82334243868145)) ;
#56071=CARTESIAN_POINT('Ctrl Pts',(26.8633054246535,-16.1020900207686,-8.85594973051555)) ;
#56072=CARTESIAN_POINT('Ctrl Pts',(26.8183061828456,-16.108079933754,-8.88991847615642)) ;
#56073=CARTESIAN_POINT('Ctrl Pts',(26.7619644875617,-16.1155796568302,-8.93244934199296)) ;
#56074=CARTESIAN_POINT('Ctrl Pts',(26.706696039165,-16.1227292229209,-8.97712180235449)) ;
#56075=CARTESIAN_POINT('Ctrl Pts',(26.6527820556249,-16.1294814162038,-9.02378910382704)) ;
#56076=CARTESIAN_POINT('Ctrl Pts',(26.5989746698281,-16.1362202591735,-9.07036413556367)) ;
#56077=CARTESIAN_POINT('Ctrl Pts',(26.5465168245935,-16.142563213636,-9.11892585748311)) ;
#56078=CARTESIAN_POINT('Ctrl Pts',(26.495660552787,-16.1484717649152,-9.169285175488)) ;
#56079=CARTESIAN_POINT('Ctrl Pts',(26.4573070580305,-16.1529277264408,-9.20726389021547)) ;
#56080=CARTESIAN_POINT('Ctrl Pts',(26.4198639271609,-16.1571367885212,-9.24626406062484)) ;
#56081=CARTESIAN_POINT('Ctrl Pts',(26.3834267567978,-16.1610860188908,-9.28618986789499)) ;
#56082=CARTESIAN_POINT('Ctrl Pts',(26.3330202775945,-16.166549308068,-9.34142246015669)) ;
#56083=CARTESIAN_POINT('Ctrl Pts',(26.2845066768924,-16.171518536629,-9.39846541580138)) ;
#56084=CARTESIAN_POINT('Ctrl Pts',(26.2381082630198,-16.1759680067789,-9.45703697656326)) ;
#56085=CARTESIAN_POINT('Ctrl Pts',(26.1917098491729,-16.1804174769265,-9.51560853729283)) ;
#56086=CARTESIAN_POINT('Ctrl Pts',(26.1474269617336,-16.184347145014,-9.57570816684701)) ;
#56087=CARTESIAN_POINT('Ctrl Pts',(26.1054324306225,-16.1877442734701,-9.63701947062993)) ;
#56088=CARTESIAN_POINT('',(27.4875585758881,-15.9108618782029,-10.1676384740821)) ;
#56089=CARTESIAN_POINT('Ctrl Pts',(27.4875585758879,-15.9108618782028,-10.1676384740828)) ;
#56090=CARTESIAN_POINT('Ctrl Pts',(26.7875846204384,-16.0510971581644,-9.89877855202715)) ;
#56091=CARTESIAN_POINT('Ctrl Pts',(26.1054324308419,-16.1877442737199,-9.63701947038512)) ;
#56092=CARTESIAN_POINT('',(26.9481230865112,-15.9108618782029,-11.5215194621522)) ;
#56093=CARTESIAN_POINT('Origin',(-2.92277791062251E-15,-15.9108618782028,
0.)) ;
#56094=CARTESIAN_POINT('',(25.5797993342585,-16.1877442736409,-10.9562590645367)) ;
#56095=CARTESIAN_POINT('Ctrl Pts',(25.579799334239,-16.1877442737199,-10.9562590647496)) ;
#56096=CARTESIAN_POINT('Ctrl Pts',(26.2550503277099,-16.0510971581193,-11.2353388432409)) ;
#56097=CARTESIAN_POINT('Ctrl Pts',(26.9481230865116,-15.9108618782028,-11.5215194621516)) ;
#56098=CARTESIAN_POINT('',(26.1208051708581,-15.9108618823941,-13.2909850543146)) ;
#56099=CARTESIAN_POINT('Ctrl Pts',(25.579799334248,-16.1877442734701,-10.9562590644211)) ;
#56100=CARTESIAN_POINT('Ctrl Pts',(25.568123424087,-16.184347145014,-11.0296504108912)) ;
#56101=CARTESIAN_POINT('Ctrl Pts',(25.5589421180155,-16.1804174769264,-11.1037357887423)) ;
#56102=CARTESIAN_POINT('Ctrl Pts',(25.5523475266828,-16.1759680067789,-11.178166641881)) ;
#56103=CARTESIAN_POINT('Ctrl Pts',(25.5457529353466,-16.171518536629,-11.2525974950608)) ;
#56104=CARTESIAN_POINT('Ctrl Pts',(25.541745181025,-16.166549308068,-11.3273732006547)) ;
#56105=CARTESIAN_POINT('Ctrl Pts',(25.5403566338808,-16.1610860188908,-11.4021363221146)) ;
#56106=CARTESIAN_POINT('Ctrl Pts',(25.5390261782592,-16.1558512929189,-11.4737716394019)) ;
#56107=CARTESIAN_POINT('Ctrl Pts',(25.5400991249098,-16.1501596984484,-11.5454416108816)) ;
#56108=CARTESIAN_POINT('Ctrl Pts',(25.5435610181598,-16.1440425621063,-11.616831523354)) ;
#56109=CARTESIAN_POINT('Ctrl Pts',(25.5470300636165,-16.1379127878751,-11.6883689260482)) ;
#56110=CARTESIAN_POINT('Ctrl Pts',(25.5528978824486,-16.1313557844545,-11.7596246018672)) ;
#56111=CARTESIAN_POINT('Ctrl Pts',(25.5610987922911,-16.124412468004,-11.8302887546736)) ;
#56112=CARTESIAN_POINT('Ctrl Pts',(25.5672783132574,-16.1191805644219,-11.8835353605034)) ;
#56113=CARTESIAN_POINT('Ctrl Pts',(25.5747814590423,-16.1137295207042,-11.9364462043401)) ;
#56114=CARTESIAN_POINT('Ctrl Pts',(25.583561515064,-16.1080799337539,-11.9888939120546)) ;
#56115=CARTESIAN_POINT('Ctrl Pts',(25.594875159794,-16.1008000918636,-12.056476024346)) ;
#56116=CARTESIAN_POINT('Ctrl Pts',(25.6083124325426,-16.0931892946343,-12.1232980022537)) ;
#56117=CARTESIAN_POINT('Ctrl Pts',(25.6237302964865,-16.0853002129678,-12.1890767808231)) ;
#56118=CARTESIAN_POINT('Ctrl Pts',(25.6392738836098,-16.0773468007019,-12.2553919447961)) ;
#56119=CARTESIAN_POINT('Ctrl Pts',(25.6568302519724,-16.0691106491229,-12.3206463859086)) ;
#56120=CARTESIAN_POINT('Ctrl Pts',(25.6762064916025,-16.0606518030567,-12.3845755781982)) ;
#56121=CARTESIAN_POINT('Ctrl Pts',(25.6920743943232,-16.0537245483844,-12.4369295036055)) ;
#56122=CARTESIAN_POINT('Ctrl Pts',(25.709161848733,-16.046648082628,-12.4883950429174)) ;
#56123=CARTESIAN_POINT('Ctrl Pts',(25.7273420792229,-16.0394576303854,-12.5388423577954)) ;
#56124=CARTESIAN_POINT('Ctrl Pts',(25.7495783165907,-16.0306629892537,-12.6005444615625)) ;
#56125=CARTESIAN_POINT('Ctrl Pts',(25.7740208512851,-16.0214720150687,-12.6623053003954)) ;
#56126=CARTESIAN_POINT('Ctrl Pts',(25.8006914174555,-16.0119118209662,-12.7237889985167)) ;
#56127=CARTESIAN_POINT('Ctrl Pts',(25.8271435441353,-16.0024299275611,-12.784769127737)) ;
#56128=CARTESIAN_POINT('Ctrl Pts',(25.8557873490937,-15.9925848997544,-12.8454761456396)) ;
#56129=CARTESIAN_POINT('Ctrl Pts',(25.886593953266,-15.9824119250013,-12.9055877146238)) ;
#56130=CARTESIAN_POINT('Ctrl Pts',(25.9118892323843,-15.974058903214,-12.9549452779303)) ;
#56131=CARTESIAN_POINT('Ctrl Pts',(25.938641745247,-15.9654849570548,-13.0039013583173)) ;
#56132=CARTESIAN_POINT('Ctrl Pts',(25.9668102537101,-15.9567135267634,-13.0522837860431)) ;
#56133=CARTESIAN_POINT('Ctrl Pts',(26.0020990379238,-15.9457249040891,-13.1128960493439)) ;
#56134=CARTESIAN_POINT('Ctrl Pts',(26.0396164464604,-15.9344245943221,-13.1726164001282)) ;
#56135=CARTESIAN_POINT('Ctrl Pts',(26.079251847358,-15.9228603613878,-13.231147679351)) ;
#56136=CARTESIAN_POINT('Ctrl Pts',(26.0928557632711,-15.9188912113635,-13.2512371595329)) ;
#56137=CARTESIAN_POINT('Ctrl Pts',(26.1067087778732,-15.9148910240723,-13.2711867422769)) ;
#56138=CARTESIAN_POINT('Ctrl Pts',(26.1208051521851,-15.9108618900532,-13.2909850310201)) ;
#56139=CARTESIAN_POINT('',(25.6594598237771,-15.9108618960635,-14.1611741945452)) ;
#56140=CARTESIAN_POINT('Origin',(-2.92277791062251E-15,-15.9108618782028,
0.)) ;
#56141=CARTESIAN_POINT('',(23.4234276096246,-16.1877442736409,-15.0236076122497)) ;
#56142=CARTESIAN_POINT('Ctrl Pts',(25.6594598224132,-15.9108619316234,-14.1611741563844)) ;
#56143=CARTESIAN_POINT('Ctrl Pts',(25.5886682727421,-15.922600929087,-14.1595517042466)) ;
#56144=CARTESIAN_POINT('Ctrl Pts',(25.5179735150173,-15.9340937870887,-14.1603636010547)) ;
#56145=CARTESIAN_POINT('Ctrl Pts',(25.4476864284671,-15.9452906674734,-14.1635522014843)) ;
#56146=CARTESIAN_POINT('Ctrl Pts',(25.4235621279405,-15.9491337191721,-14.1646466095583)) ;
#56147=CARTESIAN_POINT('Ctrl Pts',(25.3994857899391,-15.9529419543585,-14.1660205563673)) ;
#56148=CARTESIAN_POINT('Ctrl Pts',(25.3754697336308,-15.9567135267634,-14.1676703300568)) ;
#56149=CARTESIAN_POINT('Ctrl Pts',(25.3075380506038,-15.9673817754482,-14.1723368707201)) ;
#56150=CARTESIAN_POINT('Ctrl Pts',(25.2400799043394,-15.977757691291,-14.1792146616279)) ;
#56151=CARTESIAN_POINT('Ctrl Pts',(25.1733919327092,-15.9877997661731,-14.1881868857565)) ;
#56152=CARTESIAN_POINT('Ctrl Pts',(25.1061606222867,-15.997923658641,-14.1972322108852)) ;
#56153=CARTESIAN_POINT('Ctrl Pts',(25.039712551615,-16.0077081692744,-14.2084060321102)) ;
#56154=CARTESIAN_POINT('Ctrl Pts',(24.9743326121174,-16.0171189356805,-14.2215395966218)) ;
#56155=CARTESIAN_POINT('Ctrl Pts',(24.9208299762537,-16.0248200870136,-14.2322872407014)) ;
#56156=CARTESIAN_POINT('Ctrl Pts',(24.8680423661167,-16.0322710948774,-14.2443462655726)) ;
#56157=CARTESIAN_POINT('Ctrl Pts',(24.8161134701842,-16.0394576303853,-14.2576018449788)) ;
#56158=CARTESIAN_POINT('Ctrl Pts',(24.7525766051236,-16.0482506141109,-14.2738205213998)) ;
#56159=CARTESIAN_POINT('Ctrl Pts',(24.6886963848685,-16.0568730319549,-14.2922476850668)) ;
#56160=CARTESIAN_POINT('Ctrl Pts',(24.6247998525748,-16.0652608298865,-14.3129372812856)) ;
#56161=CARTESIAN_POINT('Ctrl Pts',(24.5614270859275,-16.073579872281,-14.3334572830154)) ;
#56162=CARTESIAN_POINT('Ctrl Pts',(24.498038756358,-16.081668020051,-14.3562028166603)) ;
#56163=CARTESIAN_POINT('Ctrl Pts',(24.4349551708164,-16.0894673869312,-14.3811756315062)) ;
#56164=CARTESIAN_POINT('Ctrl Pts',(24.3831190588151,-16.0958761674669,-14.4016959240075)) ;
#56165=CARTESIAN_POINT('Ctrl Pts',(24.33148885998,-16.1020900207685,-14.4237191398173)) ;
#56166=CARTESIAN_POINT('Ctrl Pts',(24.2802393992345,-16.108079933754,-14.4472202082416)) ;
#56167=CARTESIAN_POINT('Ctrl Pts',(24.2160720625252,-16.1155796568302,-14.4766449270323)) ;
#56168=CARTESIAN_POINT('Ctrl Pts',(24.1524925012697,-16.1227292229209,-14.5083918874139)) ;
#56169=CARTESIAN_POINT('Ctrl Pts',(24.0898069063631,-16.1294814162038,-14.5423782205364)) ;
#56170=CARTESIAN_POINT('Ctrl Pts',(24.0272452522698,-16.1362202591735,-14.5762973565018)) ;
#56171=CARTESIAN_POINT('Ctrl Pts',(23.9655745075671,-16.142563213636,-14.6124468462664)) ;
#56172=CARTESIAN_POINT('Ctrl Pts',(23.9050814623739,-16.1484717649152,-14.6506961962637)) ;
#56173=CARTESIAN_POINT('Ctrl Pts',(23.8594603499876,-16.1529277264408,-14.6795421220946)) ;
#56174=CARTESIAN_POINT('Ctrl Pts',(23.8145087349089,-16.1571367885212,-14.7095813238667)) ;
#56175=CARTESIAN_POINT('Ctrl Pts',(23.7703405769757,-16.1610860188908,-14.7407407733971)) ;
#56176=CARTESIAN_POINT('Ctrl Pts',(23.7092391985723,-16.1665493080681,-14.7838461553213)) ;
#56177=CARTESIAN_POINT('Ctrl Pts',(23.6495972696092,-16.171518536629,-14.8291264882632)) ;
#56178=CARTESIAN_POINT('Ctrl Pts',(23.5916924706681,-16.1759680067789,-14.876354391028)) ;
#56179=CARTESIAN_POINT('Ctrl Pts',(23.5337876717589,-16.1804174769265,-14.9235822937668)) ;
#56180=CARTESIAN_POINT('Ctrl Pts',(23.4776204497978,-16.184347145014,-14.9727573155733)) ;
#56181=CARTESIAN_POINT('Ctrl Pts',(23.423427609523,-16.1877442734701,-15.0236076123058)) ;
#56182=CARTESIAN_POINT('',(24.659173012817,-15.9108618782029,-15.8389373042029)) ;
#56183=CARTESIAN_POINT('Ctrl Pts',(24.6591730128168,-15.9108618782028,-15.8389373042032)) ;
#56184=CARTESIAN_POINT('Ctrl Pts',(24.0333609963471,-16.0510971579214,-15.4258894690935)) ;
#56185=CARTESIAN_POINT('Ctrl Pts',(23.4234276097899,-16.1877442737199,-15.0236076121142)) ;
#56186=CARTESIAN_POINT('',(23.8413048334143,-15.9108618782029,-17.045202622519)) ;
#56187=CARTESIAN_POINT('Origin',(-2.92277791062251E-15,-15.9108618782028,
0.)) ;
#56188=CARTESIAN_POINT('',(22.6264860066069,-16.1877442736409,-16.199008539506)) ;
#56189=CARTESIAN_POINT('Ctrl Pts',(22.6264860065421,-16.1877442737199,-16.1990085397097)) ;
#56190=CARTESIAN_POINT('Ctrl Pts',(23.2259561029842,-16.0510971583948,-16.6167225905446)) ;
#56191=CARTESIAN_POINT('Ctrl Pts',(23.8413048334146,-15.9108618782028,-17.0452026225187)) ;
#56192=CARTESIAN_POINT('',(22.6529462781943,-15.9108618960635,-18.595449925547)) ;
#56193=CARTESIAN_POINT('Ctrl Pts',(22.6264860066214,-16.1877442734702,-16.1990085393908)) ;
#56194=CARTESIAN_POINT('Ctrl Pts',(22.5993061026931,-16.184347145014,-16.2681740614178)) ;
#56195=CARTESIAN_POINT('Ctrl Pts',(22.5744132841655,-16.1804174769265,-16.3385536548969)) ;
#56196=CARTESIAN_POINT('Ctrl Pts',(22.551972437449,-16.1759680067789,-16.4098267138495)) ;
#56197=CARTESIAN_POINT('Ctrl Pts',(22.5295315907202,-16.171518536629,-16.4810997728414)) ;
#56198=CARTESIAN_POINT('Ctrl Pts',(22.5095429691188,-16.1665493080681,-16.5532657152816)) ;
#56199=CARTESIAN_POINT('Ctrl Pts',(22.4921150243035,-16.1610860188908,-16.6259824199177)) ;
#56200=CARTESIAN_POINT('Ctrl Pts',(22.4754161983031,-16.155851292919,-16.6956569346638)) ;
#56201=CARTESIAN_POINT('Ctrl Pts',(22.4610571347385,-16.1501596984485,-16.7658819538511)) ;
#56202=CARTESIAN_POINT('Ctrl Pts',(22.4490913699374,-16.1440425621065,-16.8363470145571)) ;
#56203=CARTESIAN_POINT('Ctrl Pts',(22.4371008840904,-16.1379127878753,-16.9069576547587)) ;
#56204=CARTESIAN_POINT('Ctrl Pts',(22.4275136525808,-16.1313557844548,-16.9778088200711)) ;
#56205=CARTESIAN_POINT('Ctrl Pts',(22.4203321256725,-16.1244124680044,-17.048583837452)) ;
#56206=CARTESIAN_POINT('Ctrl Pts',(22.4149207265774,-16.1191805644222,-17.101913981571)) ;
#56207=CARTESIAN_POINT('Ctrl Pts',(22.4108741855918,-16.1137295207043,-17.1552007538358)) ;
#56208=CARTESIAN_POINT('Ctrl Pts',(22.4081742619674,-16.1080799337539,-17.2083097157992)) ;
#56209=CARTESIAN_POINT('Ctrl Pts',(22.4046952435411,-16.1008000918637,-17.2767438950482)) ;
#56210=CARTESIAN_POINT('Ctrl Pts',(22.4034536103134,-16.0931892946346,-17.3448922286831)) ;
#56211=CARTESIAN_POINT('Ctrl Pts',(22.4043705201805,-16.0853002129682,-17.4124475209615)) ;
#56212=CARTESIAN_POINT('Ctrl Pts',(22.4052949068825,-16.0773468007024,-17.4805536850181)) ;
#56213=CARTESIAN_POINT('Ctrl Pts',(22.4084130411773,-16.0691106491235,-17.5480566137945)) ;
#56214=CARTESIAN_POINT('Ctrl Pts',(22.4135933884833,-16.0606518030574,-17.6146564958564)) ;
#56215=CARTESIAN_POINT('Ctrl Pts',(22.4178357620649,-16.0537245483849,-17.6691975456164)) ;
#56216=CARTESIAN_POINT('Ctrl Pts',(22.4234601516448,-16.0466480826283,-17.7231331468177)) ;
#56217=CARTESIAN_POINT('Ctrl Pts',(22.4303706569622,-16.0394576303854,-17.7763092436615)) ;
#56218=CARTESIAN_POINT('Ctrl Pts',(22.4388228950485,-16.0306629892537,-17.8413489202666)) ;
#56219=CARTESIAN_POINT('Ctrl Pts',(22.449417222153,-16.0214720150687,-17.9069202474519)) ;
#56220=CARTESIAN_POINT('Ctrl Pts',(22.4622470676566,-16.0119118209662,-17.9726998742285)) ;
#56221=CARTESIAN_POINT('Ctrl Pts',(22.4749718330917,-16.0024299275611,-18.0379407472317)) ;
#56222=CARTESIAN_POINT('Ctrl Pts',(22.4898957474453,-15.9925848997544,-18.1033860401522)) ;
#56223=CARTESIAN_POINT('Ctrl Pts',(22.5070598998852,-15.9824119250013,-18.1687147433183)) ;
#56224=CARTESIAN_POINT('Ctrl Pts',(22.5211533723229,-15.974058903214,-18.2223560915107)) ;
#56225=CARTESIAN_POINT('Ctrl Pts',(22.5367563161497,-15.9654849570549,-18.2759186054106)) ;
#56226=CARTESIAN_POINT('Ctrl Pts',(22.5538654687518,-15.9567135267634,-18.3292252755273)) ;
#56227=CARTESIAN_POINT('Ctrl Pts',(22.5752993758999,-15.9457249040774,-18.396006503343)) ;
#56228=CARTESIAN_POINT('Ctrl Pts',(22.5991015382038,-15.934424594298,-18.462395759412)) ;
#56229=CARTESIAN_POINT('Ctrl Pts',(22.6252277906263,-15.9228603613509,-18.5280790495003)) ;
#56230=CARTESIAN_POINT('Ctrl Pts',(22.6341949792813,-15.9188912249891,-18.5506232109889)) ;
#56231=CARTESIAN_POINT('Ctrl Pts',(22.6434355147679,-15.9148910515742,-18.5730842951907)) ;
#56232=CARTESIAN_POINT('Ctrl Pts',(22.652946242239,-15.9108619316234,-18.5954499384048)) ;
#56233=CARTESIAN_POINT('',(22.0153220853233,-15.9108618949459,-19.3461191882741)) ;
#56234=CARTESIAN_POINT('Origin',(-2.92277791062251E-15,-15.9108618782028,
0.)) ;
#56235=CARTESIAN_POINT('',(19.6461693467839,-16.1877442736409,-19.7077085595375)) ;
#56236=CARTESIAN_POINT('Ctrl Pts',(22.0153220904288,-15.9108619279123,-19.3461191530285)) ;
#56237=CARTESIAN_POINT('Ctrl Pts',(21.9465343871962,-15.9226009254266,-19.3293165418211)) ;
#56238=CARTESIAN_POINT('Ctrl Pts',(21.8773178998704,-15.9340937834848,-19.314912173237)) ;
#56239=CARTESIAN_POINT('Ctrl Pts',(21.8079886315363,-15.9452906639308,-19.3029165795175)) ;
#56240=CARTESIAN_POINT('Ctrl Pts',(21.7841930710607,-15.9491337168317,-19.2987993879957)) ;
#56241=CARTESIAN_POINT('Ctrl Pts',(21.7603842591961,-15.9529419531996,-19.2949655104482)) ;
#56242=CARTESIAN_POINT('Ctrl Pts',(21.7365750250461,-15.9567135267635,-19.2914139700575)) ;
#56243=CARTESIAN_POINT('Ctrl Pts',(21.6692283787169,-15.9673817754483,-19.2813681057887)) ;
#56244=CARTESIAN_POINT('Ctrl Pts',(21.6018688446853,-15.9777576912911,-19.2735835903689)) ;
#56245=CARTESIAN_POINT('Ctrl Pts',(21.5348112378018,-15.9877997661733,-19.2680101062651)) ;
#56246=CARTESIAN_POINT('Ctrl Pts',(21.4672072805305,-15.9979236586412,-19.2623912123214)) ;
#56247=CARTESIAN_POINT('Ctrl Pts',(21.3999106875573,-16.0077081692748,-19.2590194248121)) ;
#56248=CARTESIAN_POINT('Ctrl Pts',(21.3332359665677,-16.0171189356809,-19.2577911795092)) ;
#56249=CARTESIAN_POINT('Ctrl Pts',(21.2786737668204,-16.0248200870139,-19.2567860644587)) ;
#56250=CARTESIAN_POINT('Ctrl Pts',(21.2245279677896,-16.0322710948776,-19.2572153802409)) ;
#56251=CARTESIAN_POINT('Ctrl Pts',(21.1709635828472,-16.0394576303854,-19.2589978739485)) ;
#56252=CARTESIAN_POINT('Ctrl Pts',(21.105425638374,-16.0482506141109,-19.261178818876)) ;
#56253=CARTESIAN_POINT('Ctrl Pts',(21.0390776066841,-16.0568730319549,-19.2654428066277)) ;
#56254=CARTESIAN_POINT('Ctrl Pts',(20.9722272882007,-16.0652608298865,-19.2719128259091)) ;
#56255=CARTESIAN_POINT('Ctrl Pts',(20.9059249478159,-16.073579872281,-19.2783298098581)) ;
#56256=CARTESIAN_POINT('Ctrl Pts',(20.8391289847859,-16.0816680200509,-19.2869169484544)) ;
#56257=CARTESIAN_POINT('Ctrl Pts',(20.7721518414175,-16.0894673869311,-19.2977448066129)) ;
#56258=CARTESIAN_POINT('Ctrl Pts',(20.7171163725964,-16.0958761674669,-19.3066421142631)) ;
#56259=CARTESIAN_POINT('Ctrl Pts',(20.661958918721,-16.1020900207685,-19.3170514729541)) ;
#56260=CARTESIAN_POINT('Ctrl Pts',(20.6068556068631,-16.108079933754,-19.3289859803214)) ;
#56261=CARTESIAN_POINT('Ctrl Pts',(20.5378630220768,-16.1155796568301,-19.3439286849187)) ;
#56262=CARTESIAN_POINT('Ctrl Pts',(20.4689452575836,-16.1227292229207,-19.3612656927369)) ;
#56263=CARTESIAN_POINT('Ctrl Pts',(20.4004191600592,-16.1294814162036,-19.3809818943453)) ;
#56264=CARTESIAN_POINT('Ctrl Pts',(20.3320285510829,-16.1362202591732,-19.4006591134401)) ;
#56265=CARTESIAN_POINT('Ctrl Pts',(20.264028562393,-16.1425632136357,-19.4227060610854)) ;
#56266=CARTESIAN_POINT('Ctrl Pts',(20.1967273313737,-16.1484717649149,-19.4470569459802)) ;
#56267=CARTESIAN_POINT('Ctrl Pts',(20.1459717938674,-16.1529277264406,-19.4654212794829)) ;
#56268=CARTESIAN_POINT('Ctrl Pts',(20.0956135821392,-16.1571367885211,-19.4850949129296)) ;
#56269=CARTESIAN_POINT('Ctrl Pts',(20.0457796906102,-16.1610860188908,-19.5060310234919)) ;
#56270=CARTESIAN_POINT('Ctrl Pts',(19.9768404455517,-16.166549308068,-19.5349936353278)) ;
#56271=CARTESIAN_POINT('Ctrl Pts',(19.9088589786387,-16.171518536629,-19.566394087524)) ;
#56272=CARTESIAN_POINT('Ctrl Pts',(19.8421553586711,-16.1759680067789,-19.6000700080484)) ;
#56273=CARTESIAN_POINT('Ctrl Pts',(19.7754517387401,-16.1804174769264,-19.6337459285543)) ;
#56274=CARTESIAN_POINT('Ctrl Pts',(19.7100264991306,-16.184347145014,-19.6696969732477)) ;
#56275=CARTESIAN_POINT('Ctrl Pts',(19.6461693466726,-16.1877442734701,-19.7077085595704)) ;
#56276=CARTESIAN_POINT('',(20.6777519263696,-15.9108618782029,-20.7696250296925)) ;
#56277=CARTESIAN_POINT('Ctrl Pts',(20.6777519263701,-15.9108618782028,-20.7696250296921)) ;
#56278=CARTESIAN_POINT('Ctrl Pts',(20.1553641257598,-16.0510971569168,-20.231702942616)) ;
#56279=CARTESIAN_POINT('Ctrl Pts',(19.6461693469744,-16.1877442737198,-19.7077085594409)) ;
#56280=CARTESIAN_POINT('',(19.619693664013,-15.9108618782029,-21.7718710526404)) ;
#56281=CARTESIAN_POINT('Origin',(-2.92277791062251E-15,-15.9108618782028,
0.)) ;
#56282=CARTESIAN_POINT('',(18.6151833408189,-16.1877442736409,-20.6843103790742)) ;
#56283=CARTESIAN_POINT('Ctrl Pts',(18.615183340712,-16.1877442737198,-20.6843103792592)) ;
#56284=CARTESIAN_POINT('Ctrl Pts',(19.1108419892473,-16.0510971575107,-21.2211268617121)) ;
#56285=CARTESIAN_POINT('Ctrl Pts',(19.6196936640126,-15.9108618782028,-21.7718710526408)) ;
#56286=CARTESIAN_POINT('',(18.1258609279823,-15.9108618949459,-23.0304124971064)) ;
#56287=CARTESIAN_POINT('Ctrl Pts',(18.6151833408578,-16.1877442734701,-20.6843103789648)) ;
#56288=CARTESIAN_POINT('Ctrl Pts',(18.5737703452616,-16.184347145014,-20.7460159736105)) ;
#56289=CARTESIAN_POINT('Ctrl Pts',(18.5343299748061,-16.1804174769264,-20.8093989111475)) ;
#56290=CARTESIAN_POINT('Ctrl Pts',(18.497092181757,-16.1759680067789,-20.8741815268916)) ;
#56291=CARTESIAN_POINT('Ctrl Pts',(18.4598543886874,-16.171518536629,-20.9389641426714)) ;
#56292=CARTESIAN_POINT('Ctrl Pts',(18.4248195455368,-16.166549308068,-21.0051459226955)) ;
#56293=CARTESIAN_POINT('Ctrl Pts',(18.39216711438,-16.1610860188908,-21.0724160582175)) ;
#56294=CARTESIAN_POINT('Ctrl Pts',(18.3608807365454,-16.155851292919,-21.1368718675514)) ;
#56295=CARTESIAN_POINT('Ctrl Pts',(18.3317610766189,-16.1501596984485,-21.2023682905993)) ;
#56296=CARTESIAN_POINT('Ctrl Pts',(18.30492715963,-16.1440425621065,-21.2686136316174)) ;
#56297=CARTESIAN_POINT('Ctrl Pts',(18.2780378042711,-16.1379127878753,-21.3349958342692)) ;
#56298=CARTESIAN_POINT('Ctrl Pts',(18.2534438107098,-16.1313557844548,-21.4021295673313)) ;
#56299=CARTESIAN_POINT('Ctrl Pts',(18.2312156472675,-16.1244124680044,-21.4697060881353)) ;
#56300=CARTESIAN_POINT('Ctrl Pts',(18.2144663591183,-16.1191805644222,-21.5206261122753)) ;
#56301=CARTESIAN_POINT('Ctrl Pts',(18.199059343121,-16.1137295207043,-21.5717971827197)) ;
#56302=CARTESIAN_POINT('Ctrl Pts',(18.1850056852781,-16.1080799337539,-21.6230840828956)) ;
#56303=CARTESIAN_POINT('Ctrl Pts',(18.1668966787307,-16.1008000918638,-21.6891704229405)) ;
#56304=CARTESIAN_POINT('Ctrl Pts',(18.1510341969168,-16.0931892946346,-21.7554585719638)) ;
#56305=CARTESIAN_POINT('Ctrl Pts',(18.1374072790211,-16.0853002129682,-21.8216315675676)) ;
#56306=CARTESIAN_POINT('Ctrl Pts',(18.1236692420074,-16.0773468007025,-21.8883441631719)) ;
#56307=CARTESIAN_POINT('Ctrl Pts',(18.1122033417405,-16.0691106491235,-21.9549392176873)) ;
#56308=CARTESIAN_POINT('Ctrl Pts',(18.1029455694405,-16.0606518030575,-22.0210956530574)) ;
#56309=CARTESIAN_POINT('Ctrl Pts',(18.0953640452087,-16.053724548385,-22.0752735482998)) ;
#56310=CARTESIAN_POINT('Ctrl Pts',(18.0892623797524,-16.0466480826283,-22.129157242622)) ;
#56311=CARTESIAN_POINT('Ctrl Pts',(18.0845800323485,-16.0394576303854,-22.1825756662427)) ;
#56312=CARTESIAN_POINT('Ctrl Pts',(18.0788530538943,-16.0306629892537,-22.2479117326944)) ;
#56313=CARTESIAN_POINT('Ctrl Pts',(18.0751037944482,-16.0214720150686,-22.3142275058505)) ;
#56314=CARTESIAN_POINT('Ctrl Pts',(18.0734930099685,-16.0119118209661,-22.3812272790436)) ;
#56315=CARTESIAN_POINT('Ctrl Pts',(18.0718954182698,-16.0024299275609,-22.4476783051183)) ;
#56316=CARTESIAN_POINT('Ctrl Pts',(18.0724016163703,-15.9925848997542,-22.5148017238976)) ;
#56317=CARTESIAN_POINT('Ctrl Pts',(18.0751207403865,-15.9824119250011,-22.5822928636936)) ;
#56318=CARTESIAN_POINT('Ctrl Pts',(18.0773534110361,-15.9740589032138,-22.6377097869478)) ;
#56319=CARTESIAN_POINT('Ctrl Pts',(18.081077209515,-15.9654849570548,-22.6933742107403)) ;
#56320=CARTESIAN_POINT('Ctrl Pts',(18.0863270012958,-15.9567135267635,-22.7491125625987)) ;
#56321=CARTESIAN_POINT('Ctrl Pts',(18.0929038056638,-15.9457249040785,-22.8189401388673)) ;
#56322=CARTESIAN_POINT('Ctrl Pts',(18.1018777590367,-15.9344245943002,-22.8888940123242)) ;
#56323=CARTESIAN_POINT('Ctrl Pts',(18.1132732284097,-15.9228603613543,-22.9586580355687)) ;
#56324=CARTESIAN_POINT('Ctrl Pts',(18.1171844420595,-15.9188912237728,-22.9826028149406)) ;
#56325=CARTESIAN_POINT('Ctrl Pts',(18.1213804711799,-15.9148910491191,-23.0065252208016)) ;
#56326=CARTESIAN_POINT('Ctrl Pts',(18.125860892512,-15.9108619279123,-23.0304125002962)) ;
#56327=CARTESIAN_POINT('',(17.3417723053832,-15.9108618962294,-23.6264611434763)) ;
#56328=CARTESIAN_POINT('Origin',(-2.92277791062251E-15,-15.9108618782028,
0.)) ;
#56329=CARTESIAN_POINT('',(14.9502780404355,-16.1877442736409,-23.4702989581266)) ;
#56330=CARTESIAN_POINT('Ctrl Pts',(17.3417723204951,-15.9108619321403,-23.6264611079952)) ;
#56331=CARTESIAN_POINT('Ctrl Pts',(17.2782049000365,-15.9226009295966,-23.595264010192)) ;
#56332=CARTESIAN_POINT('Ctrl Pts',(17.2137031689819,-15.9340937875903,-23.5663169095397)) ;
#56333=CARTESIAN_POINT('Ctrl Pts',(17.1485734783208,-15.9452906679664,-23.5396980233582)) ;
#56334=CARTESIAN_POINT('Ctrl Pts',(17.1262193270725,-15.9491337194978,-23.5305617507654)) ;
#56335=CARTESIAN_POINT('Ctrl Pts',(17.1037913301717,-15.9529419545198,-23.5216993195756)) ;
#56336=CARTESIAN_POINT('Ctrl Pts',(17.0813022267581,-15.9567135267635,-23.5131125336849)) ;
#56337=CARTESIAN_POINT('Ctrl Pts',(17.0176896714601,-15.9673817754481,-23.4888239979325)) ;
#56338=CARTESIAN_POINT('Ctrl Pts',(16.9535784066094,-15.9777576912908,-23.4667411714743)) ;
#56339=CARTESIAN_POINT('Ctrl Pts',(16.8892867036426,-15.9877997661728,-23.4468825890607)) ;
#56340=CARTESIAN_POINT('Ctrl Pts',(16.8244711854299,-15.9979236586406,-23.4268622092806)) ;
#56341=CARTESIAN_POINT('Ctrl Pts',(16.7594727840492,-16.007708169274,-23.4091024740735)) ;
#56342=CARTESIAN_POINT('Ctrl Pts',(16.6946209174192,-16.01711893568,-23.3935698503413)) ;
#56343=CARTESIAN_POINT('Ctrl Pts',(16.641550421604,-16.0248200870133,-23.380858974223)) ;
#56344=CARTESIAN_POINT('Ctrl Pts',(16.5885782310602,-16.0322710948773,-23.369638506587)) ;
#56345=CARTESIAN_POINT('Ctrl Pts',(16.5358829682124,-16.0394576303854,-23.3598645671712)) ;
#56346=CARTESIAN_POINT('Ctrl Pts',(16.4714084257695,-16.0482506141109,-23.3479058020443)) ;
#56347=CARTESIAN_POINT('Ctrl Pts',(16.4056949428662,-16.056873031955,-23.3378072345523)) ;
#56348=CARTESIAN_POINT('Ctrl Pts',(16.3390166847862,-16.0652608298866,-23.3297551459858)) ;
#56349=CARTESIAN_POINT('Ctrl Pts',(16.2728849944109,-16.0735798722809,-23.3217690611166)) ;
#56350=CARTESIAN_POINT('Ctrl Pts',(16.2058047029135,-16.0816680200509,-23.3157962796076)) ;
#56351=CARTESIAN_POINT('Ctrl Pts',(16.1380657785028,-16.089467386931,-23.3119728824655)) ;
#56352=CARTESIAN_POINT('Ctrl Pts',(16.0824043502165,-16.0958761674667,-23.3088311770475)) ;
#56353=CARTESIAN_POINT('Ctrl Pts',(16.0262987425406,-16.1020900207685,-23.3071399485763)) ;
#56354=CARTESIAN_POINT('Ctrl Pts',(15.9699181491897,-16.108079933754,-23.3069498505863)) ;
#56355=CARTESIAN_POINT('Ctrl Pts',(15.8993263329097,-16.1155796568302,-23.3067118367311)) ;
#56356=CARTESIAN_POINT('Ctrl Pts',(15.8282928832485,-16.1227292229209,-23.3088282327695)) ;
#56357=CARTESIAN_POINT('Ctrl Pts',(15.7571304872636,-16.1294814162039,-23.3133523951902)) ;
#56358=CARTESIAN_POINT('Ctrl Pts',(15.686108792268,-16.1362202591736,-23.3178676125195)) ;
#56359=CARTESIAN_POINT('Ctrl Pts',(15.6149591634837,-16.1425632136361,-23.3247811272778)) ;
#56360=CARTESIAN_POINT('Ctrl Pts',(15.5439966773993,-16.1484717649153,-23.334094926757)) ;
#56361=CARTESIAN_POINT('Ctrl Pts',(15.4904799872992,-16.1529277264409,-23.3411189721067)) ;
#56362=CARTESIAN_POINT('Ctrl Pts',(15.437069872936,-16.1571367885212,-23.3495071199925)) ;
#56363=CARTESIAN_POINT('Ctrl Pts',(15.3839004251958,-16.1610860188908,-23.3592409423245)) ;
#56364=CARTESIAN_POINT('Ctrl Pts',(15.3103468359604,-16.1665493080681,-23.3727065245325)) ;
#56365=CARTESIAN_POINT('Ctrl Pts',(15.2372045689343,-16.171518536629,-23.3887588457374)) ;
#56366=CARTESIAN_POINT('Ctrl Pts',(15.1648211150739,-16.1759680067789,-23.407308135406)) ;
#56367=CARTESIAN_POINT('Ctrl Pts',(15.0924376612533,-16.1804174769264,-23.4258574250643)) ;
#56368=CARTESIAN_POINT('Ctrl Pts',(15.0208136154844,-16.184347145014,-23.4469034617514)) ;
#56369=CARTESIAN_POINT('Ctrl Pts',(14.9502780403199,-16.1877442734702,-23.4702989581348)) ;
#56370=CARTESIAN_POINT('',(15.7294621415156,-15.9108618782029,-24.7291481725744)) ;
#56371=CARTESIAN_POINT('Ctrl Pts',(15.7294621415156,-15.9108618782028,-24.7291481725744)) ;
#56372=CARTESIAN_POINT('Ctrl Pts',(15.3349248241001,-16.0510971573237,-24.0915044676574)) ;
#56373=CARTESIAN_POINT('Ctrl Pts',(14.9502780406423,-16.1877442737198,-23.4702989580733)) ;
#56374=CARTESIAN_POINT('',(14.4806874246062,-15.9108618782029,-25.4805109900364)) ;
#56375=CARTESIAN_POINT('Origin',(-2.92277791062251E-15,-15.9108618782028,
0.)) ;
#56376=CARTESIAN_POINT('',(13.7334553913052,-16.1877442736409,-24.2024368542756)) ;
#56377=CARTESIAN_POINT('Ctrl Pts',(13.7334553911612,-16.1877442737199,-24.2024368544333)) ;
#56378=CARTESIAN_POINT('Ctrl Pts',(14.102126141797,-16.0510971569896,-24.8332548261164)) ;
#56379=CARTESIAN_POINT('Ctrl Pts',(14.4806874246063,-15.9108618782028,-25.4805109900364)) ;
#56380=CARTESIAN_POINT('',(12.751230463362,-15.9108618962294,-26.3884985273164)) ;
#56381=CARTESIAN_POINT('Ctrl Pts',(13.7334553913666,-16.1877442734702,-24.2024368541772)) ;
#56382=CARTESIAN_POINT('Ctrl Pts',(13.6797457297494,-16.184347145014,-24.2537972364167)) ;
#56383=CARTESIAN_POINT('Ctrl Pts',(13.6276019952533,-16.1804174769265,-24.3072198022979)) ;
#56384=CARTESIAN_POINT('Ctrl Pts',(13.5773084536876,-16.1759680067789,-24.3624828117221)) ;
#56385=CARTESIAN_POINT('Ctrl Pts',(13.5270149120943,-16.171518536629,-24.4177458211767)) ;
#56386=CARTESIAN_POINT('Ctrl Pts',(13.4785720377215,-16.166549308068,-24.4748488523071)) ;
#56387=CARTESIAN_POINT('Ctrl Pts',(13.4322219116136,-16.1610860188908,-24.5335269419437)) ;
#56388=CARTESIAN_POINT('Ctrl Pts',(13.3878108982001,-16.155851292919,-24.5897501638582)) ;
#56389=CARTESIAN_POINT('Ctrl Pts',(13.3452922448459,-16.1501596984486,-24.6474554508189)) ;
#56390=CARTESIAN_POINT('Ctrl Pts',(13.3048448998038,-16.1440425621066,-24.7063835136293)) ;
#56391=CARTESIAN_POINT('Ctrl Pts',(13.2643139913044,-16.1379127878754,-24.7654333207137)) ;
#56392=CARTESIAN_POINT('Ctrl Pts',(13.2258632234961,-16.1313557844549,-24.825710522781)) ;
#56393=CARTESIAN_POINT('Ctrl Pts',(13.1896277877376,-16.1244124680045,-24.8869287440011)) ;
#56394=CARTESIAN_POINT('Ctrl Pts',(13.1623237886324,-16.1191805644222,-24.9330576844272)) ;
#56395=CARTESIAN_POINT('Ctrl Pts',(13.1362767125676,-16.1137295207044,-24.9797203506699)) ;
#56396=CARTESIAN_POINT('Ctrl Pts',(13.1115264539273,-16.1080799337539,-25.0267870706076)) ;
#56397=CARTESIAN_POINT('Ctrl Pts',(13.0796342162779,-16.1008000918637,-25.0874354476383)) ;
#56398=CARTESIAN_POINT('Ctrl Pts',(13.0498925978974,-16.0931892946345,-25.1487638518767)) ;
#56399=CARTESIAN_POINT('Ctrl Pts',(13.0223590317742,-16.0853002129681,-25.210460375078)) ;
#56400=CARTESIAN_POINT('Ctrl Pts',(12.9946009463867,-16.0773468007023,-25.2726599954059)) ;
#56401=CARTESIAN_POINT('Ctrl Pts',(12.9690871443112,-16.0691106491233,-25.3352332649269)) ;
#56402=CARTESIAN_POINT('Ctrl Pts',(12.9458241355485,-16.0606518030571,-25.3978528522157)) ;
#56403=CARTESIAN_POINT('Ctrl Pts',(12.9267732171505,-16.0537245483847,-25.449134294772)) ;
#56404=CARTESIAN_POINT('Ctrl Pts',(12.9092308037536,-16.0466480826282,-25.5004465405545)) ;
#56405=CARTESIAN_POINT('Ctrl Pts',(12.8931745449892,-16.0394576303854,-25.5516095048324)) ;
#56406=CARTESIAN_POINT('Ctrl Pts',(12.8735361371421,-16.0306629892538,-25.6141869192784)) ;
#56407=CARTESIAN_POINT('Ctrl Pts',(12.8556186023503,-16.0214720150688,-25.6781462865562)) ;
#56408=CARTESIAN_POINT('Ctrl Pts',(12.8396425063793,-16.0119118209664,-25.743233371235)) ;
#56409=CARTESIAN_POINT('Ctrl Pts',(12.823797259159,-16.0024299275613,-25.8077873742565)) ;
#56410=CARTESIAN_POINT('Ctrl Pts',(12.8098620717459,-15.9925848997546,-25.8734503024339)) ;
#56411=CARTESIAN_POINT('Ctrl Pts',(12.7980090241213,-15.9824119250016,-25.9399480681732)) ;
#56412=CARTESIAN_POINT('Ctrl Pts',(12.7882764957844,-15.9740589032142,-25.9945493327509)) ;
#56413=CARTESIAN_POINT('Ctrl Pts',(12.7799470282373,-15.9654849570549,-26.049712859848)) ;
#56414=CARTESIAN_POINT('Ctrl Pts',(12.7730919847679,-15.9567135267634,-26.1052766300655)) ;
#56415=CARTESIAN_POINT('Ctrl Pts',(12.7645041622943,-15.9457249040773,-26.1748854949425)) ;
#56416=CARTESIAN_POINT('Ctrl Pts',(12.7582302946523,-15.9344245942978,-26.2451330204268)) ;
#56417=CARTESIAN_POINT('Ctrl Pts',(12.7543621414963,-15.9228603613505,-26.3157156886516)) ;
#56418=CARTESIAN_POINT('Ctrl Pts',(12.7530344938471,-15.9188912251586,-26.3399414392269)) ;
#56419=CARTESIAN_POINT('Ctrl Pts',(12.7519898122864,-15.9148910519162,-26.364206566251)) ;
#56420=CARTESIAN_POINT('Ctrl Pts',(12.7512304249355,-15.9108619321403,-26.3884985240483)) ;
#56421=CARTESIAN_POINT('',(11.8573408058245,-15.9108618828344,-26.8020561960657)) ;
#56422=CARTESIAN_POINT('Origin',(-2.92277791062251E-15,-15.9108618782028,
0.)) ;
#56423=CARTESIAN_POINT('',(9.55532834895734,-16.1877442736409,-26.1354442627971)) ;
#56424=CARTESIAN_POINT('Ctrl Pts',(11.8573407877332,-15.9108618871751,-26.8020561755759)) ;
#56425=CARTESIAN_POINT('Ctrl Pts',(11.8019659957108,-15.9226008852454,-26.7579233271853)) ;
#56426=CARTESIAN_POINT('Ctrl Pts',(11.7451950535357,-15.934093743921,-26.7157870228874)) ;
#56427=CARTESIAN_POINT('Ctrl Pts',(11.6873103354369,-15.9452906250395,-26.675789507789)) ;
#56428=CARTESIAN_POINT('Ctrl Pts',(11.6674427673654,-15.949133691139,-26.6620613014505)) ;
#56429=CARTESIAN_POINT('Ctrl Pts',(11.6474442112849,-15.9529419404769,-26.6485846614785)) ;
#56430=CARTESIAN_POINT('Ctrl Pts',(11.6273267208508,-15.9567135267634,-26.635364088185)) ;
#56431=CARTESIAN_POINT('Ctrl Pts',(11.5704227089682,-15.9673817754481,-26.5979685858856)) ;
#56432=CARTESIAN_POINT('Ctrl Pts',(11.5125574847872,-15.9777576912908,-26.562620016811)) ;
#56433=CARTESIAN_POINT('Ctrl Pts',(11.4540378943115,-15.9877997661729,-26.5294049013298)) ;
#56434=CARTESIAN_POINT('Ctrl Pts',(11.3950415167503,-15.9979236586407,-26.4959191664206)) ;
#56435=CARTESIAN_POINT('Ctrl Pts',(11.335380559969,-16.007708169274,-26.4646019089955)) ;
#56436=CARTESIAN_POINT('Ctrl Pts',(11.2753839489031,-16.0171189356801,-26.4354911950566)) ;
#56437=CARTESIAN_POINT('Ctrl Pts',(11.2262866744231,-16.0248200870134,-26.4116689043108)) ;
#56438=CARTESIAN_POINT('Ctrl Pts',(11.1769650131244,-16.0322710948773,-26.3893233098529)) ;
#56439=CARTESIAN_POINT('Ctrl Pts',(11.1276028442977,-16.0394576303854,-26.3684499558578)) ;
#56440=CARTESIAN_POINT('Ctrl Pts',(11.0672064618319,-16.0482506141109,-26.3429106592426)) ;
#56441=CARTESIAN_POINT('Ctrl Pts',(11.0052002171405,-16.0568730319549,-26.3189217342993)) ;
#56442=CARTESIAN_POINT('Ctrl Pts',(10.9418118207047,-16.0652608298865,-26.2967240445969)) ;
#56443=CARTESIAN_POINT('Ctrl Pts',(10.87894302468,-16.0735798722809,-26.274708311362)) ;
#56444=CARTESIAN_POINT('Ctrl Pts',(10.8147150045907,-16.0816680200509,-26.2544548903729)) ;
#56445=CARTESIAN_POINT('Ctrl Pts',(10.7493816959561,-16.089467386931,-26.2361590157312)) ;
#56446=CARTESIAN_POINT('Ctrl Pts',(10.6956969747283,-16.0958761674668,-26.2211251998985)) ;
#56447=CARTESIAN_POINT('Ctrl Pts',(10.6412666491104,-16.1020900207684,-26.2074124642288)) ;
#56448=CARTESIAN_POINT('Ctrl Pts',(10.5862450681494,-16.1080799337539,-26.1951066496522)) ;
#56449=CARTESIAN_POINT('Ctrl Pts',(10.51735481525,-16.11557965683,-26.1796990466079)) ;
#56450=CARTESIAN_POINT('Ctrl Pts',(10.4475271255812,-16.1227292229206,-26.1664958705399)) ;
#56451=CARTESIAN_POINT('Ctrl Pts',(10.3770559056829,-16.1294814162034,-26.155616448966)) ;
#56452=CARTESIAN_POINT('Ctrl Pts',(10.3067240201933,-16.136220259173,-26.1447585379858)) ;
#56453=CARTESIAN_POINT('Ctrl Pts',(10.2357516288819,-16.1425632136355,-26.1362153515903)) ;
#56454=CARTESIAN_POINT('Ctrl Pts',(10.1644460147151,-16.1484717649146,-26.1300565627414)) ;
#56455=CARTESIAN_POINT('Ctrl Pts',(10.1106705529661,-16.1529277264404,-26.1254118833843)) ;
#56456=CARTESIAN_POINT('Ctrl Pts',(10.0567059335498,-16.157136788521,-26.1221223252373)) ;
#56457=CARTESIAN_POINT('Ctrl Pts',(10.0026870738765,-16.1610860188908,-26.1201987166258)) ;
#56458=CARTESIAN_POINT('Ctrl Pts',(9.92795842454788,-16.166549308068,-26.1175376335476)) ;
#56459=CARTESIAN_POINT('Ctrl Pts',(9.85307540852308,-16.171518536629,-26.1174912350626)) ;
#56460=CARTESIAN_POINT('Ctrl Pts',(9.77839669062397,-16.1759680067789,-26.1200465497064)) ;
#56461=CARTESIAN_POINT('Ctrl Pts',(9.70371797276597,-16.1804174769265,-26.1226018643487)) ;
#56462=CARTESIAN_POINT('Ctrl Pts',(9.62924418161368,-16.184347145014,-26.1277588037449)) ;
#56463=CARTESIAN_POINT('Ctrl Pts',(9.55532834884255,-16.1877442734701,-26.1354442627804)) ;
#56464=CARTESIAN_POINT('',(10.0456801889655,-15.9108618782028,-27.532363831381)) ;
#56465=CARTESIAN_POINT('Ctrl Pts',(10.0456801889651,-15.9108618782028,-27.5323638313812)) ;
#56466=CARTESIAN_POINT('Ctrl Pts',(9.79744148248229,-16.0510971574616,-26.8248140204399)) ;
#56467=CARTESIAN_POINT('Ctrl Pts',(9.55532834917085,-16.1877442737199,-26.1354442627893)) ;
#56468=CARTESIAN_POINT('',(8.66458033535308,-15.9108618782028,-27.9977105530921)) ;
#56469=CARTESIAN_POINT('Origin',(-2.92277791062251E-15,-15.9108618782028,
0.)) ;
#56470=CARTESIAN_POINT('',(8.209566331333,-16.1877442736409,-26.5888842812483)) ;
#56471=CARTESIAN_POINT('Ctrl Pts',(8.20956633115831,-16.1877442737199,-26.5888842813713)) ;
#56472=CARTESIAN_POINT('Ctrl Pts',(8.43401054640113,-16.0510971576296,-27.2842073897287)) ;
#56473=CARTESIAN_POINT('Ctrl Pts',(8.66458033535351,-15.9108618782028,-27.997710553092)) ;
#56474=CARTESIAN_POINT('',(6.78036653080776,-15.9108618828344,-28.5126880007908)) ;
#56475=CARTESIAN_POINT('Ctrl Pts',(8.20956633141424,-16.1877442734701,-26.5888842811654)) ;
#56476=CARTESIAN_POINT('Ctrl Pts',(8.14607140785912,-16.184347145014,-26.6274978966082)) ;
#56477=CARTESIAN_POINT('Ctrl Pts',(8.08366249239415,-16.1804174769265,-26.6684621110277)) ;
#56478=CARTESIAN_POINT('Ctrl Pts',(8.02266487241838,-16.1759680067789,-26.7116214772316)) ;
#56479=CARTESIAN_POINT('Ctrl Pts',(7.96166725240905,-16.171518536629,-26.7547808434592)) ;
#56480=CARTESIAN_POINT('Ctrl Pts',(7.90208148177934,-16.166549308068,-26.8001350514255)) ;
#56481=CARTESIAN_POINT('Ctrl Pts',(7.84420094110269,-16.1610860188908,-26.8474773729212)) ;
#56482=CARTESIAN_POINT('Ctrl Pts',(7.78874190173793,-16.155851292919,-26.8928390720476)) ;
#56483=CARTESIAN_POINT('Ctrl Pts',(7.73481237993059,-16.1501596984485,-26.9400549878379)) ;
#56484=CARTESIAN_POINT('Ctrl Pts',(7.68264287973525,-16.1440425621065,-26.9889103617178)) ;
#56485=CARTESIAN_POINT('Ctrl Pts',(7.63036559832969,-16.1379127878753,-27.0378666698851)) ;
#56486=CARTESIAN_POINT('Ctrl Pts',(7.57985597144212,-16.1313557844548,-27.0884688459826)) ;
#56487=CARTESIAN_POINT('Ctrl Pts',(7.53130759207052,-16.1244124680044,-27.1404662716341)) ;
#56488=CARTESIAN_POINT('Ctrl Pts',(7.49472558666167,-16.1191805644222,-27.1796471903599)) ;
#56489=CARTESIAN_POINT('Ctrl Pts',(7.4592563828573,-16.1137295207043,-27.2196195579886)) ;
#56490=CARTESIAN_POINT('Ctrl Pts',(7.42496681800598,-16.1080799337539,-27.260265310174)) ;
#56491=CARTESIAN_POINT('Ctrl Pts',(7.38078259484197,-16.1008000918638,-27.3126398734855)) ;
#56492=CARTESIAN_POINT('Ctrl Pts',(7.33855252491512,-16.0931892946346,-27.3661408849174)) ;
#56493=CARTESIAN_POINT('Ctrl Pts',(7.29839974951543,-16.0853002129682,-27.4204760748612)) ;
#56494=CARTESIAN_POINT('Ctrl Pts',(7.25791955297621,-16.0773468007025,-27.4752543347953)) ;
#56495=CARTESIAN_POINT('Ctrl Pts',(7.21955084612071,-16.0691106491236,-27.5308799627835)) ;
#56496=CARTESIAN_POINT('Ctrl Pts',(7.18337035333025,-16.0606518030575,-27.5870346796851)) ;
#56497=CARTESIAN_POINT('Ctrl Pts',(7.15374084053614,-16.053724548385,-27.6330218062984)) ;
#56498=CARTESIAN_POINT('Ctrl Pts',(7.12557794295134,-16.0466480826283,-27.6793632999596)) ;
#56499=CARTESIAN_POINT('Ctrl Pts',(7.09889854564046,-16.0394576303854,-27.7258784815505)) ;
#56500=CARTESIAN_POINT('Ctrl Pts',(7.06626697852494,-16.0306629892538,-27.7827711936417)) ;
#56501=CARTESIAN_POINT('Ctrl Pts',(7.03501897240025,-16.0214720150688,-27.8413834861136)) ;
#56502=CARTESIAN_POINT('Ctrl Pts',(7.00542458942953,-16.0119118209664,-27.9015144825385)) ;
#56503=CARTESIAN_POINT('Ctrl Pts',(6.97607259283704,-16.0024299275613,-27.9611529890723)) ;
#56504=CARTESIAN_POINT('Ctrl Pts',(6.94834761378586,-15.9925848997547,-28.0222851011058)) ;
#56505=CARTESIAN_POINT('Ctrl Pts',(6.92247662985391,-15.9824119250017,-28.0846801311699)) ;
#56506=CARTESIAN_POINT('Ctrl Pts',(6.90123398473867,-15.9740589032142,-28.1359126426234)) ;
#56507=CARTESIAN_POINT('Ctrl Pts',(6.88124072781037,-15.965484957055,-28.1879958878066)) ;
#56508=CARTESIAN_POINT('Ctrl Pts',(6.86260138330431,-15.9567135267634,-28.2407869762416)) ;
#56509=CARTESIAN_POINT('Ctrl Pts',(6.83925049104925,-15.9457249040898,-28.306922296487)) ;
#56510=CARTESIAN_POINT('Ctrl Pts',(6.81802216149098,-15.9344245943236,-28.3741787776958)) ;
#56511=CARTESIAN_POINT('Ctrl Pts',(6.79907125636311,-15.9228603613902,-28.4422797236946)) ;
#56512=CARTESIAN_POINT('Ctrl Pts',(6.79256680389258,-15.91889121042,-28.4656537717128)) ;
#56513=CARTESIAN_POINT('Ctrl Pts',(6.78633023914337,-15.9148910221682,-28.4891271056646)) ;
#56514=CARTESIAN_POINT('Ctrl Pts',(6.78036653281026,-15.9108618871751,-28.5126879735306)) ;
#56515=CARTESIAN_POINT('',(5.8184729570234,-15.9108618818334,-28.7244167966786)) ;
#56516=CARTESIAN_POINT('Origin',(-2.92277791062251E-15,-15.9108618782028,
0.)) ;
#56517=CARTESIAN_POINT('',(3.71358212386679,-16.1877442736409,-27.5785252411991)) ;
#56518=CARTESIAN_POINT('Ctrl Pts',(5.81847294179667,-15.9108618853164,-28.7244167739446)) ;
#56519=CARTESIAN_POINT('Ctrl Pts',(5.77388003967716,-15.9226008834119,-28.6694117834359)) ;
#56520=CARTESIAN_POINT('Ctrl Pts',(5.72749443064539,-15.9340937421156,-28.6160565279039)) ;
#56521=CARTESIAN_POINT('Ctrl Pts',(5.67956130868255,-15.9452906232646,-28.5645506289581)) ;
#56522=CARTESIAN_POINT('Ctrl Pts',(5.66310938939528,-15.9491336899665,-28.5468724378123)) ;
#56523=CARTESIAN_POINT('Ctrl Pts',(5.64647546513558,-15.9529419398963,-28.529411773067)) ;
#56524=CARTESIAN_POINT('Ctrl Pts',(5.62967034032204,-15.9567135267634,-28.5121756210024)) ;
#56525=CARTESIAN_POINT('Ctrl Pts',(5.58213564020621,-15.9673817754481,-28.4634217242814)) ;
#56526=CARTESIAN_POINT('Ctrl Pts',(5.53322217026505,-15.9777576912908,-28.416460272393)) ;
#56527=CARTESIAN_POINT('Ctrl Pts',(5.48321100329122,-15.9877997661729,-28.3714417257282)) ;
#56528=CARTESIAN_POINT('Ctrl Pts',(5.43279237142662,-15.9979236586408,-28.3260563914375)) ;
#56529=CARTESIAN_POINT('Ctrl Pts',(5.38125853927543,-16.0077081692742,-28.2826459719449)) ;
#56530=CARTESIAN_POINT('Ctrl Pts',(5.3289225586257,-16.0171189356802,-28.2413183524286)) ;
#56531=CARTESIAN_POINT('Ctrl Pts',(5.28609423946784,-16.0248200870134,-28.2074985508943)) ;
#56532=CARTESIAN_POINT('Ctrl Pts',(5.24272933347944,-16.0322710948773,-28.175072684776)) ;
#56533=CARTESIAN_POINT('Ctrl Pts',(5.19900837882614,-16.0394576303854,-28.1440759310355)) ;
#56534=CARTESIAN_POINT('Ctrl Pts',(5.1455142240551,-16.048250614111,-28.1061502920567)) ;
#56535=CARTESIAN_POINT('Ctrl Pts',(5.09011456066198,-16.0568730319551,-28.0693927051302)) ;
#56536=CARTESIAN_POINT('Ctrl Pts',(5.03297999683575,-16.0652608298868,-28.0340873535912)) ;
#56537=CARTESIAN_POINT('Ctrl Pts',(4.97631377018983,-16.0735798722812,-27.9990714032078)) ;
#56538=CARTESIAN_POINT('Ctrl Pts',(4.91794125234338,-16.0816680200512,-27.9654843701936)) ;
#56539=CARTESIAN_POINT('Ctrl Pts',(4.85806847238345,-16.0894673869314,-27.933571512816)) ;
#56540=CARTESIAN_POINT('Ctrl Pts',(4.80887069611335,-16.0958761674671,-27.9073485510887)) ;
#56541=CARTESIAN_POINT('Ctrl Pts',(4.75866075408531,-16.1020900207686,-27.8822555005002)) ;
#56542=CARTESIAN_POINT('Ctrl Pts',(4.70757093348884,-16.108079933754,-27.8584093755501)) ;
#56543=CARTESIAN_POINT('Ctrl Pts',(4.64360347562769,-16.1155796568301,-27.8285526257106)) ;
#56544=CARTESIAN_POINT('Ctrl Pts',(4.57824661111033,-16.1227292229208,-27.8006472433746)) ;
#56545=CARTESIAN_POINT('Ctrl Pts',(4.51176172321611,-16.1294814162036,-27.7748729474675)) ;
#56546=CARTESIAN_POINT('Ctrl Pts',(4.44540828802764,-16.1362202591733,-27.7491496120273)) ;
#56547=CARTESIAN_POINT('Ctrl Pts',(4.37793172432457,-16.1425632136358,-27.725549194379)) ;
#56548=CARTESIAN_POINT('Ctrl Pts',(4.30961715334096,-16.148471764915,-27.7042057953237)) ;
#56549=CARTESIAN_POINT('Ctrl Pts',(4.25809740077133,-16.1529277264407,-27.6881095713047)) ;
#56550=CARTESIAN_POINT('Ctrl Pts',(4.20610160193261,-16.1571367885211,-27.6732961232077)) ;
#56551=CARTESIAN_POINT('Ctrl Pts',(4.15375919217086,-16.1610860188908,-27.6598050294532)) ;
#56552=CARTESIAN_POINT('Ctrl Pts',(4.08134971133679,-16.166549308068,-27.6411417103761)) ;
#56553=CARTESIAN_POINT('Ctrl Pts',(4.0082273929161,-16.171518536629,-27.6249987617427)) ;
#56554=CARTESIAN_POINT('Ctrl Pts',(3.93474530482786,-16.1759680067789,-27.6114406176889)) ;
#56555=CARTESIAN_POINT('Ctrl Pts',(3.86126321678012,-16.1804174769265,-27.5978824736426)) ;
#56556=CARTESIAN_POINT('Ctrl Pts',(3.78742199194697,-16.184347145014,-27.5869091829933)) ;
#56557=CARTESIAN_POINT('Ctrl Pts',(3.71358212375819,-16.1877442734702,-27.578525241158)) ;
#56558=CARTESIAN_POINT('',(3.8921733957507,-15.9108618782028,-29.0481967574568)) ;
#56559=CARTESIAN_POINT('Ctrl Pts',(3.89217339575145,-15.9108618782028,-29.0481967574567)) ;
#56560=CARTESIAN_POINT('Ctrl Pts',(3.80184066662191,-16.0510971574376,-28.3038250840197)) ;
#56561=CARTESIAN_POINT('Ctrl Pts',(3.71358212407717,-16.1877442737199,-27.5785252412372)) ;
#56562=CARTESIAN_POINT('',(2.4433270996089,-15.9108618782028,-29.2057682879055)) ;
#56563=CARTESIAN_POINT('Origin',(-2.92277791062251E-15,-15.9108618782028,
0.)) ;
#56564=CARTESIAN_POINT('',(2.30180707398557,-16.187744273641,-27.7320650306519)) ;
#56565=CARTESIAN_POINT('Ctrl Pts',(2.30180707378832,-16.1877442737199,-27.7320650307344)) ;
#56566=CARTESIAN_POINT('Ctrl Pts',(2.37152999322547,-16.0510971577989,-28.4593807420696)) ;
#56567=CARTESIAN_POINT('Ctrl Pts',(2.44332709960815,-15.9108618782028,-29.2057682879056)) ;
#56568=CARTESIAN_POINT('',(0.492460230914681,-15.9108618818334,-29.3036555873477)) ;
#56569=CARTESIAN_POINT('Ctrl Pts',(2.30180707408278,-16.1877442734702,-27.7320650305885)) ;
#56570=CARTESIAN_POINT('Ctrl Pts',(2.23149584064573,-16.184347145014,-27.7561263494924)) ;
#56571=CARTESIAN_POINT('Ctrl Pts',(2.16173991573636,-16.1804174769264,-27.7827167713124)) ;
#56572=CARTESIAN_POINT('Ctrl Pts',(2.09289039826652,-16.1759680067789,-27.8117544103006)) ;
#56573=CARTESIAN_POINT('Ctrl Pts',(2.02404088075871,-16.171518536629,-27.8407920493047)) ;
#56574=CARTESIAN_POINT('Ctrl Pts',(1.95609837828191,-16.166549308068,-27.87227672175)) ;
#56575=CARTESIAN_POINT('Ctrl Pts',(1.88939385278888,-16.1610860188908,-27.9060696007688)) ;
#56576=CARTESIAN_POINT('Ctrl Pts',(1.82547999051558,-16.155851292919,-27.9384487144716)) ;
#56577=CARTESIAN_POINT('Ctrl Pts',(1.76266128475666,-16.1501596984486,-27.9729674953457)) ;
#56578=CARTESIAN_POINT('Ctrl Pts',(1.7012090172553,-16.1440425621066,-28.009465757311)) ;
#56579=CARTESIAN_POINT('Ctrl Pts',(1.63962979052034,-16.1379127878754,-28.0460394240019)) ;
#56580=CARTESIAN_POINT('Ctrl Pts',(1.57942307856946,-16.1313557844549,-28.0846004726154)) ;
#56581=CARTESIAN_POINT('Ctrl Pts',(1.52083182384675,-16.1244124680045,-28.1249457608655)) ;
#56582=CARTESIAN_POINT('Ctrl Pts',(1.47668234604868,-16.1191805644222,-28.1553466016784)) ;
#56583=CARTESIAN_POINT('Ctrl Pts',(1.43344951505291,-16.1137295207044,-28.1867596072095)) ;
#56584=CARTESIAN_POINT('Ctrl Pts',(1.39122398593246,-16.1080799337539,-28.2190838414456)) ;
#56585=CARTESIAN_POINT('Ctrl Pts',(1.33681378242112,-16.1008000918637,-28.2607356146682)) ;
#56586=CARTESIAN_POINT('Ctrl Pts',(1.28406989208191,-16.0931892946345,-28.3039075854619)) ;
#56587=CARTESIAN_POINT('Ctrl Pts',(1.23317540655631,-16.0853002129681,-28.3483407890563)) ;
#56588=CARTESIAN_POINT('Ctrl Pts',(1.18186590786466,-16.0773468007023,-28.3931363180443)) ;
#56589=CARTESIAN_POINT('Ctrl Pts',(1.13243637431771,-16.0691106491233,-28.4392133119591)) ;
#56590=CARTESIAN_POINT('Ctrl Pts',(1.08503015713038,-16.0606518030572,-28.4862774263233)) ;
#56591=CARTESIAN_POINT('Ctrl Pts',(1.0462074930285,-16.0537245483848,-28.5248199300628)) ;
#56592=CARTESIAN_POINT('Ctrl Pts',(1.008740977047,-16.0466480826282,-28.5640237948626)) ;
#56593=CARTESIAN_POINT('Ctrl Pts',(0.972685940156643,-16.0394576303854,
-28.6037161955719)) ;
#56594=CARTESIAN_POINT('Ctrl Pts',(0.928587029583222,-16.0306629892537,
-28.652263965323)) ;
#56595=CARTESIAN_POINT('Ctrl Pts',(0.885469674162133,-16.0214720150687,
-28.7027885373364)) ;
#56596=CARTESIAN_POINT('Ctrl Pts',(0.843640804647336,-16.0119118209662,
-28.7551517869456)) ;
#56597=CARTESIAN_POINT('Ctrl Pts',(0.802154525420636,-16.002429927561,-28.8070861667102)) ;
#56598=CARTESIAN_POINT('Ctrl Pts',(0.761936143937485,-15.9925848997543,
-28.860828992985)) ;
#56599=CARTESIAN_POINT('Ctrl Pts',(0.723256922153069,-15.9824119250012,
-28.9162037651156)) ;
#56600=CARTESIAN_POINT('Ctrl Pts',(0.691497442736168,-15.9740589032139,
-28.9616719481493)) ;
#56601=CARTESIAN_POINT('Ctrl Pts',(0.660775258900229,-15.9654849570548,
-29.0082395567595)) ;
#56602=CARTESIAN_POINT('Ctrl Pts',(0.631223168391031,-15.9567135267634,
-29.055789510789)) ;
#56603=CARTESIAN_POINT('Ctrl Pts',(0.59420106811579,-15.9457249040904,-29.1153588724087)) ;
#56604=CARTESIAN_POINT('Ctrl Pts',(0.559010889735018,-15.9344245943247,
-29.1764794711086)) ;
#56605=CARTESIAN_POINT('Ctrl Pts',(0.525863355899135,-15.9228603613919,
-29.2389143704133)) ;
#56606=CARTESIAN_POINT('Ctrl Pts',(0.514486242769484,-15.9188912098108,
-29.2603436844656)) ;
#56607=CARTESIAN_POINT('Ctrl Pts',(0.503349410828287,-15.9148910209385,
-29.2819275511905)) ;
#56608=CARTESIAN_POINT('Ctrl Pts',(0.492460240898269,-15.9108618853164,
-29.3036555618719)) ;
#56609=CARTESIAN_POINT('Origin',(-2.92277791062251E-15,-15.9108618782028,
0.)) ;
#56610=CARTESIAN_POINT('Origin',(-1.76151330856832E-15,-9.58923182202279,
0.)) ;
#56611=CARTESIAN_POINT('',(1.01645642765342E-15,-2.97427793106409,-25.5228270052942)) ;
#56612=CARTESIAN_POINT('',(-1.30824146500192E-16,-9.58923182202279,-26.6311750163962)) ;
#56613=CARTESIAN_POINT('',(2.75950304786523,-2.97427793637248,-25.3732110958861)) ;
#56614=CARTESIAN_POINT('Origin',(-5.46365993374796E-16,-2.97427793741672,
0.)) ;
#56615=CARTESIAN_POINT('',(2.98582626636667,-16.2025431678319,-27.5780838874313)) ;
#56616=CARTESIAN_POINT('Ctrl Pts',(2.98582626636861,-16.2025431678318,-27.5780838874311)) ;
#56617=CARTESIAN_POINT('Ctrl Pts',(2.98552181236654,-16.1852171611512,-27.5751968800475)) ;
#56618=CARTESIAN_POINT('Ctrl Pts',(2.98521730416944,-16.167887657688,-27.5723092892116)) ;
#56619=CARTESIAN_POINT('Ctrl Pts',(2.9479315159664,-14.0459096732034,-27.2187269791237)) ;
#56620=CARTESIAN_POINT('Ctrl Pts',(2.90606163823145,-11.6569178621466,-26.8206408073361)) ;
#56621=CARTESIAN_POINT('Ctrl Pts',(2.86542833808716,-9.31987893565106,-26.4311762695601)) ;
#56622=CARTESIAN_POINT('Ctrl Pts',(2.83991825733066,-7.8564133077769,-26.1872986972926)) ;
#56623=CARTESIAN_POINT('Ctrl Pts',(2.7972066419062,-5.36133051494367,-25.7714235433997)) ;
#56624=CARTESIAN_POINT('Ctrl Pts',(2.7799975101858,-4.34397548535831,-25.6018305106833)) ;
#56625=CARTESIAN_POINT('Ctrl Pts',(2.76445921051843,-3.37503715194868,-25.4402158918861)) ;
#56626=CARTESIAN_POINT('Ctrl Pts',(2.76096814266673,-3.14436060309406,-25.4017174269074)) ;
#56627=CARTESIAN_POINT('Ctrl Pts',(2.75967493119254,-3.02949077923723,-25.3824979545439)) ;
#56628=CARTESIAN_POINT('Ctrl Pts',(2.75955256053887,-3.01786690009984,-25.3805521788679)) ;
#56629=CARTESIAN_POINT('Ctrl Pts',(2.75941568018604,-3.00170199339844,-25.3778426381123)) ;
#56630=CARTESIAN_POINT('Ctrl Pts',(2.75936689772594,-2.99510037673092,-25.3767353094954)) ;
#56631=CARTESIAN_POINT('Ctrl Pts',(2.75933336756686,-2.98631509723413,-25.375258288366)) ;
#56632=CARTESIAN_POINT('Ctrl Pts',(2.75931662463871,-2.98020409896568,-25.3742301638833)) ;
#56633=CARTESIAN_POINT('Ctrl Pts',(2.75939097519427,-2.97566130081685,-25.3734564362549)) ;
#56634=CARTESIAN_POINT('Ctrl Pts',(2.7594225130813,-2.97461345302792,-25.3732764024227)) ;
#56635=CARTESIAN_POINT('Ctrl Pts',(2.7594800824429,-2.97437347879031,-25.3732296962218)) ;
#56636=CARTESIAN_POINT('Ctrl Pts',(2.75949154295653,-2.97432570636421,-25.3732203982688)) ;
#56637=CARTESIAN_POINT('Ctrl Pts',(2.75950300346898,-2.97427793394,-25.3732111003045)) ;
#56638=CARTESIAN_POINT('',(3.01245352594498,-16.2025431678319,-27.5751879984371)) ;
#56639=CARTESIAN_POINT('Origin',(-0.0970287445296982,-21.5586464785792,
0.892164572691303)) ;
#56640=CARTESIAN_POINT('Ctrl Pts',(2.75950309456866,-2.97427793462802,-25.3732110905128)) ;
#56641=CARTESIAN_POINT('Ctrl Pts',(2.75951141791194,-2.97432669170439,-25.3732184027943)) ;
#56642=CARTESIAN_POINT('Ctrl Pts',(2.75951974125522,-2.97437544878077,-25.3732257150757)) ;
#56643=CARTESIAN_POINT('Ctrl Pts',(2.75988939774605,-2.97654084904765,-25.3735504682689)) ;
#56644=CARTESIAN_POINT('Ctrl Pts',(2.76054593631754,-3.00035443887309,-25.3774925990095)) ;
#56645=CARTESIAN_POINT('Ctrl Pts',(2.76768271304796,-3.25662181914454,-25.4199076371643)) ;
#56646=CARTESIAN_POINT('Ctrl Pts',(2.80101276140845,-4.98861101441761,-25.708191593734)) ;
#56647=CARTESIAN_POINT('Ctrl Pts',(2.85987603015594,-8.03277302580515,-26.2148517658915)) ;
#56648=CARTESIAN_POINT('Ctrl Pts',(2.96783636940418,-13.8113507317231,-27.177029718695)) ;
#56649=CARTESIAN_POINT('Ctrl Pts',(3.01245352594286,-16.2025431678266,-27.5751879984364)) ;
#56650=CARTESIAN_POINT('',(8.14947771659192,-2.97427793708563,-24.1867879500451)) ;
#56651=CARTESIAN_POINT('Origin',(-5.46365993374796E-16,-2.97427793741672,
0.)) ;
#56652=CARTESIAN_POINT('',(8.84449214097205,-16.2025431678319,-26.2914592246876)) ;
#56653=CARTESIAN_POINT('Ctrl Pts',(8.8444921409701,-16.2025431678318,-26.2914592246882)) ;
#56654=CARTESIAN_POINT('Ctrl Pts',(8.84368137315711,-16.1872403113959,-26.2890267531794)) ;
#56655=CARTESIAN_POINT('Ctrl Pts',(8.84287052996823,-16.1719359305085,-26.2865940375341)) ;
#56656=CARTESIAN_POINT('Ctrl Pts',(8.73054679496111,-14.051850633938,-25.9495945481204)) ;
#56657=CARTESIAN_POINT('Ctrl Pts',(8.60409127671067,-11.6630949900927,-25.5698538329076)) ;
#56658=CARTESIAN_POINT('Ctrl Pts',(8.48066779311721,-9.32575037806886,-25.1981813327223)) ;
#56659=CARTESIAN_POINT('Ctrl Pts',(8.40325559611451,-7.86092828798006,-24.9652738433449)) ;
#56660=CARTESIAN_POINT('Ctrl Pts',(8.27203747702655,-5.36388181438923,-24.5679912751739)) ;
#56661=CARTESIAN_POINT('Ctrl Pts',(8.21874191386539,-4.34594047228758,-24.4059695641208)) ;
#56662=CARTESIAN_POINT('Ctrl Pts',(8.1687574984097,-3.37573518131635,-24.2512722575224)) ;
#56663=CARTESIAN_POINT('Ctrl Pts',(8.15704769885815,-3.14458998495216,-24.2143496755378)) ;
#56664=CARTESIAN_POINT('Ctrl Pts',(8.15164435056689,-3.02954097345787,-24.1958288135939)) ;
#56665=CARTESIAN_POINT('Ctrl Pts',(8.15110606607062,-3.01790731507202,-24.1939532713909)) ;
#56666=CARTESIAN_POINT('Ctrl Pts',(8.15038939015159,-3.00173216030816,-24.1913348682466)) ;
#56667=CARTESIAN_POINT('Ctrl Pts',(8.15010371261148,-2.9951315069744,-24.1902640829975)) ;
#56668=CARTESIAN_POINT('Ctrl Pts',(8.14975280318563,-2.98633297379899,-24.1888266765532)) ;
#56669=CARTESIAN_POINT('Ctrl Pts',(8.14951604066345,-2.98023844423496,-24.187828896103)) ;
#56670=CARTESIAN_POINT('Ctrl Pts',(8.14942093279696,-2.97566575016659,-24.1870524576967)) ;
#56671=CARTESIAN_POINT('Ctrl Pts',(8.14941248312575,-2.9745868821094,-24.1868645533682)) ;
#56672=CARTESIAN_POINT('Ctrl Pts',(8.14945763957049,-2.97437302162435,-24.1868115263829)) ;
#56673=CARTESIAN_POINT('Ctrl Pts',(8.14946767807719,-2.97432547935386,-24.1867997382152)) ;
#56674=CARTESIAN_POINT('Ctrl Pts',(8.14947771658388,-2.97427793708336,-24.1867879500474)) ;
#56675=CARTESIAN_POINT('',(8.86987433948411,-16.2025431678319,-26.2829069662563)) ;
#56676=CARTESIAN_POINT('Origin',(-0.286549277334569,-21.5586464785792,0.850447948841961)) ;
#56677=CARTESIAN_POINT('Ctrl Pts',(8.14947771672321,-2.97427793642345,-24.1867879498838)) ;
#56678=CARTESIAN_POINT('Ctrl Pts',(8.14949133329423,-2.97432588904375,-24.1867918402822)) ;
#56679=CARTESIAN_POINT('Ctrl Pts',(8.14950494986526,-2.97437384166406,-24.1867957306806)) ;
#56680=CARTESIAN_POINT('Ctrl Pts',(8.14976489484414,-2.97528927351905,-24.1868699997108)) ;
#56681=CARTESIAN_POINT('Ctrl Pts',(8.15057001316975,-2.98748334132594,-24.1887547193953)) ;
#56682=CARTESIAN_POINT('Ctrl Pts',(8.1554153766091,-3.05983249654133,-24.1999139580347)) ;
#56683=CARTESIAN_POINT('Ctrl Pts',(8.17321910187599,-3.37814096324511,-24.250194325778)) ;
#56684=CARTESIAN_POINT('Ctrl Pts',(8.25150376159725,-4.77686335530337,-24.4711209579954)) ;
#56685=CARTESIAN_POINT('Ctrl Pts',(8.51332551264261,-9.61051733687626,-25.2375264361977)) ;
#56686=CARTESIAN_POINT('Ctrl Pts',(8.64483231029231,-12.0381142500592,-25.6224325826173)) ;
#56687=CARTESIAN_POINT('Ctrl Pts',(8.76313990580416,-14.2266207751237,-25.9695132217007)) ;
#56688=CARTESIAN_POINT('Ctrl Pts',(8.86987433948527,-16.2025431678314,-26.2829069662558)) ;
#56689=CARTESIAN_POINT('',(13.15839190919,-2.97427793741672,-21.8694174764822)) ;
#56690=CARTESIAN_POINT('Origin',(-5.46365993374796E-16,-2.97427793741672,
0.)) ;
#56691=CARTESIAN_POINT('',(14.2895993930077,-16.2025431678318,-23.7754751494576)) ;
#56692=CARTESIAN_POINT('Ctrl Pts',(14.2895993930102,-16.2025431678314,-23.7754751494561)) ;
#56693=CARTESIAN_POINT('Ctrl Pts',(14.288479812531,-16.1895116831815,-23.7736005749326)) ;
#56694=CARTESIAN_POINT('Ctrl Pts',(14.287359600215,-16.176472803045,-23.7717249344438)) ;
#56695=CARTESIAN_POINT('Ctrl Pts',(14.1053987293089,-14.0585050844697,-23.4670553231882)) ;
#56696=CARTESIAN_POINT('Ctrl Pts',(13.9002890366153,-11.6700134946164,-23.1234150926258)) ;
#56697=CARTESIAN_POINT('Ctrl Pts',(13.6998225204247,-9.33232681203563,-22.7869156532154)) ;
#56698=CARTESIAN_POINT('Ctrl Pts',(13.5740212516687,-7.86598567644115,-22.5758763480535)) ;
#56699=CARTESIAN_POINT('Ctrl Pts',(13.3602778229174,-5.36674011566134,-22.2157738106669)) ;
#56700=CARTESIAN_POINT('Ctrl Pts',(13.2733417726211,-4.34814220965037,-22.0689027346577)) ;
#56701=CARTESIAN_POINT('Ctrl Pts',(13.1911487884526,-3.37651773132946,-21.9283631278092)) ;
#56702=CARTESIAN_POINT('Ctrl Pts',(13.1717308858037,-3.1448473048907,-21.8947451711901)) ;
#56703=CARTESIAN_POINT('Ctrl Pts',(13.16245590613,-3.02959726689373,-21.8777895079707)) ;
#56704=CARTESIAN_POINT('Ctrl Pts',(13.1615260986429,-3.01795254848073,-21.876071921995)) ;
#56705=CARTESIAN_POINT('Ctrl Pts',(13.1602624142991,-3.00176697334617,-21.8736672944438)) ;
#56706=CARTESIAN_POINT('Ctrl Pts',(13.1597534264871,-2.99516934250607,-21.8726834277241)) ;
#56707=CARTESIAN_POINT('Ctrl Pts',(13.1591004799476,-2.98635587386225,-21.8713528885411)) ;
#56708=CARTESIAN_POINT('Ctrl Pts',(13.1586561623224,-2.98028108276681,-21.8704323482376)) ;
#56709=CARTESIAN_POINT('Ctrl Pts',(13.1584155616641,-2.97606013386572,-21.8697517396796)) ;
#56710=CARTESIAN_POINT('Ctrl Pts',(13.1582567494634,-2.97516487197257,-21.8696722323615)) ;
#56711=CARTESIAN_POINT('Ctrl Pts',(13.1583774170714,-2.97437303709565,-21.8694447921021)) ;
#56712=CARTESIAN_POINT('Ctrl Pts',(13.1583846631407,-2.97432548753967,-21.8694311343495)) ;
#56713=CARTESIAN_POINT('Ctrl Pts',(13.1583919092032,-2.97427793798588,-21.8694174765856)) ;
#56714=CARTESIAN_POINT('',(14.3125496870687,-16.2025431678319,-23.7616664156855)) ;
#56715=CARTESIAN_POINT('Origin',(-0.46267108440793,-21.5586464785791,0.768965324109772)) ;
#56716=CARTESIAN_POINT('Ctrl Pts',(13.1583919092032,-2.97427793798589,-21.8694174765856)) ;
#56717=CARTESIAN_POINT('Ctrl Pts',(13.1584053694963,-2.97432607419128,-21.8694187904502)) ;
#56718=CARTESIAN_POINT('Ctrl Pts',(13.1584188297894,-2.97437421039667,-21.8694201043147)) ;
#56719=CARTESIAN_POINT('Ctrl Pts',(13.1586774926046,-2.97529923084781,-21.8694453524952)) ;
#56720=CARTESIAN_POINT('Ctrl Pts',(13.1597050744733,-2.98568920246521,-21.8708587537663)) ;
#56721=CARTESIAN_POINT('Ctrl Pts',(13.1706903685768,-3.09726433021604,-21.8860667553059)) ;
#56722=CARTESIAN_POINT('Ctrl Pts',(13.2279185476989,-3.74807332618725,-21.9788942538091)) ;
#56723=CARTESIAN_POINT('Ctrl Pts',(13.4698566107615,-6.49929376644458,-22.3713043467384)) ;
#56724=CARTESIAN_POINT('Ctrl Pts',(14.2415308001386,-15.3848269920527,-23.6444991319492)) ;
#56725=CARTESIAN_POINT('Ctrl Pts',(14.3125496870575,-16.2025431677232,-23.761666415671)) ;
#56726=CARTESIAN_POINT('',(17.5520343204297,-2.97427793976807,-18.5294573485322)) ;
#56727=CARTESIAN_POINT('Origin',(-5.46365993374796E-16,-2.97427793741672,
0.)) ;
#56728=CARTESIAN_POINT('',(19.0665408591787,-16.2025431678318,-20.1477762807808)) ;
#56729=CARTESIAN_POINT('Ctrl Pts',(19.0665408591778,-16.2025431678318,-20.1477762807817)) ;
#56730=CARTESIAN_POINT('Ctrl Pts',(19.0652008544727,-16.190873531221,-20.1463523789925)) ;
#56731=CARTESIAN_POINT('Ctrl Pts',(19.0638614007779,-16.1792086722493,-20.1449290578845)) ;
#56732=CARTESIAN_POINT('Ctrl Pts',(18.8208071414155,-14.0625257526841,-19.886655527428)) ;
#56733=CARTESIAN_POINT('Ctrl Pts',(18.5466384510028,-11.6741934639051,-19.5951615140958)) ;
#56734=CARTESIAN_POINT('Ctrl Pts',(18.2784972693573,-9.33630026618093,-19.3095987195106)) ;
#56735=CARTESIAN_POINT('Ctrl Pts',(18.1101644799581,-7.86904147552841,-19.1304250740684)) ;
#56736=CARTESIAN_POINT('Ctrl Pts',(17.8238542141176,-5.36846742573192,-18.8245280395046)) ;
#56737=CARTESIAN_POINT('Ctrl Pts',(17.7073320841991,-4.34947290227263,-18.6997311217121)) ;
#56738=CARTESIAN_POINT('Ctrl Pts',(17.5967504477281,-3.37699090265648,-18.580041634387)) ;
#56739=CARTESIAN_POINT('Ctrl Pts',(17.5705234637249,-3.14500297466746,-18.5513449311427)) ;
#56740=CARTESIAN_POINT('Ctrl Pts',(17.5578067836975,-3.02963134974649,-18.5367643290789)) ;
#56741=CARTESIAN_POINT('Ctrl Pts',(17.5565287224273,-3.01797986529181,-18.5352859406662)) ;
#56742=CARTESIAN_POINT('Ctrl Pts',(17.5547769763625,-3.00178832029484,-18.5332084551072)) ;
#56743=CARTESIAN_POINT('Ctrl Pts',(17.554068640032,-2.99519322179253,-18.5323573519155)) ;
#56744=CARTESIAN_POINT('Ctrl Pts',(17.5531439282108,-2.98637087130639,-18.5311971856173)) ;
#56745=CARTESIAN_POINT('Ctrl Pts',(17.5525133237871,-2.98030797966027,-18.530395278245)) ;
#56746=CARTESIAN_POINT('Ctrl Pts',(17.5521302611564,-2.97607197580719,-18.5297805121099)) ;
#56747=CARTESIAN_POINT('Ctrl Pts',(17.5519437475032,-2.97516258420107,-18.5297473096757)) ;
#56748=CARTESIAN_POINT('Ctrl Pts',(17.5520246374274,-2.97437252356484,-18.5294883496527)) ;
#56749=CARTESIAN_POINT('Ctrl Pts',(17.5520294791351,-2.97432523401781,-18.5294728494395)) ;
#56750=CARTESIAN_POINT('Ctrl Pts',(17.5520343208427,-2.97427794447078,-18.5294573492263)) ;
#56751=CARTESIAN_POINT('',(19.0859861185406,-16.2025431678319,-20.1293567527132)) ;
#56752=CARTESIAN_POINT('Origin',(-0.617158905796344,-21.5586464785791,0.651526735465783)) ;
#56753=CARTESIAN_POINT('Ctrl Pts',(17.5520343208427,-2.97427794447078,-18.5294573492263)) ;
#56754=CARTESIAN_POINT('Ctrl Pts',(17.5520469269176,-2.97432632302893,-18.5294565733482)) ;
#56755=CARTESIAN_POINT('Ctrl Pts',(17.5520595329925,-2.97437470158707,-18.5294557974702)) ;
#56756=CARTESIAN_POINT('Ctrl Pts',(17.5526934119907,-2.9768073503034,-18.529416783517)) ;
#56757=CARTESIAN_POINT('Ctrl Pts',(17.5528034283629,-2.979337953762,-18.529896605461)) ;
#56758=CARTESIAN_POINT('Ctrl Pts',(17.557220828315,-3.01332285628473,-18.5335555575299)) ;
#56759=CARTESIAN_POINT('Ctrl Pts',(17.5725224009764,-3.14289186108968,-18.5489642157879)) ;
#56760=CARTESIAN_POINT('Ctrl Pts',(17.6982486755249,-4.20803765545581,-18.6756937040713)) ;
#56761=CARTESIAN_POINT('Ctrl Pts',(18.2934730507535,-9.35158026128418,-19.2989393579036)) ;
#56762=CARTESIAN_POINT('Ctrl Pts',(18.5832196153222,-11.8548215072816,-19.6021969277266)) ;
#56763=CARTESIAN_POINT('Ctrl Pts',(18.8490355543646,-14.153188423186,-19.8808400851401)) ;
#56764=CARTESIAN_POINT('Ctrl Pts',(19.0859861185426,-16.2025431678314,-20.1293567527112)) ;
#56765=CARTESIAN_POINT('',(21.1249631147115,-2.97427793656,-14.323080387656)) ;
#56766=CARTESIAN_POINT('Origin',(-5.46365993374796E-16,-2.97427793741672,
0.)) ;
#56767=CARTESIAN_POINT('',(22.9519520657137,-16.2025431678319,-15.5779897858583)) ;
#56768=CARTESIAN_POINT('Ctrl Pts',(22.9519520657139,-16.2025431678317,-15.5779897858579)) ;
#56769=CARTESIAN_POINT('Ctrl Pts',(22.9502335499534,-16.1901238028483,-15.5768164009677)) ;
#56770=CARTESIAN_POINT('Ctrl Pts',(22.948514579347,-16.1777011355868,-15.5756427009756)) ;
#56771=CARTESIAN_POINT('Ctrl Pts',(22.6555236061391,-14.0603095790929,-15.3755899261384)) ;
#56772=CARTESIAN_POINT('Ctrl Pts',(22.3250901464934,-11.6718894994608,-15.1498406568082)) ;
#56773=CARTESIAN_POINT('Ctrl Pts',(22.0018462798773,-9.33411011491888,-14.9286071448455)) ;
#56774=CARTESIAN_POINT('Ctrl Pts',(21.7990020106076,-7.86735711472142,-14.7898567783282)) ;
#56775=CARTESIAN_POINT('Ctrl Pts',(21.4537280604868,-5.36751530138658,-14.5527288153069)) ;
#56776=CARTESIAN_POINT('Ctrl Pts',(21.3131328026182,-4.3487393845648,-14.4559189764242)) ;
#56777=CARTESIAN_POINT('Ctrl Pts',(21.1794721847679,-3.37673005063584,-14.3628442350099)) ;
#56778=CARTESIAN_POINT('Ctrl Pts',(21.147713535865,-3.14491714238785,-14.340473172792)) ;
#56779=CARTESIAN_POINT('Ctrl Pts',(21.132168877764,-3.02961254565857,-14.3289737413805)) ;
#56780=CARTESIAN_POINT('Ctrl Pts',(21.1306033981186,-3.0179648009679,-14.3278050250569)) ;
#56781=CARTESIAN_POINT('Ctrl Pts',(21.1284464644897,-3.00177655927346,-14.3261529979161)) ;
#56782=CARTESIAN_POINT('Ctrl Pts',(21.127571548738,-2.99518006149376,-14.3254739090271)) ;
#56783=CARTESIAN_POINT('Ctrl Pts',(21.1264197256475,-2.98636260828327,-14.3245401250765)) ;
#56784=CARTESIAN_POINT('Ctrl Pts',(21.1256306236549,-2.98029306927367,-14.3238918025835)) ;
#56785=CARTESIAN_POINT('Ctrl Pts',(21.125125531062,-2.97606537332734,-14.3233745101534)) ;
#56786=CARTESIAN_POINT('Ctrl Pts',(21.1249429849765,-2.9751639433579,-14.3233746085866)) ;
#56787=CARTESIAN_POINT('Ctrl Pts',(21.1249609586001,-2.97437281839512,-14.3231118962033)) ;
#56788=CARTESIAN_POINT('Ctrl Pts',(21.1249620364161,-2.97432537736582,-14.3230961422498)) ;
#56789=CARTESIAN_POINT('Ctrl Pts',(21.1249631142322,-2.97427793633651,-14.3230803882963)) ;
#56790=CARTESIAN_POINT('',(22.9669830516602,-16.2025431678319,-15.5558207401564)) ;
#56791=CARTESIAN_POINT('Origin',(-0.742789062672596,-21.5586464785791,0.503623480791383)) ;
#56792=CARTESIAN_POINT('Ctrl Pts',(21.1249631142997,-2.97427793336231,-14.3230803873086)) ;
#56793=CARTESIAN_POINT('Ctrl Pts',(21.1249757103847,-2.97432613941351,-14.3230762021838)) ;
#56794=CARTESIAN_POINT('Ctrl Pts',(21.1249883064698,-2.97437434546471,-14.323072017059)) ;
#56795=CARTESIAN_POINT('Ctrl Pts',(21.1252387195819,-2.97533269302076,-14.3229888158006)) ;
#56796=CARTESIAN_POINT('Ctrl Pts',(21.1267571463958,-2.98566592142204,-14.3238344593653)) ;
#56797=CARTESIAN_POINT('Ctrl Pts',(21.1441719217104,-3.10455043621784,-14.3336445177555)) ;
#56798=CARTESIAN_POINT('Ctrl Pts',(21.2437508331783,-3.81759438301236,-14.3996676280851)) ;
#56799=CARTESIAN_POINT('Ctrl Pts',(21.6375804487957,-6.63755433615676,-14.6607579010562)) ;
#56800=CARTESIAN_POINT('Ctrl Pts',(22.8541348968827,-15.3906124573063,-15.479844027184)) ;
#56801=CARTESIAN_POINT('Ctrl Pts',(22.9669830516443,-16.2025431677233,-15.5558207401474)) ;
#56802=CARTESIAN_POINT('',(23.7101121129195,-2.97427793806634,-9.44697210723373)) ;
#56803=CARTESIAN_POINT('Origin',(-5.46365993374796E-16,-2.97427793741672,
0.)) ;
#56804=CARTESIAN_POINT('',(25.7641555029171,-16.2025431678319,-10.2797938022428)) ;
#56805=CARTESIAN_POINT('Ctrl Pts',(25.7641555029177,-16.2025431678319,-10.2797938022413)) ;
#56806=CARTESIAN_POINT('Ctrl Pts',(25.7618588421009,-16.1877688223624,-10.2788700351982)) ;
#56807=CARTESIAN_POINT('Ctrl Pts',(25.7595617877488,-16.1729919326657,-10.2779461041504)) ;
#56808=CARTESIAN_POINT('Ctrl Pts',(25.4300733391726,-14.0533996634013,-10.1454170231319)) ;
#56809=CARTESIAN_POINT('Ctrl Pts',(25.0587933387861,-11.6647055250785,-9.99596160917884)) ;
#56810=CARTESIAN_POINT('Ctrl Pts',(24.6956035468433,-9.32728125403024,-9.84940980079011)) ;
#56811=CARTESIAN_POINT('Ctrl Pts',(24.4679197096846,-7.86210552892475,-9.75760726356454)) ;
#56812=CARTESIAN_POINT('Ctrl Pts',(24.0800976015277,-5.36454711209344,-9.60038948428051)) ;
#56813=CARTESIAN_POINT('Ctrl Pts',(23.9220842020473,-4.34645292073481,-9.53610920565715)) ;
#56814=CARTESIAN_POINT('Ctrl Pts',(23.7717692171093,-3.37591727900287,-9.4740358356347)) ;
#56815=CARTESIAN_POINT('Ctrl Pts',(23.7360285131927,-3.14464984801546,-9.45904965421893)) ;
#56816=CARTESIAN_POINT('Ctrl Pts',(23.7184073683066,-3.02955407834925,-9.45117461641968)) ;
#56817=CARTESIAN_POINT('Ctrl Pts',(23.7166290266303,-3.0179178504392,-9.45037050831506)) ;
#56818=CARTESIAN_POINT('Ctrl Pts',(23.7141690200475,-3.00174015894501,-9.44922145101896)) ;
#56819=CARTESIAN_POINT('Ctrl Pts',(23.7131680376703,-2.99514001169015,-9.44874601721026)) ;
#56820=CARTESIAN_POINT('Ctrl Pts',(23.711844782819,-2.98633794415978,-9.44808267590362)) ;
#56821=CARTESIAN_POINT('Ctrl Pts',(23.7109317473047,-2.98024818549774,-9.44761755137845)) ;
#56822=CARTESIAN_POINT('Ctrl Pts',(23.7102769572539,-2.97566596594098,-9.44718670224653)) ;
#56823=CARTESIAN_POINT('Ctrl Pts',(23.71012721905,-2.97457957456447,-9.44707073648006)) ;
#56824=CARTESIAN_POINT('Ctrl Pts',(23.7101168677483,-2.97437287975886,-9.44700315107804)) ;
#56825=CARTESIAN_POINT('Ctrl Pts',(23.7101144904349,-2.97432540956222,-9.44698762919633)) ;
#56826=CARTESIAN_POINT('Ctrl Pts',(23.7101121131215,-2.97427793936558,-9.44697210731461)) ;
#56827=CARTESIAN_POINT('',(25.7740693832514,-16.2025431678319,-10.2549118388444)) ;
#56828=CARTESIAN_POINT('Origin',(-0.833687228529012,-21.5586464785791,0.332171351892473)) ;
#56829=CARTESIAN_POINT('Ctrl Pts',(23.7101121131215,-2.97427793936557,-9.44697210731464)) ;
#56830=CARTESIAN_POINT('Ctrl Pts',(23.7101245644293,-2.97432536598929,-9.44696232568401)) ;
#56831=CARTESIAN_POINT('Ctrl Pts',(23.7101370157242,-2.97437279261535,-9.44695254404822)) ;
#56832=CARTESIAN_POINT('Ctrl Pts',(23.710141161062,-2.974388582092,-9.4469492875036)) ;
#56833=CARTESIAN_POINT('Ctrl Pts',(23.7103474475408,-2.97517432156201,-9.44678723047638)) ;
#56834=CARTESIAN_POINT('Ctrl Pts',(23.7104505646161,-2.976087915043,-9.4469419856964)) ;
#56835=CARTESIAN_POINT('Ctrl Pts',(23.7105996529263,-2.97697407685809,-9.44696894400583)) ;
#56836=CARTESIAN_POINT('Ctrl Pts',(23.7106181044487,-2.97708375034319,-9.44697228043005)) ;
#56837=CARTESIAN_POINT('Ctrl Pts',(23.7106365725645,-2.97719377294972,-9.44697573324589)) ;
#56838=CARTESIAN_POINT('Ctrl Pts',(23.7106549402653,-2.97730340753796,-9.44697926243895)) ;
#56839=CARTESIAN_POINT('Ctrl Pts',(23.7122516294942,-2.98683385276827,-9.44728605230987)) ;
#56840=CARTESIAN_POINT('Ctrl Pts',(23.717151258952,-3.01773210335417,-9.44897572128477)) ;
#56841=CARTESIAN_POINT('Ctrl Pts',(23.7194721219178,-3.03238727965577,-9.44978480081932)) ;
#56842=CARTESIAN_POINT('Ctrl Pts',(23.7514418208435,-3.23426114336774,-9.46092980571913)) ;
#56843=CARTESIAN_POINT('Ctrl Pts',(23.8661184658587,-3.96778714974358,-9.50516074375344)) ;
#56844=CARTESIAN_POINT('Ctrl Pts',(24.0044670674295,-4.85383245444821,-9.55902094396787)) ;
#56845=CARTESIAN_POINT('Ctrl Pts',(24.1732653666677,-5.93489101798971,-9.62473545130367)) ;
#56846=CARTESIAN_POINT('Ctrl Pts',(24.3773019647013,-7.24299428982599,-9.70478555188628)) ;
#56847=CARTESIAN_POINT('Ctrl Pts',(24.5093215665893,-8.08953550083095,-9.75664790617047)) ;
#56848=CARTESIAN_POINT('Ctrl Pts',(24.5789706735296,-8.53614220537689,-9.7840087420468)) ;
#56849=CARTESIAN_POINT('Ctrl Pts',(24.6285750786978,-8.85428404324401,-9.80352538383069)) ;
#56850=CARTESIAN_POINT('Ctrl Pts',(24.6423854231622,-8.94284901749011,-9.8089550279813)) ;
#56851=CARTESIAN_POINT('Ctrl Pts',(24.9521304391092,-10.9292266513597,-9.93073368588121)) ;
#56852=CARTESIAN_POINT('Ctrl Pts',(25.3061682654494,-13.2004672662886,-10.0702956267967)) ;
#56853=CARTESIAN_POINT('Ctrl Pts',(25.6253338879632,-15.2482357967354,-10.1962203605316)) ;
#56854=CARTESIAN_POINT('Ctrl Pts',(25.6758923865101,-15.5726194238176,-10.2161678893959)) ;
#56855=CARTESIAN_POINT('Ctrl Pts',(25.7255757904938,-15.8913954202363,-10.2357733156429)) ;
#56856=CARTESIAN_POINT('Ctrl Pts',(25.7740693832509,-16.2025431678319,-10.2549118388455)) ;
#56857=CARTESIAN_POINT('',(25.1866026330875,-2.97427793670427,-4.12913383088527)) ;
#56858=CARTESIAN_POINT('Origin',(-5.46365993374796E-16,-2.97427793741672,
0.)) ;
#56859=CARTESIAN_POINT('',(27.3716556636073,-16.2025431678319,-4.50092608560063)) ;
#56860=CARTESIAN_POINT('Ctrl Pts',(27.3716556636072,-16.202543167832,-4.50092608560152)) ;
#56861=CARTESIAN_POINT('Ctrl Pts',(27.3688793881231,-16.1857433178334,-4.50046163223941)) ;
#56862=CARTESIAN_POINT('Ctrl Pts',(27.3661036374749,-16.1689466370182,-4.49999725972657)) ;
#56863=CARTESIAN_POINT('Ctrl Pts',(27.0155166994629,-14.0474667172661,-4.44134451708904)) ;
#56864=CARTESIAN_POINT('Ctrl Pts',(26.620749614247,-11.6585368364515,-4.37519069607536)) ;
#56865=CARTESIAN_POINT('Ctrl Pts',(26.2345972311031,-9.32141776663148,-4.31014806193477)) ;
#56866=CARTESIAN_POINT('Ctrl Pts',(25.9927255660653,-7.85759660531187,-4.26947436137525)) ;
#56867=CARTESIAN_POINT('Ctrl Pts',(25.5804974344147,-5.36199912641347,-4.19935656741213)) ;
#56868=CARTESIAN_POINT('Ctrl Pts',(25.4124567326006,-4.34449041885194,-4.17056329497325)) ;
#56869=CARTESIAN_POINT('Ctrl Pts',(25.2525211642905,-3.37522003995815,-4.14228952629787)) ;
#56870=CARTESIAN_POINT('Ctrl Pts',(25.2144717382874,-3.14442068985397,-4.13535037988208)) ;
#56871=CARTESIAN_POINT('Ctrl Pts',(25.1955991210527,-3.02950392542895,-4.13145320038075)) ;
#56872=CARTESIAN_POINT('Ctrl Pts',(25.1936911107792,-3.01787749425057,-4.13105048247988)) ;
#56873=CARTESIAN_POINT('Ctrl Pts',(25.1910432510912,-3.00170978382865,-4.13045741104492)) ;
#56874=CARTESIAN_POINT('Ctrl Pts',(25.1899632323033,-2.99510816665471,-4.13020818293691)) ;
#56875=CARTESIAN_POINT('Ctrl Pts',(25.1885305246722,-2.98631952130879,-4.1298452372347)) ;
#56876=CARTESIAN_POINT('Ctrl Pts',(25.1875359969717,-2.98021222223683,-4.12958648357871)) ;
#56877=CARTESIAN_POINT('Ctrl Pts',(25.1868092668585,-2.97566275848799,-4.12930762945622)) ;
#56878=CARTESIAN_POINT('Ctrl Pts',(25.1866429189275,-2.97460667468206,-4.12922855990008)) ;
#56879=CARTESIAN_POINT('Ctrl Pts',(25.186614318913,-2.97437337060343,-4.12916138794003)) ;
#56880=CARTESIAN_POINT('Ctrl Pts',(25.1866084692863,-2.9743256524054,-4.12914764911027)) ;
#56881=CARTESIAN_POINT('Ctrl Pts',(25.186602619648,-2.97427793420933,-4.1291339102786)) ;
#56882=CARTESIAN_POINT('',(27.3759888763025,-16.2025431678319,-4.47449465746573)) ;
#56883=CARTESIAN_POINT('Origin',(-0.885603106156239,-21.5586464785792,0.145187259760998)) ;
#56884=CARTESIAN_POINT('Ctrl Pts',(25.1866026463618,-2.97427793634941,-4.12913374954807)) ;
#56885=CARTESIAN_POINT('Ctrl Pts',(25.1866118621959,-2.97432675308219,-4.12912809313557)) ;
#56886=CARTESIAN_POINT('Ctrl Pts',(25.18662107803,-2.97437556981498,-4.12912243672306)) ;
#56887=CARTESIAN_POINT('Ctrl Pts',(25.1870320563893,-2.97655254268123,-4.12887019008873)) ;
#56888=CARTESIAN_POINT('Ctrl Pts',(25.1905243613001,-2.9974640474975,-4.12922534632092)) ;
#56889=CARTESIAN_POINT('Ctrl Pts',(25.2327027816895,-3.25009986877477,-4.13359396024206)) ;
#56890=CARTESIAN_POINT('Ctrl Pts',(25.5150428575483,-4.95577965796636,-4.17790529570596)) ;
#56891=CARTESIAN_POINT('Ctrl Pts',(26.0181996523211,-7.99518172117798,-4.25658117072354)) ;
#56892=CARTESIAN_POINT('Ctrl Pts',(26.9837924566198,-13.8318142714633,-4.41151055827675)) ;
#56893=CARTESIAN_POINT('Ctrl Pts',(27.3759888763017,-16.2025431678263,-4.47449465746506)) ;
#56894=CARTESIAN_POINT('',(25.4853955792416,-2.97427793781143,1.38177804637892)) ;
#56895=CARTESIAN_POINT('Origin',(-5.46365993374796E-16,-2.97427793741672,
0.)) ;
#56896=CARTESIAN_POINT('',(27.6992876268763,-16.2025431678319,1.48839993237836)) ;
#56897=CARTESIAN_POINT('Ctrl Pts',(27.6992876268763,-16.2025431678319,1.48839993237756)) ;
#56898=CARTESIAN_POINT('Ctrl Pts',(27.6963977131487,-16.1852729916106,1.4882527002794)) ;
#56899=CARTESIAN_POINT('Ctrl Pts',(27.6935087726697,-16.1680086338848,1.48810552502117)) ;
#56900=CARTESIAN_POINT('Ctrl Pts',(27.3384366271439,-14.0460917074,1.47001749405664)) ;
#56901=CARTESIAN_POINT('Ctrl Pts',(26.9386687046014,-11.6571071306621,1.44976102534322)) ;
#56902=CARTESIAN_POINT('Ctrl Pts',(26.5475739404773,-9.32005883264334,1.43027240288789)) ;
#56903=CARTESIAN_POINT('Ctrl Pts',(26.3026659929641,-7.85655164084812,1.41800263993642)) ;
#56904=CARTESIAN_POINT('Ctrl Pts',(25.8850783273247,-5.36140867819081,1.39786817314536)) ;
#56905=CARTESIAN_POINT('Ctrl Pts',(25.7147993278214,-4.34403568258248,1.38986570156608)) ;
#56906=CARTESIAN_POINT('Ctrl Pts',(25.552574008522,-3.37505853191685,1.38309950148959)) ;
#56907=CARTESIAN_POINT('Ctrl Pts',(25.5139405992457,-3.14436762797809,1.38169771258376)) ;
#56908=CARTESIAN_POINT('Ctrl Pts',(25.4946783799856,-3.02949230886718,1.38144689609332)) ;
#56909=CARTESIAN_POINT('Ctrl Pts',(25.492728784212,-3.01786813878313,1.38143004544643)) ;
#56910=CARTESIAN_POINT('Ctrl Pts',(25.4900157460364,-3.00170287001805,1.3814400553632)) ;
#56911=CARTESIAN_POINT('Ctrl Pts',(25.4889073884696,-2.99510118203702,1.38145129303794)) ;
#56912=CARTESIAN_POINT('Ctrl Pts',(25.4874306594782,-2.98631555202997,1.38149777525331)) ;
#56913=CARTESIAN_POINT('Ctrl Pts',(25.4864031753873,-2.98020478534521,1.38153671577505)) ;
#56914=CARTESIAN_POINT('Ctrl Pts',(25.4856345023826,-2.9756613593825,1.38165284654919)) ;
#56915=CARTESIAN_POINT('Ctrl Pts',(25.4854562944026,-2.97461265172528,1.38169410945281)) ;
#56916=CARTESIAN_POINT('Ctrl Pts',(25.4854129102212,-2.97437347068115,1.38175405510917)) ;
#56917=CARTESIAN_POINT('Ctrl Pts',(25.4854042460737,-2.97432570444335,1.38176602670364)) ;
#56918=CARTESIAN_POINT('Ctrl Pts',(25.4853955819149,-2.97427793820744,1.38177799829751)) ;
#56919=CARTESIAN_POINT('',(27.6978375557248,-16.2025431678319,1.51514492105661)) ;
#56920=CARTESIAN_POINT('Origin',(-0.896109166816728,-21.5586464785791,-0.0485856272728391)) ;
#56921=CARTESIAN_POINT('Ctrl Pts',(25.4853955766927,-2.97427793899426,1.38177809705115)) ;
#56922=CARTESIAN_POINT('Ctrl Pts',(25.4854033747212,-2.97432678020061,1.38178542694295)) ;
#56923=CARTESIAN_POINT('Ctrl Pts',(25.4854111727497,-2.97437562140695,1.38179275683474)) ;
#56924=CARTESIAN_POINT('Ctrl Pts',(25.4861536393221,-2.97902589460994,1.38249065113243)) ;
#56925=CARTESIAN_POINT('Ctrl Pts',(25.4869504275186,-2.98368443800432,1.38221223700358)) ;
#56926=CARTESIAN_POINT('Ctrl Pts',(25.4972660985915,-3.04564095439207,1.38369682324666)) ;
#56927=CARTESIAN_POINT('Ctrl Pts',(25.5376066632687,-3.28698876069824,1.38659344204126)) ;
#56928=CARTESIAN_POINT('Ctrl Pts',(25.751738340196,-4.56809667345973,1.40200013610528)) ;
#56929=CARTESIAN_POINT('Ctrl Pts',(26.5774290539577,-9.50442793797728,1.45022142307887)) ;
#56930=CARTESIAN_POINT('Ctrl Pts',(26.9887013828208,-11.9632015308957,1.47427793563209)) ;
#56931=CARTESIAN_POINT('Ctrl Pts',(27.3622462521282,-14.1963338960462,1.49585140007546)) ;
#56932=CARTESIAN_POINT('Ctrl Pts',(27.6978375557247,-16.2025431678314,1.51514492105782)) ;
#56933=CARTESIAN_POINT('',(24.5925339350698,-2.97427793675404,6.82802848946651)) ;
#56934=CARTESIAN_POINT('Origin',(-5.46365993374796E-16,-2.97427793741672,
0.)) ;
#56935=CARTESIAN_POINT('',(22.5497250682996,-2.97427793653627,11.9551076002299)) ;
#56936=CARTESIAN_POINT('Origin',(-5.46365993374796E-16,-2.97427793741672,
0.)) ;
#56937=CARTESIAN_POINT('',(24.5142296821797,-16.2025431678319,12.9814641887756)) ;
#56938=CARTESIAN_POINT('Ctrl Pts',(24.5142296821792,-16.2025431678315,12.9814641887765)) ;
#56939=CARTESIAN_POINT('Ctrl Pts',(24.5122080448287,-16.1889101644085,12.9804008194301)) ;
#56940=CARTESIAN_POINT('Ctrl Pts',(24.5101851232767,-16.1752685151775,12.9793367797034)) ;
#56941=CARTESIAN_POINT('Ctrl Pts',(24.1960275789333,-14.05673727217,12.8140933509909)) ;
#56942=CARTESIAN_POINT('Ctrl Pts',(23.8417764769763,-11.6681756019773,12.627883389876)) ;
#56943=CARTESIAN_POINT('Ctrl Pts',(23.4949308862975,-9.33057976211665,12.4459358417275)) ;
#56944=CARTESIAN_POINT('Ctrl Pts',(23.2774501530511,-7.86464213425622,12.3317760355887)) ;
#56945=CARTESIAN_POINT('Ctrl Pts',(22.9063904996838,-5.36598072794395,12.1378872505747)) ;
#56946=CARTESIAN_POINT('Ctrl Pts',(22.7550540299499,-4.34755722511546,12.0590438033061)) ;
#56947=CARTESIAN_POINT('Ctrl Pts',(22.6103266209746,-3.37630976879788,11.9846094037368)) ;
#56948=CARTESIAN_POINT('Ctrl Pts',(22.5757274743488,-3.14477890327531,11.9670507629476)) ;
#56949=CARTESIAN_POINT('Ctrl Pts',(22.5583025731781,-3.0295822976008,11.9587113092107)) ;
#56950=CARTESIAN_POINT('Ctrl Pts',(22.5565376094953,-3.01794053203936,11.9578760760157)) ;
#56951=CARTESIAN_POINT('Ctrl Pts',(22.5540684899263,-3.0017576190999,11.9567446344546)) ;
#56952=CARTESIAN_POINT('Ctrl Pts',(22.5530583529934,-2.99515899568192,11.9562895998487)) ;
#56953=CARTESIAN_POINT('Ctrl Pts',(22.5516950135079,-2.98634952387366,11.9557099462857)) ;
#56954=CARTESIAN_POINT('Ctrl Pts',(22.5507509201939,-2.98026930995719,11.9553157774299)) ;
#56955=CARTESIAN_POINT('Ctrl Pts',(22.5500592500757,-2.9760549690666,11.955112918444)) ;
#56956=CARTESIAN_POINT('Ctrl Pts',(22.549968984505,-2.97516557803826,11.9549650384074)) ;
#56957=CARTESIAN_POINT('Ctrl Pts',(22.549751253269,-2.97437322618191,11.955092295629)) ;
#56958=CARTESIAN_POINT('Ctrl Pts',(22.5497381608798,-2.97432558130056,11.9550999477284)) ;
#56959=CARTESIAN_POINT('Ctrl Pts',(22.5497250684906,-2.97427793641922,11.9551075998279)) ;
#56960=CARTESIAN_POINT('',(24.5016837039789,-16.2025431678319,13.0051284140257)) ;
#56961=CARTESIAN_POINT('Origin',(-0.792886077760343,-21.5586464785791,-0.420361594016718)) ;
#56962=CARTESIAN_POINT('Ctrl Pts',(22.5497250680389,-2.97427793477537,11.9551076000919)) ;
#56963=CARTESIAN_POINT('Ctrl Pts',(22.5497269705711,-2.97432600972966,11.9551212081462)) ;
#56964=CARTESIAN_POINT('Ctrl Pts',(22.5497288731033,-2.97437408468395,11.9551348162005)) ;
#56965=CARTESIAN_POINT('Ctrl Pts',(22.5497645661837,-2.97527601066585,11.9553901145756)) ;
#56966=CARTESIAN_POINT('Ctrl Pts',(22.5512523836686,-2.98580920545014,11.9563515605873)) ;
#56967=CARTESIAN_POINT('Ctrl Pts',(22.5664879099537,-3.09354746925243,11.9661527335954)) ;
#56968=CARTESIAN_POINT('Ctrl Pts',(22.6569327161989,-3.70814168940487,12.0153986349189)) ;
#56969=CARTESIAN_POINT('Ctrl Pts',(23.0555175961015,-6.41664653573796,12.2324312219111)) ;
#56970=CARTESIAN_POINT('Ctrl Pts',(24.3803519333028,-15.3815014745936,12.9402943899549)) ;
#56971=CARTESIAN_POINT('Ctrl Pts',(24.5016837039635,-16.202543167723,13.0051284140159)) ;
#56972=CARTESIAN_POINT('',(19.452530284046,-2.97427793908284,16.5231281529567)) ;
#56973=CARTESIAN_POINT('Origin',(-5.46365993374796E-16,-2.97427793741672,
0.)) ;
#56974=CARTESIAN_POINT('',(21.1504695437725,-16.2025431678318,17.9477995161824)) ;
#56975=CARTESIAN_POINT('Ctrl Pts',(21.1504695437711,-16.2025431678318,17.947799516184)) ;
#56976=CARTESIAN_POINT('Ctrl Pts',(21.148968900584,-16.190824464327,17.9465332633256)) ;
#56977=CARTESIAN_POINT('Ctrl Pts',(21.1474684155399,-16.1791070126478,17.945267148275)) ;
#56978=CARTESIAN_POINT('Ctrl Pts',(20.8764086676346,-14.0623748796458,17.7165466823383)) ;
#56979=CARTESIAN_POINT('Ctrl Pts',(20.5704981887938,-11.674036593923,17.4585606095428)) ;
#56980=CARTESIAN_POINT('Ctrl Pts',(20.2708383068535,-9.33615114017493,17.2062735872375)) ;
#56981=CARTESIAN_POINT('Ctrl Pts',(20.082818488219,-7.86892678806865,17.0478916631225)) ;
#56982=CARTESIAN_POINT('Ctrl Pts',(19.761875934007,-5.3684025943473,16.778567618261)) ;
#56983=CARTESIAN_POINT('Ctrl Pts',(19.6309555628547,-4.349422954631,16.6689743597236)) ;
#56984=CARTESIAN_POINT('Ctrl Pts',(19.5054589643214,-3.37697313855551,16.5650382345451)) ;
#56985=CARTESIAN_POINT('Ctrl Pts',(19.4753859819799,-3.1449971286427,16.5404046002665)) ;
#56986=CARTESIAN_POINT('Ctrl Pts',(19.4601388940641,-3.02963007022637,16.528496426528)) ;
#56987=CARTESIAN_POINT('Ctrl Pts',(19.4585935139585,-3.0179788392836,16.527300304782)) ;
#56988=CARTESIAN_POINT('Ctrl Pts',(19.4564242764873,-3.00178759363925,16.5256636322884)) ;
#56989=CARTESIAN_POINT('Ctrl Pts',(19.4555360690703,-2.99519247023055,16.5250024107204)) ;
#56990=CARTESIAN_POINT('Ctrl Pts',(19.4543275962744,-2.98637053452838,16.5241419079155)) ;
#56991=CARTESIAN_POINT('Ctrl Pts',(19.4534925911232,-2.98030667154562,16.5235555486211)) ;
#56992=CARTESIAN_POINT('Ctrl Pts',(19.4528580640734,-2.97607130659674,16.5232064063515)) ;
#56993=CARTESIAN_POINT('Ctrl Pts',(19.4528144225956,-2.97516258009942,16.523022595322)) ;
#56994=CARTESIAN_POINT('Ctrl Pts',(19.4525606694781,-2.97437254331412,16.5231168652152)) ;
#56995=CARTESIAN_POINT('Ctrl Pts',(19.4525454769748,-2.97432524286461,16.5231225092668)) ;
#56996=CARTESIAN_POINT('Ctrl Pts',(19.4525302844714,-2.9742779424151,16.5231281533183)) ;
#56997=CARTESIAN_POINT('',(21.1331297746478,-16.2025431678318,17.9682134705435)) ;
#56998=CARTESIAN_POINT('Origin',(-0.683983524963516,-21.5586464785791,-0.580980842721111)) ;
#56999=CARTESIAN_POINT('Ctrl Pts',(19.4525302844714,-2.9742779424151,16.5231281533183)) ;
#57000=CARTESIAN_POINT('Ctrl Pts',(19.4525255622681,-2.97432450011737,16.5231457624397)) ;
#57001=CARTESIAN_POINT('Ctrl Pts',(19.4525208400648,-2.97437105781963,16.5231633715611)) ;
#57002=CARTESIAN_POINT('Ctrl Pts',(19.4524565452229,-2.9750049610918,16.5234031273721)) ;
#57003=CARTESIAN_POINT('Ctrl Pts',(19.4526315145313,-2.9757780922962,16.5233972335742)) ;
#57004=CARTESIAN_POINT('Ctrl Pts',(19.4535415058967,-2.98456713021951,16.5246006215295)) ;
#57005=CARTESIAN_POINT('Ctrl Pts',(19.4570077244971,-3.01292535222663,16.5278593349976)) ;
#57006=CARTESIAN_POINT('Ctrl Pts',(19.48457703876,-3.23724786189985,16.5534596918303)) ;
#57007=CARTESIAN_POINT('Ctrl Pts',(19.5819054214816,-4.00652715930706,16.6379749412941)) ;
#57008=CARTESIAN_POINT('Ctrl Pts',(19.8512530910474,-6.12954829805385,16.8703386896818)) ;
#57009=CARTESIAN_POINT('Ctrl Pts',(20.03438465427,-7.56992759765112,17.0275276590373)) ;
#57010=CARTESIAN_POINT('Ctrl Pts',(20.2755054134284,-9.46557599994605,17.2342758017243)) ;
#57011=CARTESIAN_POINT('Ctrl Pts',(20.353310307754,-10.076892225596,17.3008930715163)) ;
#57012=CARTESIAN_POINT('Ctrl Pts',(20.6176064477318,-12.1539254231473,17.5273016927547)) ;
#57013=CARTESIAN_POINT('Ctrl Pts',(20.8875535671149,-14.2741505136447,17.7582360672092)) ;
#57014=CARTESIAN_POINT('Ctrl Pts',(21.133129774648,-16.2025431678318,17.9682134705432)) ;
#57015=CARTESIAN_POINT('',(15.445756803441,-2.97427793744554,20.3185455967131)) ;
#57016=CARTESIAN_POINT('Origin',(-5.46365993374796E-16,-2.97427793741672,
0.)) ;
#57017=CARTESIAN_POINT('',(16.7977369565509,-16.2025431678319,22.0749156857653)) ;
#57018=CARTESIAN_POINT('Ctrl Pts',(16.797736956552,-16.2025431678319,22.0749156857645)) ;
#57019=CARTESIAN_POINT('Ctrl Pts',(16.7965330820174,-16.1907211336376,22.0733426945111)) ;
#57020=CARTESIAN_POINT('Ctrl Pts',(16.7953292286977,-16.1788993343194,22.0717697365644)) ;
#57021=CARTESIAN_POINT('Ctrl Pts',(16.5797648994147,-14.0620696072946,21.7901138157647)) ;
#57022=CARTESIAN_POINT('Ctrl Pts',(16.3364645751062,-11.6737192459128,21.4723960063734)) ;
#57023=CARTESIAN_POINT('Ctrl Pts',(16.0980463971873,-9.3358494693627,21.1615914035746)) ;
#57024=CARTESIAN_POINT('Ctrl Pts',(15.9484768950245,-7.86869477940399,20.9665029328927)) ;
#57025=CARTESIAN_POINT('Ctrl Pts',(15.6929447704673,-5.36827143841294,20.6344957971552)) ;
#57026=CARTESIAN_POINT('Ctrl Pts',(15.5886476126233,-4.34932190866538,20.4993247717653)) ;
#57027=CARTESIAN_POINT('Ctrl Pts',(15.4884348833676,-3.3769371970094,20.3708492157565)) ;
#57028=CARTESIAN_POINT('Ctrl Pts',(15.4643629708558,-3.14498529561199,20.3403298909891)) ;
#57029=CARTESIAN_POINT('Ctrl Pts',(15.4520332309067,-3.0296274890746,20.3254236572053)) ;
#57030=CARTESIAN_POINT('Ctrl Pts',(15.4507811640484,-3.0179767598727,20.3239233549216)) ;
#57031=CARTESIAN_POINT('Ctrl Pts',(15.44901451832,-3.00178590816239,20.3218586775132)) ;
#57032=CARTESIAN_POINT('Ctrl Pts',(15.4482891915348,-2.99519054213983,20.3210219470156)) ;
#57033=CARTESIAN_POINT('Ctrl Pts',(15.4472940203856,-2.98636924589745,20.3199218611091)) ;
#57034=CARTESIAN_POINT('Ctrl Pts',(15.4466045047521,-2.98030468072635,20.3191696239606)) ;
#57035=CARTESIAN_POINT('Ctrl Pts',(15.4460599816571,-2.97607045456207,20.3186923930545)) ;
#57036=CARTESIAN_POINT('Ctrl Pts',(15.4460558392151,-2.97516281294533,20.3185045129636)) ;
#57037=CARTESIAN_POINT('Ctrl Pts',(15.4457887885214,-2.97437258257387,20.3185412020118)) ;
#57038=CARTESIAN_POINT('Ctrl Pts',(15.4457727963274,-2.97432526003727,20.3185433991146)) ;
#57039=CARTESIAN_POINT('Ctrl Pts',(15.4457568041244,-2.97427793750316,20.3185455962057)) ;
#57040=CARTESIAN_POINT('',(16.7764141848447,-16.2025431678319,22.09112483541)) ;
#57041=CARTESIAN_POINT('Origin',(-0.54309866273249,-21.5586464785792,-0.714434072933713)) ;
#57042=CARTESIAN_POINT('Ctrl Pts',(15.4457568041244,-2.97427793750316,20.3185455962057)) ;
#57043=CARTESIAN_POINT('Ctrl Pts',(15.4457539152905,-2.97432629596546,20.3185579701203)) ;
#57044=CARTESIAN_POINT('Ctrl Pts',(15.4457510264566,-2.97437465442775,20.3185703440349)) ;
#57045=CARTESIAN_POINT('Ctrl Pts',(15.445605609725,-2.97680889943481,20.3191932161949)) ;
#57046=CARTESIAN_POINT('Ctrl Pts',(15.4460664305379,-2.97934517843716,20.3193767133853)) ;
#57047=CARTESIAN_POINT('Ctrl Pts',(15.4489469102806,-3.01314182309645,20.3243001217788)) ;
#57048=CARTESIAN_POINT('Ctrl Pts',(15.461523981169,-3.14117529750347,20.341686154419)) ;
#57049=CARTESIAN_POINT('Ctrl Pts',(15.5658036103066,-4.20201593204481,20.4856872188289)) ;
#57050=CARTESIAN_POINT('Ctrl Pts',(16.0849048047097,-9.34914178729712,21.1743789821445)) ;
#57051=CARTESIAN_POINT('Ctrl Pts',(16.3373613204017,-11.853076400732,21.5094631536216)) ;
#57052=CARTESIAN_POINT('Ctrl Pts',(16.5694362224003,-14.1525004571554,21.816998218385)) ;
#57053=CARTESIAN_POINT('Ctrl Pts',(16.7764141848436,-16.2025431678314,22.0911248354107)) ;
#57054=CARTESIAN_POINT('',(10.7167569009779,-2.97427793741672,23.1638904314851)) ;
#57055=CARTESIAN_POINT('Origin',(-5.46365993374796E-16,-2.97427793741672,
0.)) ;
#57056=CARTESIAN_POINT('',(11.6595608585889,-16.2025431678318,25.169833332384)) ;
#57057=CARTESIAN_POINT('Ctrl Pts',(11.6595608585918,-16.2025431678318,25.1698333323826)) ;
#57058=CARTESIAN_POINT('Ctrl Pts',(11.6585530880691,-16.1883190110886,25.1676735901348)) ;
#57059=CARTESIAN_POINT('Ctrl Pts',(11.6575457015777,-16.1741003377176,25.1655146825256)) ;
#57060=CARTESIAN_POINT('Ctrl Pts',(11.5074098720457,-14.0550300026374,24.8437636611566)) ;
#57061=CARTESIAN_POINT('Ctrl Pts',(11.338077613478,-11.6664005728183,24.4811293179889)) ;
#57062=CARTESIAN_POINT('Ctrl Pts',(11.1720722581951,-9.32889248177215,24.1263935292874)) ;
#57063=CARTESIAN_POINT('Ctrl Pts',(11.068051484594,-7.863344578113,23.9039571658016)) ;
#57064=CARTESIAN_POINT('Ctrl Pts',(10.8900298857863,-5.3652473681901,23.525133601664)) ;
#57065=CARTESIAN_POINT('Ctrl Pts',(10.8172778670904,-4.34699231213758,23.3708075548896)) ;
#57066=CARTESIAN_POINT('Ctrl Pts',(10.7471329839059,-3.37610897168059,23.2240208229558)) ;
#57067=CARTESIAN_POINT('Ctrl Pts',(10.7302245680935,-3.1447128703852,23.1891243965598)) ;
#57068=CARTESIAN_POINT('Ctrl Pts',(10.7214034046739,-3.02956783168136,23.1719480498592)) ;
#57069=CARTESIAN_POINT('Ctrl Pts',(10.7205040011658,-3.01792892294217,23.1702154461329)) ;
#57070=CARTESIAN_POINT('Ctrl Pts',(10.7192232634546,-3.00174867959296,23.1678208698723)) ;
#57071=CARTESIAN_POINT('Ctrl Pts',(10.7186943984944,-2.99514921220744,23.166847191043)) ;
#57072=CARTESIAN_POINT('Ctrl Pts',(10.717960123488,-2.98634352741144,23.1655612451486)) ;
#57073=CARTESIAN_POINT('Ctrl Pts',(10.7174466464294,-2.9802583336125,23.1646753895135)) ;
#57074=CARTESIAN_POINT('Ctrl Pts',(10.7169801109564,-2.97566543965881,23.1640433166783)) ;
#57075=CARTESIAN_POINT('Ctrl Pts',(10.7168553875118,-2.97457165285031,23.1638990908922)) ;
#57076=CARTESIAN_POINT('Ctrl Pts',(10.7167886800643,-2.9743727123176,23.1638932257357)) ;
#57077=CARTESIAN_POINT('Ctrl Pts',(10.7167727904227,-2.97432532489865,23.1638918286617)) ;
#57078=CARTESIAN_POINT('Ctrl Pts',(10.7167569007811,-2.9742779374797,23.1638904315878)) ;
#57079=CARTESIAN_POINT('',(11.6352521133992,-16.2025431678318,25.1810797554983)) ;
#57080=CARTESIAN_POINT('Origin',(-0.376819110642892,-21.5586464785792,-0.814481159932352)) ;
#57081=CARTESIAN_POINT('Ctrl Pts',(10.7167569006248,-2.97427793701361,23.1638904315741)) ;
#57082=CARTESIAN_POINT('Ctrl Pts',(10.7167499840165,-2.97432596370162,23.1639024979641)) ;
#57083=CARTESIAN_POINT('Ctrl Pts',(10.7167430674081,-2.97437399038964,23.1639145643541)) ;
#57084=CARTESIAN_POINT('Ctrl Pts',(10.7166124790537,-2.97528075362364,23.1641423826623)) ;
#57085=CARTESIAN_POINT('Ctrl Pts',(10.717256330779,-2.98644231985364,23.1659050928526)) ;
#57086=CARTESIAN_POINT('Ctrl Pts',(10.7232995481034,-3.09146650890056,23.1824981979959)) ;
#57087=CARTESIAN_POINT('Ctrl Pts',(10.7638322197368,-3.68205504702985,23.272777034556)) ;
#57088=CARTESIAN_POINT('Ctrl Pts',(10.947704709346,-6.36122868516908,23.6823230437698)) ;
#57089=CARTESIAN_POINT('Ctrl Pts',(11.5777447190413,-15.3793271372196,25.0557078381133)) ;
#57090=CARTESIAN_POINT('Ctrl Pts',(11.6352521133898,-16.2025431677228,25.1810797554824)) ;
#57091=CARTESIAN_POINT('',(5.48671463442036,-2.97427793619619,24.9261040060569)) ;
#57092=CARTESIAN_POINT('Origin',(-5.46365993374796E-16,-2.97427793741672,
0.)) ;
#57093=CARTESIAN_POINT('',(-5.12525029468365E-8,-2.97427793862301,25.5228270065607)) ;
#57094=CARTESIAN_POINT('Origin',(-5.46365993374796E-16,-2.97427793741672,
0.)) ;
#57095=CARTESIAN_POINT('',(0.0133921350610688,-16.2025431678318,27.7392445831865)) ;
#57096=CARTESIAN_POINT('Ctrl Pts',(0.0133921350608421,-16.2025431678318,
27.7392445831865)) ;
#57097=CARTESIAN_POINT('Ctrl Pts',(0.0133827205563863,-16.1853207396188,
27.7363589370385)) ;
#57098=CARTESIAN_POINT('Ctrl Pts',(0.0133732997516836,-16.1680999693416,
27.7334735686804)) ;
#57099=CARTESIAN_POINT('Ctrl Pts',(0.0122116115369291,-14.0462236600739,
27.3779497062717)) ;
#57100=CARTESIAN_POINT('Ctrl Pts',(0.0107953830161923,-11.6572443672643,
26.97767230005)) ;
#57101=CARTESIAN_POINT('Ctrl Pts',(0.00908199061164238,-9.32018928178254,
26.5860948800897)) ;
#57102=CARTESIAN_POINT('Ctrl Pts',(0.00807469792554111,-7.85665194902709,
26.3408767894379)) ;
#57103=CARTESIAN_POINT('Ctrl Pts',(0.00557187555144761,-5.36146535513246,
25.9228041835425)) ;
#57104=CARTESIAN_POINT('Ctrl Pts',(0.0043438896367992,-4.34407933277878,
25.7523394851314)) ;
#57105=CARTESIAN_POINT('Ctrl Pts',(0.00231744706143683,-3.37507403506501,
25.5899810524667)) ;
#57106=CARTESIAN_POINT('Ctrl Pts',(0.0016255918363982,-3.14437272175176,
25.551326666984)) ;
#57107=CARTESIAN_POINT('Ctrl Pts',(0.000833185359603188,-3.02949341768707,
25.5320784508113)) ;
#57108=CARTESIAN_POINT('Ctrl Pts',(0.000744461577372581,-3.01786903750215,
25.5301307668094)) ;
#57109=CARTESIAN_POINT('Ctrl Pts',(0.000587585115252702,-3.00170356762241,
25.527422215767)) ;
#57110=CARTESIAN_POINT('Ctrl Pts',(0.000516359911024086,-2.99510191775345,
25.5263160984832)) ;
#57111=CARTESIAN_POINT('Ctrl Pts',(0.000389995404236694,-2.9863159414149,
25.52484399371)) ;
#57112=CARTESIAN_POINT('Ctrl Pts',(0.000295494913282459,-2.98020577737517,
25.5238202256846)) ;
#57113=CARTESIAN_POINT('Ctrl Pts',(0.000137918756552516,-2.97566162983232,
25.5230588462965)) ;
#57114=CARTESIAN_POINT('Ctrl Pts',(8.70400132779651E-5,-2.97461210268643,
25.5228829962964)) ;
#57115=CARTESIAN_POINT('Ctrl Pts',(2.48813437772203E-5,-2.97437346419653,
25.5228430120269)) ;
#57116=CARTESIAN_POINT('Ctrl Pts',(1.24407261809522E-5,-2.97432570239241,
25.5228350094584)) ;
#57117=CARTESIAN_POINT('Ctrl Pts',(1.08584684169698E-10,-2.9742779405883,
25.52282700689)) ;
#57118=CARTESIAN_POINT('',(-0.0133921350595798,-16.2025431678318,27.7392445831865)) ;
#57119=CARTESIAN_POINT('Origin',(0.,-21.5586464785791,-0.89742531835827)) ;
#57120=CARTESIAN_POINT('Ctrl Pts',(-1.04424683376919E-7,-2.97427794148292,
25.5228270070399)) ;
#57121=CARTESIAN_POINT('Ctrl Pts',(-6.9948999599768E-6,-2.97432678358026,
25.5228351906136)) ;
#57122=CARTESIAN_POINT('Ctrl Pts',(-1.38853752365767E-5,-2.9743756256776,
25.5228433741872)) ;
#57123=CARTESIAN_POINT('Ctrl Pts',(-0.000671733076929959,-2.97903868013909,
25.5236246766248)) ;
#57124=CARTESIAN_POINT('Ctrl Pts',(-0.000349894671792411,-2.98370976889989,
25.5244073252225)) ;
#57125=CARTESIAN_POINT('Ctrl Pts',(-0.00127721170310683,-3.0459772111706,
25.5348403374966)) ;
#57126=CARTESIAN_POINT('Ctrl Pts',(-0.00198813524755864,-3.28900867603421,
25.5755606587986)) ;
#57127=CARTESIAN_POINT('Ctrl Pts',(-0.00577579228133441,-4.57301664693183,
25.7906983042822)) ;
#57128=CARTESIAN_POINT('Ctrl Pts',(-0.00922328543825932,-9.50679819544934,
26.6173615102215)) ;
#57129=CARTESIAN_POINT('Ctrl Pts',(-0.0109779254506447,-11.9648785601619,
27.0292169145927)) ;
#57130=CARTESIAN_POINT('Ctrl Pts',(-0.012295824988902,-14.1970078152399,
27.4032138392471)) ;
#57131=CARTESIAN_POINT('Ctrl Pts',(-0.0133921350608563,-16.2025431678313,
27.7392445831864)) ;
#57132=CARTESIAN_POINT('',(-5.48671360278494,-2.97427793932974,24.926104233655)) ;
#57133=CARTESIAN_POINT('Origin',(-5.46365993374796E-16,-2.97427793741672,
0.)) ;
#57134=CARTESIAN_POINT('',(-5.9500385847868,-16.2025431678319,27.0935953729783)) ;
#57135=CARTESIAN_POINT('Ctrl Pts',(-5.95003858478663,-16.2025431678314,
27.0935953729783)) ;
#57136=CARTESIAN_POINT('Ctrl Pts',(-5.93287872287226,-15.7189595649501,
27.0144076436256)) ;
#57137=CARTESIAN_POINT('Ctrl Pts',(-5.91524350319025,-15.221824220667,26.9329995753094)) ;
#57138=CARTESIAN_POINT('Ctrl Pts',(-5.84492153936488,-13.2386274094556,
26.6082360433019)) ;
#57139=CARTESIAN_POINT('Ctrl Pts',(-5.79005095651472,-11.6894126530758,
26.3545265310519)) ;
#57140=CARTESIAN_POINT('Ctrl Pts',(-5.73090391748631,-10.0154554223458,
26.0803571843471)) ;
#57141=CARTESIAN_POINT('Ctrl Pts',(-5.72326138326653,-9.79907595711066,
26.0449167916378)) ;
#57142=CARTESIAN_POINT('Ctrl Pts',(-5.71470558583829,-9.55673624964,26.0052236145411)) ;
#57143=CARTESIAN_POINT('Ctrl Pts',(-5.71390057186316,-9.53393434274454,
26.0014888551816)) ;
#57144=CARTESIAN_POINT('Ctrl Pts',(-5.70139110462718,-9.17956028534485,
25.943445032905)) ;
#57145=CARTESIAN_POINT('Ctrl Pts',(-5.6614752520146,-8.04994044340242,25.7584305573157)) ;
#57146=CARTESIAN_POINT('Ctrl Pts',(-5.58189130805735,-5.78271924794518,
25.3869777597823)) ;
#57147=CARTESIAN_POINT('Ctrl Pts',(-5.54324092011608,-4.67645412098992,
25.2056915431067)) ;
#57148=CARTESIAN_POINT('Ctrl Pts',(-5.51469385636707,-3.84233733089944,
25.0688719125288)) ;
#57149=CARTESIAN_POINT('Ctrl Pts',(-5.51222100231848,-3.76985007295875,
25.0569801203902)) ;
#57150=CARTESIAN_POINT('Ctrl Pts',(-5.50324787511175,-3.50579051812552,
25.013652489226)) ;
#57151=CARTESIAN_POINT('Ctrl Pts',(-5.49776736515089,-3.34217420314569,
24.9867883866358)) ;
#57152=CARTESIAN_POINT('Ctrl Pts',(-5.49131928366058,-3.14397212208866,
24.9542036358068)) ;
#57153=CARTESIAN_POINT('Ctrl Pts',(-5.48943105222872,-3.0840140701563,24.9443327026901)) ;
#57154=CARTESIAN_POINT('Ctrl Pts',(-5.48781659384092,-3.02914875405639,
24.9352752309949)) ;
#57155=CARTESIAN_POINT('Ctrl Pts',(-5.48742247974211,-3.01553314732883,
24.933026052041)) ;
#57156=CARTESIAN_POINT('Ctrl Pts',(-5.48690349060606,-2.99517799299728,
24.9296481052891)) ;
#57157=CARTESIAN_POINT('Ctrl Pts',(-5.48675589318455,-2.99005670072696,
24.9288019711253)) ;
#57158=CARTESIAN_POINT('Ctrl Pts',(-5.48665234506065,-2.97915009782824,
24.9269535988966)) ;
#57159=CARTESIAN_POINT('Ctrl Pts',(-5.48668297585237,-2.97671402055501,
24.9265289164305)) ;
#57160=CARTESIAN_POINT('Ctrl Pts',(-5.48671360402347,-2.97427794328177,
24.9261042337966)) ;
#57161=CARTESIAN_POINT('',(-5.97619665355032,-16.2025431678318,27.0878375466411)) ;
#57162=CARTESIAN_POINT('Origin',(0.192919915744003,-21.5586464785792,-0.876444013123368)) ;
#57163=CARTESIAN_POINT('Ctrl Pts',(-5.48671360403907,-2.97427794326962,
24.9261042338674)) ;
#57164=CARTESIAN_POINT('Ctrl Pts',(-5.4867544422091,-2.97466563176781,24.9261617575856)) ;
#57165=CARTESIAN_POINT('Ctrl Pts',(-5.48679114024367,-2.9751949691749,24.9262444942833)) ;
#57166=CARTESIAN_POINT('Ctrl Pts',(-5.48794225379729,-2.98815252649866,
24.9282141483353)) ;
#57167=CARTESIAN_POINT('Ctrl Pts',(-5.48820355368734,-3.0009526412213,24.9303526539106)) ;
#57168=CARTESIAN_POINT('Ctrl Pts',(-5.4917702937201,-3.08233977560006,24.9435305502341)) ;
#57169=CARTESIAN_POINT('Ctrl Pts',(-5.49591359064664,-3.18658700036627,
24.9605034752394)) ;
#57170=CARTESIAN_POINT('Ctrl Pts',(-5.50101843278592,-3.31684853906785,
24.9817278336455)) ;
#57171=CARTESIAN_POINT('Ctrl Pts',(-5.50255804554906,-3.35653277590054,
24.9881972734115)) ;
#57172=CARTESIAN_POINT('Ctrl Pts',(-5.50440219560687,-3.40414624973906,
24.9959600406285)) ;
#57173=CARTESIAN_POINT('Ctrl Pts',(-5.5047590081922,-3.41339294985133,24.9974678889237)) ;
#57174=CARTESIAN_POINT('Ctrl Pts',(-5.54132990195816,-4.36100762295681,
25.1519933426862)) ;
#57175=CARTESIAN_POINT('Ctrl Pts',(-5.63758587198842,-6.96806954423069,
25.5780803406581)) ;
#57176=CARTESIAN_POINT('Ctrl Pts',(-5.72482181396427,-9.33961765357979,
25.9657474153764)) ;
#57177=CARTESIAN_POINT('Ctrl Pts',(-5.74458877632446,-9.87816198815649,
26.0537904891407)) ;
#57178=CARTESIAN_POINT('Ctrl Pts',(-5.75033083195084,-10.0345661355023,
26.0793596823434)) ;
#57179=CARTESIAN_POINT('Ctrl Pts',(-5.75109550216058,-10.0553952782751,
26.0827648693305)) ;
#57180=CARTESIAN_POINT('Ctrl Pts',(-5.82459880453683,-12.0576523218942,
26.4100981603903)) ;
#57181=CARTESIAN_POINT('Ctrl Pts',(-5.90433700445679,-14.2366140340412,
26.7663749738318)) ;
#57182=CARTESIAN_POINT('Ctrl Pts',(-5.97619665355194,-16.2025431678313,
27.0878375466407)) ;
#57183=CARTESIAN_POINT('',(-10.716756900978,-2.97427793741671,23.1638904314851)) ;
#57184=CARTESIAN_POINT('Origin',(-5.46365993374796E-16,-2.97427793741672,
0.)) ;
#57185=CARTESIAN_POINT('',(-11.6352521133983,-16.2025431678318,25.1810797554987)) ;
#57186=CARTESIAN_POINT('Ctrl Pts',(-11.6352521133968,-16.2025431678318,
25.1810797554994)) ;
#57187=CARTESIAN_POINT('Ctrl Pts',(-11.6342584581205,-16.1883190325504,
25.1789134868053)) ;
#57188=CARTESIAN_POINT('Ctrl Pts',(-11.6332651881032,-16.1741003483714,
25.1767480462244)) ;
#57189=CARTESIAN_POINT('Ctrl Pts',(-11.4852346439277,-14.0550299934948,
24.8540230124763)) ;
#57190=CARTESIAN_POINT('Ctrl Pts',(-11.3184718899869,-11.6664005713927,
24.4901998913042)) ;
#57191=CARTESIAN_POINT('Ctrl Pts',(-11.1555753225574,-9.32889248183853,
24.1340258244603)) ;
#57192=CARTESIAN_POINT('Ctrl Pts',(-11.0533843889444,-7.86334458038693,
23.910742887255)) ;
#57193=CARTESIAN_POINT('Ctrl Pts',(-10.8799081843125,-5.36524737160743,
23.5298164000503)) ;
#57194=CARTESIAN_POINT('Ctrl Pts',(-10.8093853863934,-4.34699231493492,
23.3744590058058)) ;
#57195=CARTESIAN_POINT('Ctrl Pts',(-10.7429209444356,-3.37610897447703,
23.2259695204405)) ;
#57196=CARTESIAN_POINT('Ctrl Pts',(-10.7272704888776,-3.14471287330663,
23.1904910996795)) ;
#57197=CARTESIAN_POINT('Ctrl Pts',(-10.7198900306606,-3.02956785456265,
23.1726482154596)) ;
#57198=CARTESIAN_POINT('Ctrl Pts',(-10.7191517661507,-3.01792892777941,
23.1708410575628)) ;
#57199=CARTESIAN_POINT('Ctrl Pts',(-10.718155837799,-3.0017485997851,23.1683146988345)) ;
#57200=CARTESIAN_POINT('Ctrl Pts',(-10.7177561124938,-2.99514906175769,
23.1672812605971)) ;
#57201=CARTESIAN_POINT('Ctrl Pts',(-10.7172513792382,-2.98634347416415,
23.1658891353251)) ;
#57202=CARTESIAN_POINT('Ctrl Pts',(-10.7169086091624,-2.98025788613349,
23.1649242294489)) ;
#57203=CARTESIAN_POINT('Ctrl Pts',(-10.7167289165089,-2.97566524671235,
23.1641594959843)) ;
#57204=CARTESIAN_POINT('Ctrl Pts',(-10.716699744908,-2.97457162490568,23.1639710936711)) ;
#57205=CARTESIAN_POINT('Ctrl Pts',(-10.7167384565843,-2.97437271210288,
23.1639164615673)) ;
#57206=CARTESIAN_POINT('Ctrl Pts',(-10.7167476789213,-2.97432532480766,
23.1639034464702)) ;
#57207=CARTESIAN_POINT('Ctrl Pts',(-10.7167569012583,-2.97427793751245,
23.1638904313731)) ;
#57208=CARTESIAN_POINT('',(-11.6595608585908,-16.2025431678319,25.1698333323831)) ;
#57209=CARTESIAN_POINT('Origin',(0.376819110642888,-21.5586464785791,-0.81448115993236)) ;
#57210=CARTESIAN_POINT('Ctrl Pts',(-10.7167569012583,-2.97427793751246,
23.163890431373)) ;
#57211=CARTESIAN_POINT('Ctrl Pts',(-10.7167705770044,-2.97432596381794,
23.1638929706548)) ;
#57212=CARTESIAN_POINT('Ctrl Pts',(-10.7167842527504,-2.97437399012343,
23.1638955099365)) ;
#57213=CARTESIAN_POINT('Ctrl Pts',(-10.7170423164564,-2.97528025486022,
23.1639434266246)) ;
#57214=CARTESIAN_POINT('Ctrl Pts',(-10.7179683584633,-2.98643371533908,
23.1655740852485)) ;
#57215=CARTESIAN_POINT('Ctrl Pts',(-10.7267027186728,-3.0914576706438,23.1809220919597)) ;
#57216=CARTESIAN_POINT('Ctrl Pts',(-10.7692656529469,-3.6819918304019,23.2702515899602)) ;
#57217=CARTESIAN_POINT('Ctrl Pts',(-10.9623645657162,-6.36109345723266,
23.6755157069365)) ;
#57218=CARTESIAN_POINT('Ctrl Pts',(-11.6012362667214,-15.3793218860576,
25.0448385213858)) ;
#57219=CARTESIAN_POINT('Ctrl Pts',(-11.6595608585848,-16.2025431677229,
25.1698333323657)) ;
#57220=CARTESIAN_POINT('',(-15.4457568027361,-2.97427793608127,20.3185455969618)) ;
#57221=CARTESIAN_POINT('Origin',(-5.46365993374796E-16,-2.97427793741672,
0.)) ;
#57222=CARTESIAN_POINT('',(-16.7764141848438,-16.2025431678318,22.0911248354107)) ;
#57223=CARTESIAN_POINT('Ctrl Pts',(-16.7764141848437,-16.2025431678318,
22.0911248354107)) ;
#57224=CARTESIAN_POINT('Ctrl Pts',(-16.7752198634206,-16.190713841179,22.0895430472459)) ;
#57225=CARTESIAN_POINT('Ctrl Pts',(-16.7740266741282,-16.1788957010685,
22.0879627528603)) ;
#57226=CARTESIAN_POINT('Ctrl Pts',(-16.5603070515992,-14.0620696485942,
21.8049052958167)) ;
#57227=CARTESIAN_POINT('Ctrl Pts',(-16.3192597867892,-11.6737192528371,
21.4854747478875)) ;
#57228=CARTESIAN_POINT('Ctrl Pts',(-16.0835676324059,-9.33584946938956,
21.1725978744201)) ;
#57229=CARTESIAN_POINT('Ctrl Pts',(-15.9356042182785,-7.86869477874113,
20.97628848721)) ;
#57230=CARTESIAN_POINT('Ctrl Pts',(-15.6840608298526,-5.36827143780728,
20.6412491931078)) ;
#57231=CARTESIAN_POINT('Ctrl Pts',(-15.5817192347535,-4.34932190857903,
20.5045915876768)) ;
#57232=CARTESIAN_POINT('Ctrl Pts',(-15.4847363587165,-3.37693719727565,
20.3736607611576)) ;
#57233=CARTESIAN_POINT('Ctrl Pts',(-15.4617693823315,-3.1449852959358,20.3423014857958)) ;
#57234=CARTESIAN_POINT('Ctrl Pts',(-15.4507050345335,-3.02962747694642,
20.3264333232862)) ;
#57235=CARTESIAN_POINT('Ctrl Pts',(-15.4495943826826,-3.01797675837514,
20.324825522346)) ;
#57236=CARTESIAN_POINT('Ctrl Pts',(-15.4480775917176,-3.00178591878239,
20.3225709128349)) ;
#57237=CARTESIAN_POINT('Ctrl Pts',(-15.4474654051385,-2.99519054883672,
20.321648174563)) ;
#57238=CARTESIAN_POINT('Ctrl Pts',(-15.4466716458739,-2.98636916407357,
20.3203949606915)) ;
#57239=CARTESIAN_POINT('Ctrl Pts',(-15.4461313364807,-2.98030508165379,
20.3195294015113)) ;
#57240=CARTESIAN_POINT('Ctrl Pts',(-15.4458171571932,-2.97607071487635,
20.3188770382006)) ;
#57241=CARTESIAN_POINT('Ctrl Pts',(-15.4456372043608,-2.97516294137418,
20.3188227779353)) ;
#57242=CARTESIAN_POINT('Ctrl Pts',(-15.4457440117809,-2.97437258105023,
20.3185752400619)) ;
#57243=CARTESIAN_POINT('Ctrl Pts',(-15.4457504068511,-2.97432525840346,
20.3185604187873)) ;
#57244=CARTESIAN_POINT('Ctrl Pts',(-15.4457568019214,-2.97427793575669,
20.3185455975128)) ;
#57245=CARTESIAN_POINT('',(-16.7977369565509,-16.2025431678318,22.0749156857653)) ;
#57246=CARTESIAN_POINT('Origin',(0.543098662732483,-21.5586464785792,-0.71443407293372)) ;
#57247=CARTESIAN_POINT('Ctrl Pts',(-15.4457568025556,-2.97427793106408,
20.3185455960431)) ;
#57248=CARTESIAN_POINT('Ctrl Pts',(-15.4457694984367,-2.9743262894881,20.3185461227573)) ;
#57249=CARTESIAN_POINT('Ctrl Pts',(-15.4457821943179,-2.97437464791213,
20.3185466494715)) ;
#57250=CARTESIAN_POINT('Ctrl Pts',(-15.4464212757398,-2.97680889962313,
20.3185731630504)) ;
#57251=CARTESIAN_POINT('Ctrl Pts',(-15.4464747921446,-2.97934518644453,
20.3190662866477)) ;
#57252=CARTESIAN_POINT('Ctrl Pts',(-15.4504481397431,-3.01314189784647,
20.323158932543)) ;
#57253=CARTESIAN_POINT('Ctrl Pts',(-15.4638357589392,-3.14117566784154,
20.3399288645903)) ;
#57254=CARTESIAN_POINT('Ctrl Pts',(-15.5746903197145,-4.20201721913459,
20.4789319888574)) ;
#57255=CARTESIAN_POINT('Ctrl Pts',(-16.0994049025687,-9.34914228273644,
21.1633563985944)) ;
#57256=CARTESIAN_POINT('Ctrl Pts',(-16.3547359668196,-11.8530767546699,
21.4962553652859)) ;
#57257=CARTESIAN_POINT('Ctrl Pts',(-16.588974741721,-14.1525006000269,21.8021454522111)) ;
#57258=CARTESIAN_POINT('Ctrl Pts',(-16.7977369565519,-16.2025431678313,
22.0749156857645)) ;
#57259=CARTESIAN_POINT('',(-19.4525302835701,-2.97427793904102,16.5231281535061)) ;
#57260=CARTESIAN_POINT('Origin',(-5.46365993374796E-16,-2.97427793741672,
0.)) ;
#57261=CARTESIAN_POINT('',(-21.1331297746477,-16.2025431678318,17.9682134705436)) ;
#57262=CARTESIAN_POINT('Ctrl Pts',(-21.1331297746474,-16.2025431678318,
17.9682134705439)) ;
#57263=CARTESIAN_POINT('Ctrl Pts',(-21.1316374631217,-16.1908247582476,
17.9669374849658)) ;
#57264=CARTESIAN_POINT('Ctrl Pts',(-21.1301452569594,-16.1791071590717,
17.965661585088)) ;
#57265=CARTESIAN_POINT('Ctrl Pts',(-20.8605852292292,-14.0623748808398,
17.7351754744795)) ;
#57266=CARTESIAN_POINT('Ctrl Pts',(-20.5565069219806,-11.6740365940616,
17.4750324022608)) ;
#57267=CARTESIAN_POINT('Ctrl Pts',(-20.259063823058,-9.33615114006502,17.2201355811663)) ;
#57268=CARTESIAN_POINT('Ctrl Pts',(-20.0723501178403,-7.86892678670822,
17.0602159811398)) ;
#57269=CARTESIAN_POINT('Ctrl Pts',(-19.7546512798608,-5.36840259178783,
16.7870731379981)) ;
#57270=CARTESIAN_POINT('Ctrl Pts',(-19.6253211866005,-4.34942295199821,
16.6756076595711)) ;
#57271=CARTESIAN_POINT('Ctrl Pts',(-19.5024511712846,-3.37697313538146,
16.5685792814353)) ;
#57272=CARTESIAN_POINT('Ctrl Pts',(-19.473276780477,-3.14499712523272,16.5428877433583)) ;
#57273=CARTESIAN_POINT('Ctrl Pts',(-19.4590587751061,-3.02963007194482,
16.5297680413151)) ;
#57274=CARTESIAN_POINT('Ctrl Pts',(-19.4576283953209,-3.01797883744602,
16.5284365298052)) ;
#57275=CARTESIAN_POINT('Ctrl Pts',(-19.4556623320526,-3.00178752696938,
16.5265606453689)) ;
#57276=CARTESIAN_POINT('Ctrl Pts',(-19.4548661148076,-2.9951923179276,16.5257911024352)) ;
#57277=CARTESIAN_POINT('Ctrl Pts',(-19.4538214301102,-2.98637030522913,
16.5247377534462)) ;
#57278=CARTESIAN_POINT('Ctrl Pts',(-19.4531077541231,-2.98030684070767,
16.524008657544)) ;
#57279=CARTESIAN_POINT('Ctrl Pts',(-19.4526605493631,-2.97607144563206,
16.5234389746291)) ;
#57280=CARTESIAN_POINT('Ctrl Pts',(-19.4524720868882,-2.97516264973382,
16.5234256419414)) ;
#57281=CARTESIAN_POINT('Ctrl Pts',(-19.4525240609173,-2.97437254348245,
16.5231599642006)) ;
#57282=CARTESIAN_POINT('Ctrl Pts',(-19.4525271723989,-2.9743252428848,16.5231440591025)) ;
#57283=CARTESIAN_POINT('Ctrl Pts',(-19.4525302838691,-2.97427794228964,
16.5231281539948)) ;
#57284=CARTESIAN_POINT('',(-21.1504695437717,-16.2025431678318,17.9477995161833)) ;
#57285=CARTESIAN_POINT('Origin',(0.683983524963512,-21.5586464785791,-0.580980842721122)) ;
#57286=CARTESIAN_POINT('Ctrl Pts',(-19.4525302838691,-2.97427794228965,
16.5231281539948)) ;
#57287=CARTESIAN_POINT('Ctrl Pts',(-19.4525427535086,-2.97432631415661,
16.5231259928427)) ;
#57288=CARTESIAN_POINT('Ctrl Pts',(-19.452555223148,-2.97437468602357,16.5231238316906)) ;
#57289=CARTESIAN_POINT('Ctrl Pts',(-19.4531824648511,-2.97680786400913,
16.5230151224743)) ;
#57290=CARTESIAN_POINT('Ctrl Pts',(-19.4533427230956,-2.97934036345287,
16.523481894319)) ;
#57291=CARTESIAN_POINT('Ctrl Pts',(-19.458120904464,-3.01326272602979,16.5266361147738)) ;
#57292=CARTESIAN_POINT('Ctrl Pts',(-19.4749326989184,-3.14232006038648,
16.5402453876941)) ;
#57293=CARTESIAN_POINT('Ctrl Pts',(-19.6134421521223,-4.20603554880853,
16.65248228589)) ;
#57294=CARTESIAN_POINT('Ctrl Pts',(-20.2727144713711,-9.35077018734797,
17.2078483873162)) ;
#57295=CARTESIAN_POINT('Ctrl Pts',(-20.593580039196,-11.8542418942229,17.4780259333328)) ;
#57296=CARTESIAN_POINT('Ctrl Pts',(-20.8880093579677,-14.1529599452982,
17.726333838428)) ;
#57297=CARTESIAN_POINT('Ctrl Pts',(-21.1504695437716,-16.2025431678313,
17.9477995161832)) ;
#57298=CARTESIAN_POINT('',(-22.5497250681625,-2.97427793560092,11.9551076001539)) ;
#57299=CARTESIAN_POINT('Origin',(-5.46365993374796E-16,-2.97427793741672,
0.)) ;
#57300=CARTESIAN_POINT('',(-24.5016837039787,-16.2025431678318,13.005128414026)) ;
#57301=CARTESIAN_POINT('Ctrl Pts',(-24.5016837039782,-16.2025431678318,
13.0051284140269)) ;
#57302=CARTESIAN_POINT('Ctrl Pts',(-24.4996676420489,-16.1889006495292,
13.0040511248088)) ;
#57303=CARTESIAN_POINT('Ctrl Pts',(-24.4976524169855,-16.1752637798932,
13.0029742776455)) ;
#57304=CARTESIAN_POINT('Ctrl Pts',(-24.1845818021322,-14.0567372972925,
12.8356823852449)) ;
#57305=CARTESIAN_POINT('Ctrl Pts',(-23.8316567265512,-11.6681756060599,
12.6469712655301)) ;
#57306=CARTESIAN_POINT('Ctrl Pts',(-23.4864154829261,-9.33057976204126,
12.4619975963323)) ;
#57307=CARTESIAN_POINT('Ctrl Pts',(-23.269879341362,-7.86464212508095,12.34605621553)) ;
#57308=CARTESIAN_POINT('Ctrl Pts',(-22.9011691865421,-5.36600381543967,
12.1477438959469)) ;
#57309=CARTESIAN_POINT('Ctrl Pts',(-22.7509867332351,-4.34760394628317,
12.0667321657766)) ;
#57310=CARTESIAN_POINT('Ctrl Pts',(-22.6081554098183,-3.37633177831297,
11.9887125870729)) ;
#57311=CARTESIAN_POINT('Ctrl Pts',(-22.5742032273907,-3.14478388077979,
11.9699275781758)) ;
#57312=CARTESIAN_POINT('Ctrl Pts',(-22.5575213999732,-3.02958227422016,
11.9601847498191)) ;
#57313=CARTESIAN_POINT('Ctrl Pts',(-22.5558396144626,-3.01794052653865,
11.9591926323437)) ;
#57314=CARTESIAN_POINT('Ctrl Pts',(-22.5535174978171,-3.00175763485085,
11.9577839214564)) ;
#57315=CARTESIAN_POINT('Ctrl Pts',(-22.5525739903808,-2.99515898007651,
11.9572031990715)) ;
#57316=CARTESIAN_POINT('Ctrl Pts',(-22.55132911353,-2.98634939833744,11.9564000619532)) ;
#57317=CARTESIAN_POINT('Ctrl Pts',(-22.5504731163466,-2.9802696426833,11.95583989009)) ;
#57318=CARTESIAN_POINT('Ctrl Pts',(-22.549917036684,-2.97605518832563,11.9553812397866)) ;
#57319=CARTESIAN_POINT('Ctrl Pts',(-22.549743958395,-2.97516568496484,11.9553895210276)) ;
#57320=CARTESIAN_POINT('Ctrl Pts',(-22.5497270953284,-2.97437322186437,
11.9551378608054)) ;
#57321=CARTESIAN_POINT('Ctrl Pts',(-22.5497260814769,-2.97432557691684,
11.9551227303367)) ;
#57322=CARTESIAN_POINT('Ctrl Pts',(-22.5497250676253,-2.97427793196933,
11.9551075998681)) ;
#57323=CARTESIAN_POINT('',(-24.5142296821799,-16.2025431678318,12.9814641887753)) ;
#57324=CARTESIAN_POINT('Origin',(0.792886077760343,-21.5586464785791,-0.420361594016722)) ;
#57325=CARTESIAN_POINT('Ctrl Pts',(-22.5497250676253,-2.97427793196933,
11.9551075998681)) ;
#57326=CARTESIAN_POINT('Ctrl Pts',(-22.5497352940808,-2.97432684211101,
11.9551058060875)) ;
#57327=CARTESIAN_POINT('Ctrl Pts',(-22.5497455205363,-2.97437575225269,
11.9551040123068)) ;
#57328=CARTESIAN_POINT('Ctrl Pts',(-22.5499048520773,-2.97513778835108,
11.9550760646145)) ;
#57329=CARTESIAN_POINT('Ctrl Pts',(-22.5500439827512,-2.97596782595578,
11.9551105442205)) ;
#57330=CARTESIAN_POINT('Ctrl Pts',(-22.5514940525204,-2.98473527704851,
11.9555115761301)) ;
#57331=CARTESIAN_POINT('Ctrl Pts',(-22.5558837380948,-3.01362289847503,
11.9575649728667)) ;
#57332=CARTESIAN_POINT('Ctrl Pts',(-22.5895429583672,-3.23583015028412,
11.9735614046487)) ;
#57333=CARTESIAN_POINT('Ctrl Pts',(-22.7007162739326,-3.98248101845175,
12.0309463354103)) ;
#57334=CARTESIAN_POINT('Ctrl Pts',(-22.9981001655269,-5.9830848446617,12.185645166953)) ;
#57335=CARTESIAN_POINT('Ctrl Pts',(-23.1944779036023,-7.30595314390739,
12.2884330665384)) ;
#57336=CARTESIAN_POINT('Ctrl Pts',(-23.4213140715843,-8.83439078112419,
12.4073031199904)) ;
#57337=CARTESIAN_POINT('Ctrl Pts',(-23.4860190491741,-9.27052278052022,
12.4412627181695)) ;
#57338=CARTESIAN_POINT('Ctrl Pts',(-23.8053430784459,-11.4225775147922,
12.6087526144909)) ;
#57339=CARTESIAN_POINT('Ctrl Pts',(-24.1472874488276,-13.7281025785756,
12.7884729898918)) ;
#57340=CARTESIAN_POINT('Ctrl Pts',(-24.4735167425919,-15.9279951058929,
12.9600499578252)) ;
#57341=CARTESIAN_POINT('Ctrl Pts',(-24.4939674190775,-16.0659036750085,
12.9708063576517)) ;
#57342=CARTESIAN_POINT('Ctrl Pts',(-24.5142296821805,-16.2025431678318,
12.981464188774)) ;
#57343=CARTESIAN_POINT('',(-24.592552107853,-2.97439688780173,6.82803753488347)) ;
#57344=CARTESIAN_POINT('Origin',(-5.46365993374796E-16,-2.97427793741672,
0.)) ;
#57345=CARTESIAN_POINT('',(-26.7245661349767,-16.2025431678318,7.43393800703095)) ;
#57346=CARTESIAN_POINT('Ctrl Pts',(-26.7245661349768,-16.2025431678313,
7.43393800703048)) ;
#57347=CARTESIAN_POINT('Ctrl Pts',(-26.6689832159522,-15.8579457768539,
7.41830998820638)) ;
#57348=CARTESIAN_POINT('Ctrl Pts',(-26.6124202750428,-15.5072677851224,
7.40240343975473)) ;
#57349=CARTESIAN_POINT('Ctrl Pts',(-26.3507918514815,-13.8852011858705,
7.3288117644863)) ;
#57350=CARTESIAN_POINT('Ctrl Pts',(-26.1359705189235,-12.5532595769792,
7.26833999538627)) ;
#57351=CARTESIAN_POINT('Ctrl Pts',(-25.877434070244,-10.95010355525,7.19545563196677)) ;
#57352=CARTESIAN_POINT('Ctrl Pts',(-25.8274200724287,-10.6399639551473,
7.18135091155874)) ;
#57353=CARTESIAN_POINT('Ctrl Pts',(-25.7535520225924,-10.1818898397547,
7.16051008425751)) ;
#57354=CARTESIAN_POINT('Ctrl Pts',(-25.7125628705679,-9.92770194704203,
7.1489430778947)) ;
#57355=CARTESIAN_POINT('Ctrl Pts',(-25.6721063124177,-9.6768097016269,7.13752188896885)) ;
#57356=CARTESIAN_POINT('Ctrl Pts',(-25.6516451009408,-9.54991748949785,
7.13174456271593)) ;
#57357=CARTESIAN_POINT('Ctrl Pts',(-25.6480238982615,-9.52746023152702,
7.13072208912283)) ;
#57358=CARTESIAN_POINT('Ctrl Pts',(-25.5859834329005,-9.14270729296583,
7.11320283416776)) ;
#57359=CARTESIAN_POINT('Ctrl Pts',(-25.3739725568845,-7.8279579923284,7.05337615177815)) ;
#57360=CARTESIAN_POINT('Ctrl Pts',(-25.0488113106629,-5.81059539629016,
6.96103715749616)) ;
#57361=CARTESIAN_POINT('Ctrl Pts',(-24.9410807235872,-5.14207211743425,
6.93035492624889)) ;
#57362=CARTESIAN_POINT('Ctrl Pts',(-24.766903337543,-4.06065733928159,6.88040057681779)) ;
#57363=CARTESIAN_POINT('Ctrl Pts',(-24.6971464703163,-3.62728003610139,
6.86022009636915)) ;
#57364=CARTESIAN_POINT('Ctrl Pts',(-24.630044306151,-3.20962006541524,6.84032192534756)) ;
#57365=CARTESIAN_POINT('Ctrl Pts',(-24.6139309219069,-3.10915131540964,
6.83543402113868)) ;
#57366=CARTESIAN_POINT('Ctrl Pts',(-24.6021451332267,-3.03535094781093,
6.83166179919274)) ;
#57367=CARTESIAN_POINT('Ctrl Pts',(-24.6002338489497,-3.02336908310285,
6.83104144184553)) ;
#57368=CARTESIAN_POINT('Ctrl Pts',(-24.5972607462002,-3.0046695511412,6.83003816803247)) ;
#57369=CARTESIAN_POINT('Ctrl Pts',(-24.5961100776802,-2.99742051577194,
6.82964246735651)) ;
#57370=CARTESIAN_POINT('Ctrl Pts',(-24.5946263153786,-2.98801463919662,
6.82909564333515)) ;
#57371=CARTESIAN_POINT('Ctrl Pts',(-24.59337944986,-2.97996100765901,6.82854250312845)) ;
#57372=CARTESIAN_POINT('Ctrl Pts',(-24.5925577081587,-2.97451596139029,
6.82809194035633)) ;
#57373=CARTESIAN_POINT('Ctrl Pts',(-24.5925713143705,-2.97451583818675,
6.82804285739138)) ;
#57374=CARTESIAN_POINT('',(-26.7317316862594,-16.2025431678318,7.40813002376167)) ;
#57375=CARTESIAN_POINT('Origin',(0.864714158790679,-21.5586464785792,-0.240086704374452)) ;
#57376=CARTESIAN_POINT('Ctrl Pts',(-24.5925713143603,-2.97451583818853,
6.82804285738853)) ;
#57377=CARTESIAN_POINT('Ctrl Pts',(-24.5925806259886,-2.97456488239044,
6.82804003606991)) ;
#57378=CARTESIAN_POINT('Ctrl Pts',(-24.5925899376168,-2.97461392659235,
6.82803721475129)) ;
#57379=CARTESIAN_POINT('Ctrl Pts',(-24.5937332774705,-2.98063587992714,
6.82769079563499)) ;
#57380=CARTESIAN_POINT('Ctrl Pts',(-24.5945770239903,-2.98636186716204,
6.82823805211795)) ;
#57381=CARTESIAN_POINT('Ctrl Pts',(-24.6080089005343,-3.06781746902136,
6.83087603583482)) ;
#57382=CARTESIAN_POINT('Ctrl Pts',(-24.6568415415074,-3.36899802404575,
6.84362461449725)) ;
#57383=CARTESIAN_POINT('Ctrl Pts',(-24.6710163121772,-3.45642106171283,
6.84732431020992)) ;
#57384=CARTESIAN_POINT('Ctrl Pts',(-24.6728723965344,-3.46786980995301,
6.84780959155663)) ;
#57385=CARTESIAN_POINT('Ctrl Pts',(-24.8318196304806,-4.44835604177014,
6.88940695397689)) ;
#57386=CARTESIAN_POINT('Ctrl Pts',(-25.2480074862592,-7.02233073853014,
7.00250108447751)) ;
#57387=CARTESIAN_POINT('Ctrl Pts',(-25.628103213734,-9.37363014663993,7.10612690748992)) ;
#57388=CARTESIAN_POINT('Ctrl Pts',(-25.7147409830227,-9.90964877679412,
7.12979161674918)) ;
#57389=CARTESIAN_POINT('Ctrl Pts',(-25.7418193097697,-10.0771773232176,
7.13718657805486)) ;
#57390=CARTESIAN_POINT('Ctrl Pts',(-25.7451959194303,-10.0980678317341,
7.13810874883747)) ;
#57391=CARTESIAN_POINT('Ctrl Pts',(-26.0669352634096,-12.0886187181864,
7.22598029792739)) ;
#57392=CARTESIAN_POINT('Ctrl Pts',(-26.4160920844778,-14.2492145131363,
7.32160128400388)) ;
#57393=CARTESIAN_POINT('Ctrl Pts',(-26.7317316862593,-16.2025431678313,
7.40813002376179)) ;
#57394=CARTESIAN_POINT('',(-25.4853955845497,-2.97427793815454,1.38177794953793)) ;
#57395=CARTESIAN_POINT('Origin',(-5.46365993374796E-16,-2.97427793741672,
0.)) ;
#57396=CARTESIAN_POINT('',(-27.6978375557248,-16.2025431678318,1.51514492105713)) ;
#57397=CARTESIAN_POINT('Ctrl Pts',(-27.6978375557247,-16.2025431678318,
1.51514492105922)) ;
#57398=CARTESIAN_POINT('Ctrl Pts',(-27.6949483747658,-16.1852712613029,
1.51497881880076)) ;
#57399=CARTESIAN_POINT('Ctrl Pts',(-27.6920606024541,-16.1680077735078,
1.51481279026704)) ;
#57400=CARTESIAN_POINT('Ctrl Pts',(-27.3371143876217,-14.0460917001996,
1.49440474478063)) ;
#57401=CARTESIAN_POINT('Ctrl Pts',(-26.9374998132548,-11.6571071294358,
1.47131995388038)) ;
#57402=CARTESIAN_POINT('Ctrl Pts',(-26.5465905728723,-9.32005883265994,
1.4484095511999)) ;
#57403=CARTESIAN_POINT('Ctrl Pts',(-26.3017916915238,-7.8565516409229,1.43412818138653)) ;
#57404=CARTESIAN_POINT('Ctrl Pts',(-25.8844750239149,-5.3614086784368,1.40899545055731)) ;
#57405=CARTESIAN_POINT('Ctrl Pts',(-25.7143289878448,-4.34403568291514,
1.39854061302158)) ;
#57406=CARTESIAN_POINT('Ctrl Pts',(-25.5523230854378,-3.37505853243338,
1.3877275070587)) ;
#57407=CARTESIAN_POINT('Ctrl Pts',(-25.5137645868328,-3.14436762856298,
1.38494407232914)) ;
#57408=CARTESIAN_POINT('Ctrl Pts',(-25.4945881657819,-3.02949231117301,
1.38311080631034)) ;
#57409=CARTESIAN_POINT('Ctrl Pts',(-25.4926481764263,-3.01786813916945,
1.38291676976861)) ;
#57410=CARTESIAN_POINT('Ctrl Pts',(-25.4899521301898,-3.00170290476441,
1.38261348814891)) ;
#57411=CARTESIAN_POINT('Ctrl Pts',(-25.4888514934502,-2.99510126826416,
1.38248248287018)) ;
#57412=CARTESIAN_POINT('Ctrl Pts',(-25.4873884466953,-2.98631563827613,
1.38227661114065)) ;
#57413=CARTESIAN_POINT('Ctrl Pts',(-25.486371196431,-2.98020487444517,1.38212680866863)) ;
#57414=CARTESIAN_POINT('Ctrl Pts',(-25.4856195768672,-2.97566139772543,
1.38192825014818)) ;
#57415=CARTESIAN_POINT('Ctrl Pts',(-25.4854468698752,-2.97461266012032,
1.38186796062895)) ;
#57416=CARTESIAN_POINT('Ctrl Pts',(-25.4854102201195,-2.9743734717481,1.38180367418922)) ;
#57417=CARTESIAN_POINT('Ctrl Pts',(-25.4854029011111,-2.97432570548941,
1.38179083609563)) ;
#57418=CARTESIAN_POINT('Ctrl Pts',(-25.4853955821027,-2.97427793923073,
1.38177799800203)) ;
#57419=CARTESIAN_POINT('',(-27.6992876268763,-16.2025431678318,1.48839993237876)) ;
#57420=CARTESIAN_POINT('Origin',(0.896109166816714,-21.5586464785791,-0.0485856272728462)) ;
#57421=CARTESIAN_POINT('Ctrl Pts',(-25.4853955876312,-2.97427794002965,
1.38177789850702)) ;
#57422=CARTESIAN_POINT('Ctrl Pts',(-25.4854041324089,-2.97432678140872,
1.38177145595585)) ;
#57423=CARTESIAN_POINT('Ctrl Pts',(-25.4854126771865,-2.97437562278778,
1.38176501340469)) ;
#57424=CARTESIAN_POINT('Ctrl Pts',(-25.4862266854511,-2.9790284397228,1.38115127129212)) ;
#57425=CARTESIAN_POINT('Ctrl Pts',(-25.4869891119617,-2.983689485392,1.38151436532657)) ;
#57426=CARTESIAN_POINT('Ctrl Pts',(-25.4974120488345,-3.04568905696004,
1.38115379950162)) ;
#57427=CARTESIAN_POINT('Ctrl Pts',(-25.5378627351659,-3.2872365214572,1.38263725546573)) ;
#57428=CARTESIAN_POINT('Ctrl Pts',(-25.7524643697489,-4.5686999147475,1.39047624847401)) ;
#57429=CARTESIAN_POINT('Ctrl Pts',(-26.5784759569267,-9.50471724369494,
1.4318077909381)) ;
#57430=CARTESIAN_POINT('Ctrl Pts',(-26.9899241868522,-11.9634061746525,
1.45235798347176)) ;
#57431=CARTESIAN_POINT('Ctrl Pts',(-27.363591331709,-14.1964160924647,1.47129725231825)) ;
#57432=CARTESIAN_POINT('Ctrl Pts',(-27.6992876268763,-16.2025431678313,
1.48839993237614)) ;
#57433=CARTESIAN_POINT('',(-25.1866026070031,-2.97427793714977,-4.12913399045467)) ;
#57434=CARTESIAN_POINT('Origin',(-5.46365993374796E-16,-2.97427793741672,
0.)) ;
#57435=CARTESIAN_POINT('',(-27.3759888763025,-16.2025431678318,-4.47449465746571)) ;
#57436=CARTESIAN_POINT('Ctrl Pts',(-27.3759888763025,-16.2025431678318,
-4.4744946574655)) ;
#57437=CARTESIAN_POINT('Ctrl Pts',(-27.3732094220677,-16.1857420647624,
-4.47404829586599)) ;
#57438=CARTESIAN_POINT('Ctrl Pts',(-27.3704308025602,-16.1689460141171,
-4.47360207526417)) ;
#57439=CARTESIAN_POINT('Ctrl Pts',(-27.0194681712013,-14.0474667151253,
-4.41724160356195)) ;
#57440=CARTESIAN_POINT('Ctrl Pts',(-26.6242428750162,-11.658536835958,-4.35388274751894)) ;
#57441=CARTESIAN_POINT('Ctrl Pts',(-26.2375361320519,-9.32141776666402,
-4.29222155923528)) ;
#57442=CARTESIAN_POINT('Ctrl Pts',(-25.9953385064225,-7.85759660285274,
-4.25353612774431)) ;
#57443=CARTESIAN_POINT('Ctrl Pts',(-25.5823004912435,-5.36199912354941,
-4.18835840434003)) ;
#57444=CARTESIAN_POINT('Ctrl Pts',(-25.4138624515631,-4.34449041737206,
-4.16198878709876)) ;
#57445=CARTESIAN_POINT('Ctrl Pts',(-25.2532711456091,-3.37522003933381,
-4.13771484198824)) ;
#57446=CARTESIAN_POINT('Ctrl Pts',(-25.2149978063456,-3.14442068934507,
-4.13214150615795)) ;
#57447=CARTESIAN_POINT('Ctrl Pts',(-25.1958687361614,-3.02950392952988,
-4.12980862521967)) ;
#57448=CARTESIAN_POINT('Ctrl Pts',(-25.1939320152815,-3.01787749563495,
-4.12958103145751)) ;
#57449=CARTESIAN_POINT('Ctrl Pts',(-25.1912333983801,-3.00170981125287,
-4.1292975922956)) ;
#57450=CARTESIAN_POINT('Ctrl Pts',(-25.1901303432712,-2.99510823617433,
-4.12918892312608)) ;
#57451=CARTESIAN_POINT('Ctrl Pts',(-25.1886567289002,-2.98631949906856,
-4.12907540246666)) ;
#57452=CARTESIAN_POINT('Ctrl Pts',(-25.1876317161037,-2.98021264730425,
-4.1290030629297)) ;
#57453=CARTESIAN_POINT('Ctrl Pts',(-25.1868539544775,-2.97566296777208,
-4.12903526378729)) ;
#57454=CARTESIAN_POINT('Ctrl Pts',(-25.1866710372384,-2.97460670643535,
-4.12905707867674)) ;
#57455=CARTESIAN_POINT('Ctrl Pts',(-25.1866224802819,-2.97437337212036,
-4.12911160736365)) ;
#57456=CARTESIAN_POINT('Ctrl Pts',(-25.1866125500831,-2.97432565381897,
-4.12912275881491)) ;
#57457=CARTESIAN_POINT('Ctrl Pts',(-25.1866026198728,-2.97427793551953,
-4.12913391026427)) ;
#57458=CARTESIAN_POINT('',(-27.3716556636072,-16.2025431678318,-4.50092608560145)) ;
#57459=CARTESIAN_POINT('Origin',(0.885603106156221,-21.5586464785792,0.145187259760995)) ;
#57460=CARTESIAN_POINT('Ctrl Pts',(-25.1866025936503,-2.97427793771224,
-4.12913407248572)) ;
#57461=CARTESIAN_POINT('Ctrl Pts',(-25.1866095211381,-2.97432675457791,
-4.12914237450595)) ;
#57462=CARTESIAN_POINT('Ctrl Pts',(-25.1866164486258,-2.97437557144357,
-4.12915067652617)) ;
#57463=CARTESIAN_POINT('Ctrl Pts',(-25.1869254243862,-2.97655287275656,
-4.12952095838038)) ;
#57464=CARTESIAN_POINT('Ctrl Pts',(-25.1903482932883,-2.99746421379417,
-4.13029948590828)) ;
#57465=CARTESIAN_POINT('Ctrl Pts',(-25.2317140552067,-3.25010212170233,
-4.13962725825562)) ;
#57466=CARTESIAN_POINT('Ctrl Pts',(-25.5134259808611,-4.95579873516529,
-4.18778756473923)) ;
#57467=CARTESIAN_POINT('Ctrl Pts',(-26.0153659193611,-7.99520368216468,
-4.27388892128809)) ;
#57468=CARTESIAN_POINT('Ctrl Pts',(-26.9798765474653,-13.831802071856,-4.43538391273868)) ;
#57469=CARTESIAN_POINT('Ctrl Pts',(-27.3716556636063,-16.2025431678262,
-4.500926085601)) ;
#57470=CARTESIAN_POINT('',(-23.7101121128184,-2.97427793741671,-9.44697210719331)) ;
#57471=CARTESIAN_POINT('Origin',(-5.46365993374796E-16,-2.97427793741672,
0.)) ;
#57472=CARTESIAN_POINT('',(-25.7740693832513,-16.2025431678318,-10.2549118388445)) ;
#57473=CARTESIAN_POINT('Ctrl Pts',(-25.7740693832516,-16.2025431678318,
-10.2549118388438)) ;
#57474=CARTESIAN_POINT('Ctrl Pts',(-25.7717662057054,-16.1877653700843,
-10.254002864804)) ;
#57475=CARTESIAN_POINT('Ctrl Pts',(-25.7694634381093,-16.1729902152862,
-10.2530940582596)) ;
#57476=CARTESIAN_POINT('Ctrl Pts',(-25.4391163992136,-14.0533996573025,
-10.1227206511024)) ;
#57477=CARTESIAN_POINT('Ctrl Pts',(-25.0667883861616,-11.6647055239092,
-9.97589555283087)) ;
#57478=CARTESIAN_POINT('Ctrl Pts',(-24.702330635356,-9.32728125401795,-9.83252608174547)) ;
#57479=CARTESIAN_POINT('Ctrl Pts',(-24.473900641258,-7.86210553169967,-9.74259625848603)) ;
#57480=CARTESIAN_POINT('Ctrl Pts',(-24.0842249574383,-5.36454711554133,
-9.59003060362382)) ;
#57481=CARTESIAN_POINT('Ctrl Pts',(-23.925302428713,-4.34645292280116,-9.52803206672356)) ;
#57482=CARTESIAN_POINT('Ctrl Pts',(-23.7734866041964,-3.37591728035413,
-9.46972551968006)) ;
#57483=CARTESIAN_POINT('Ctrl Pts',(-23.7372330254185,-3.14464984931574,
-9.45602655707944)) ;
#57484=CARTESIAN_POINT('Ctrl Pts',(-23.7190244883969,-3.02955404144013,
-9.44962574507765)) ;
#57485=CARTESIAN_POINT('Ctrl Pts',(-23.7171804403966,-3.01791784367858,
-9.44898656105867)) ;
#57486=CARTESIAN_POINT('Ctrl Pts',(-23.7146042867674,-3.00174019075879,
-9.4481290283292)) ;
#57487=CARTESIAN_POINT('Ctrl Pts',(-23.7135506216482,-2.99514003796932,
-9.44778581572707)) ;
#57488=CARTESIAN_POINT('Ctrl Pts',(-23.7121337604259,-2.98633794087801,
-9.44735739531497)) ;
#57489=CARTESIAN_POINT('Ctrl Pts',(-23.7111510567275,-2.98024831805525,
-9.44706718623769)) ;
#57490=CARTESIAN_POINT('Ctrl Pts',(-23.7103793731646,-2.9756660058921,-9.44692967577819)) ;
#57491=CARTESIAN_POINT('Ctrl Pts',(-23.7101909070959,-2.97457957271177,
-9.44691089066687)) ;
#57492=CARTESIAN_POINT('Ctrl Pts',(-23.7101369135214,-2.97437287773465,
-9.44695283905479)) ;
#57493=CARTESIAN_POINT('Ctrl Pts',(-23.7101245131969,-2.97432540755282,
-9.44696247304605)) ;
#57494=CARTESIAN_POINT('Ctrl Pts',(-23.7101121128723,-2.97427793737098,
-9.4469721070373)) ;
#57495=CARTESIAN_POINT('',(-25.7641555029173,-16.2025431678318,-10.2797938022424)) ;
#57496=CARTESIAN_POINT('Origin',(0.833687228529012,-21.5586464785791,0.33217135189247)) ;
#57497=CARTESIAN_POINT('Ctrl Pts',(-23.7101121127218,-2.97427793679491,
-9.44697210715423)) ;
#57498=CARTESIAN_POINT('Ctrl Pts',(-23.7101153152554,-2.97432592122196,
-9.44698579066765)) ;
#57499=CARTESIAN_POINT('Ctrl Pts',(-23.7101185177891,-2.974373905649,-9.44699947418107)) ;
#57500=CARTESIAN_POINT('Ctrl Pts',(-23.7101786105686,-2.97527429200802,
-9.44725623350041)) ;
#57501=CARTESIAN_POINT('Ctrl Pts',(-23.7119047187706,-2.98673786471755,
-9.44811328134859)) ;
#57502=CARTESIAN_POINT('Ctrl Pts',(-23.7231965051006,-3.0618162915894,-9.4537590304828)) ;
#57503=CARTESIAN_POINT('Ctrl Pts',(-23.7746504249845,-3.39437532880271,
-9.47516001099938)) ;
#57504=CARTESIAN_POINT('Ctrl Pts',(-23.9939151254337,-4.81167572162242,
-9.56642109048687)) ;
#57505=CARTESIAN_POINT('Ctrl Pts',(-24.7425357318122,-9.62933838762751,
-9.868352084219)) ;
#57506=CARTESIAN_POINT('Ctrl Pts',(-25.118894856561,-12.051377463681,-10.0201542187415)) ;
#57507=CARTESIAN_POINT('Ctrl Pts',(-25.4578393533391,-14.2320211893607,
-10.1565867698155)) ;
#57508=CARTESIAN_POINT('Ctrl Pts',(-25.764155502917,-16.2025431678313,-10.279793802243)) ;
#57509=CARTESIAN_POINT('',(-21.124963114758,-2.97427793718828,-14.323080387775)) ;
#57510=CARTESIAN_POINT('Origin',(-5.46365993374796E-16,-2.97427793741672,
0.)) ;
#57511=CARTESIAN_POINT('',(-22.9669830516588,-16.2025431678318,-15.5558207401585)) ;
#57512=CARTESIAN_POINT('Ctrl Pts',(-22.9669830516587,-16.2025431678316,
-15.5558207401585)) ;
#57513=CARTESIAN_POINT('Ctrl Pts',(-22.9652569821592,-16.1901242777138,
-15.5546586379788)) ;
#57514=CARTESIAN_POINT('Ctrl Pts',(-22.9635303524359,-16.1777013719743,
-15.5534961631374)) ;
#57515=CARTESIAN_POINT('Ctrl Pts',(-22.6692388096402,-14.0603095716988,
-15.355361512148)) ;
#57516=CARTESIAN_POINT('Ctrl Pts',(-22.3372169635415,-11.6718894981187,
-15.131954939375)) ;
#57517=CARTESIAN_POINT('Ctrl Pts',(-22.0120512929729,-9.33411011503439,
-14.913555876619)) ;
#57518=CARTESIAN_POINT('Ctrl Pts',(-21.8080750291336,-7.86735711606076,
-14.7764750775493)) ;
#57519=CARTESIAN_POINT('Ctrl Pts',(-21.4599896090463,-5.36751530388756,
-14.5434937228485)) ;
#57520=CARTESIAN_POINT('Ctrl Pts',(-21.3180158530842,-4.34873938710956,
-14.4487170165588)) ;
#57521=CARTESIAN_POINT('Ctrl Pts',(-21.1820786906682,-3.37673005385096,
-14.3589999273775)) ;
#57522=CARTESIAN_POINT('Ctrl Pts',(-21.149541406992,-3.1449171459073,-14.3377772656239)) ;
#57523=CARTESIAN_POINT('Ctrl Pts',(-21.1331050331298,-3.02961255818415,
-14.3275930192541)) ;
#57524=CARTESIAN_POINT('Ctrl Pts',(-21.1314398779441,-3.01796480514944,
-14.3265713108627)) ;
#57525=CARTESIAN_POINT('Ctrl Pts',(-21.1291068134075,-3.00177651940637,
-14.3251790442246)) ;
#57526=CARTESIAN_POINT('Ctrl Pts',(-21.1281521135327,-2.99518000535374,
-14.3246176232549)) ;
#57527=CARTESIAN_POINT('Ctrl Pts',(-21.1268583161178,-2.98636255210082,
-14.3238932357542)) ;
#57528=CARTESIAN_POINT('Ctrl Pts',(-21.1259639730245,-2.98029308314374,
-14.3234001531875)) ;
#57529=CARTESIAN_POINT('Ctrl Pts',(-21.1252964678625,-2.9760653941696,-14.3231224034572)) ;
#57530=CARTESIAN_POINT('Ctrl Pts',(-21.1252289897392,-2.97516395667663,
-14.3229527870938)) ;
#57531=CARTESIAN_POINT('Ctrl Pts',(-21.1249915865035,-2.97437281950653,
-14.3230667237568)) ;
#57532=CARTESIAN_POINT('Ctrl Pts',(-21.1249773504602,-2.97432537843874,
-14.3230735560448)) ;
#57533=CARTESIAN_POINT('Ctrl Pts',(-21.1249631144169,-2.97427793737095,
-14.3230803883327)) ;
#57534=CARTESIAN_POINT('',(-22.9519520657146,-16.2025431678318,-15.577989785857)) ;
#57535=CARTESIAN_POINT('Origin',(0.742789062672589,-21.5586464785791,0.503623480791376)) ;
#57536=CARTESIAN_POINT('Ctrl Pts',(-21.124963114225,-2.9742779367314,-14.3230803884248)) ;
#57537=CARTESIAN_POINT('Ctrl Pts',(-21.1249638884685,-2.97432614272334,
-14.3230936391942)) ;
#57538=CARTESIAN_POINT('Ctrl Pts',(-21.1249646627119,-2.97437434871528,
-14.3231068899635)) ;
#57539=CARTESIAN_POINT('Ctrl Pts',(-21.1249800549334,-2.97533270010394,
-14.32337031973)) ;
#57540=CARTESIAN_POINT('Ctrl Pts',(-21.1263277956509,-2.98566687891167,
-14.3244679902124)) ;
#57541=CARTESIAN_POINT('Ctrl Pts',(-21.1418861653829,-3.10454524903057,
-14.3370142074003)) ;
#57542=CARTESIAN_POINT('Ctrl Pts',(-21.2400732682184,-3.81755457323848,
-14.4050797447424)) ;
#57543=CARTESIAN_POINT('Ctrl Pts',(-21.6283862075553,-6.63747712966605,
-14.6742953410927)) ;
#57544=CARTESIAN_POINT('Ctrl Pts',(-22.8396016024952,-15.3906091490516,
-15.5012780450194)) ;
#57545=CARTESIAN_POINT('Ctrl Pts',(-22.9519520656995,-16.2025431677232,
-15.5779897858469)) ;
#57546=CARTESIAN_POINT('',(-17.5520343210229,-2.97427793967815,-18.5294573479495)) ;
#57547=CARTESIAN_POINT('Origin',(-5.46365993374796E-16,-2.97427793741672,
0.)) ;
#57548=CARTESIAN_POINT('',(-19.0859861185405,-16.2025431678318,-20.1293567527133)) ;
#57549=CARTESIAN_POINT('Ctrl Pts',(-19.0859861185421,-16.2025431678318,
-20.1293567527118)) ;
#57550=CARTESIAN_POINT('Ctrl Pts',(-19.0846371298263,-16.1908759391215,
-20.1279419167462)) ;
#57551=CARTESIAN_POINT('Ctrl Pts',(-19.0832882729851,-16.179209871745,-20.1265272238852)) ;
#57552=CARTESIAN_POINT('Ctrl Pts',(-18.8385520769211,-14.0625257558835,
-19.8698466324083)) ;
#57553=CARTESIAN_POINT('Ctrl Pts',(-18.5623287580252,-11.6741934643914,
-19.5802988659292)) ;
#57554=CARTESIAN_POINT('Ctrl Pts',(-18.2917016367397,-9.33630026614505,
-19.297090878332)) ;
#57555=CARTESIAN_POINT('Ctrl Pts',(-18.1219041184186,-7.86904147581327,
-19.1193046978973)) ;
#57556=CARTESIAN_POINT('Ctrl Pts',(-17.8319562334904,-5.3684674257714,-18.8168533991059)) ;
#57557=CARTESIAN_POINT('Ctrl Pts',(-17.7136507220211,-4.34947290189771,
-18.6937457899545)) ;
#57558=CARTESIAN_POINT('Ctrl Pts',(-17.6001235387096,-3.37699090193947,
-18.5768464727248)) ;
#57559=CARTESIAN_POINT('Ctrl Pts',(-17.5728888219343,-3.14500297387669,
-18.5491043446499)) ;
#57560=CARTESIAN_POINT('Ctrl Pts',(-17.5590180714718,-3.02963135488066,
-18.5356169375373)) ;
#57561=CARTESIAN_POINT('Ctrl Pts',(-17.5576110433959,-3.01797986462699,
-18.5342607116337)) ;
#57562=CARTESIAN_POINT('Ctrl Pts',(-17.5556314417978,-3.00178831577416,
-18.5323990614106)) ;
#57563=CARTESIAN_POINT('Ctrl Pts',(-17.5548199352069,-2.99519321590349,
-18.5316456859648)) ;
#57564=CARTESIAN_POINT('Ctrl Pts',(-17.5537115426901,-2.98637094041825,
-18.530659528573)) ;
#57565=CARTESIAN_POINT('Ctrl Pts',(-17.5529448973719,-2.98030761516333,
-18.5299863859087)) ;
#57566=CARTESIAN_POINT('Ctrl Pts',(-17.5523517824303,-2.97607173941054,
-18.5295706214556)) ;
#57567=CARTESIAN_POINT('Ctrl Pts',(-17.5523287283435,-2.97516246709807,
-18.5293826094285)) ;
#57568=CARTESIAN_POINT('Ctrl Pts',(-17.5520658014124,-2.97437252302452,
-18.5294493569053)) ;
#57569=CARTESIAN_POINT('Ctrl Pts',(-17.5520500614881,-2.97432523361278,
-18.5294533526932)) ;
#57570=CARTESIAN_POINT('Ctrl Pts',(-17.5520343215638,-2.97427794420103,
-18.529457348481)) ;
#57571=CARTESIAN_POINT('',(-19.066540859179,-16.2025431678318,-20.1477762807805)) ;
#57572=CARTESIAN_POINT('Origin',(0.617158905796334,-21.5586464785791,0.651526735465776)) ;
#57573=CARTESIAN_POINT('Ctrl Pts',(-17.5520343215638,-2.97427794420103,
-18.529457348481)) ;
#57574=CARTESIAN_POINT('Ctrl Pts',(-17.5520328590378,-2.97432632137793,
-18.5294698987708)) ;
#57575=CARTESIAN_POINT('Ctrl Pts',(-17.5520313965119,-2.97437469855482,
-18.5294824490605)) ;
#57576=CARTESIAN_POINT('Ctrl Pts',(-17.5519578549723,-2.97680729268956,
-18.5301135268382)) ;
#57577=CARTESIAN_POINT('Ctrl Pts',(-17.5524313112944,-2.97933811808545,
-18.5302491313957)) ;
#57578=CARTESIAN_POINT('Ctrl Pts',(-17.5558459413838,-3.01332488184634,
-18.5348583870864)) ;
#57579=CARTESIAN_POINT('Ctrl Pts',(-17.570404533859,-3.14290217484017,-18.5509727463816)) ;
#57580=CARTESIAN_POINT('Ctrl Pts',(-17.6901444286037,-4.20807339287134,
-18.6833787023212)) ;
#57581=CARTESIAN_POINT('Ctrl Pts',(-18.2802487121423,-9.35159400823905,
-19.3114692894703)) ;
#57582=CARTESIAN_POINT('Ctrl Pts',(-18.5673745153853,-11.854831316873,-19.6172084675867)) ;
#57583=CARTESIAN_POINT('Ctrl Pts',(-18.8312173562081,-14.1531923295863,
-19.8977192805209)) ;
#57584=CARTESIAN_POINT('Ctrl Pts',(-19.066540859178,-16.2025431678313,-20.1477762807813)) ;
#57585=CARTESIAN_POINT('',(-13.1583919092399,-2.97427793887167,-21.8694174767368)) ;
#57586=CARTESIAN_POINT('Origin',(-5.46365993374796E-16,-2.97427793741672,
0.)) ;
#57587=CARTESIAN_POINT('',(-14.312549687069,-16.2025431678318,-23.7616664156853)) ;
#57588=CARTESIAN_POINT('Ctrl Pts',(-14.3125496870692,-16.2025431678318,
-23.7616664156852)) ;
#57589=CARTESIAN_POINT('Ctrl Pts',(-14.3114173894645,-16.1895058181297,
-23.7597983459377)) ;
#57590=CARTESIAN_POINT('Ctrl Pts',(-14.3102852112603,-16.1764698839562,
-23.7579304811446)) ;
#57591=CARTESIAN_POINT('Ctrl Pts',(-14.1263382038808,-14.0585051121798,
-23.4544564647785)) ;
#57592=CARTESIAN_POINT('Ctrl Pts',(-13.9188030305551,-11.6700134993328,
-23.1122755929955)) ;
#57593=CARTESIAN_POINT('Ctrl Pts',(-13.715401930735,-9.33232681200154,-22.7775418330419)) ;
#57594=CARTESIAN_POINT('Ctrl Pts',(-13.5878725388209,-7.86598567539764,
-22.5675423048878)) ;
#57595=CARTESIAN_POINT('Ctrl Pts',(-13.3698368359399,-5.36674011422468,
-22.2100223430801)) ;
#57596=CARTESIAN_POINT('Ctrl Pts',(-13.2807960510996,-4.34814220861965,
-22.0644176439079)) ;
#57597=CARTESIAN_POINT('Ctrl Pts',(-13.1951275032717,-3.37651773024291,
-21.9259692143185)) ;
#57598=CARTESIAN_POINT('Ctrl Pts',(-13.1745211431796,-3.14484730369312,
-21.8930663287957)) ;
#57599=CARTESIAN_POINT('Ctrl Pts',(-13.1638850913661,-3.02959728845171,
-21.8769295999609)) ;
#57600=CARTESIAN_POINT('Ctrl Pts',(-13.1628031114733,-3.01795255159799,
-21.8753035694779)) ;
#57601=CARTESIAN_POINT('Ctrl Pts',(-13.1612705151022,-3.00176698296443,
-21.8730607421964)) ;
#57602=CARTESIAN_POINT('Ctrl Pts',(-13.1606396748887,-2.99516939089294,
-21.8721501992151)) ;
#57603=CARTESIAN_POINT('Ctrl Pts',(-13.1597699751221,-2.98635593952167,
-21.8709500794992)) ;
#57604=CARTESIAN_POINT('Ctrl Pts',(-13.1591647786055,-2.98028104303356,
-21.8701263162042)) ;
#57605=CARTESIAN_POINT('Ctrl Pts',(-13.1586761512808,-2.97606009736442,
-21.869594940972)) ;
#57606=CARTESIAN_POINT('Ctrl Pts',(-13.1586802925452,-2.9751648529284,-21.8694173912168)) ;
#57607=CARTESIAN_POINT('Ctrl Pts',(-13.158422831361,-2.97437304087061,-21.8694174679499)) ;
#57608=CARTESIAN_POINT('Ctrl Pts',(-13.1584073704168,-2.97432549132609,
-21.8694174725579)) ;
#57609=CARTESIAN_POINT('Ctrl Pts',(-13.1583919094726,-2.97427794178158,
-21.8694174771658)) ;
#57610=CARTESIAN_POINT('',(-14.2895993930079,-16.2025431678318,-23.7754751494576)) ;
#57611=CARTESIAN_POINT('Origin',(0.462671084407919,-21.5586464785791,0.768965324109761)) ;
#57612=CARTESIAN_POINT('Ctrl Pts',(-13.1583919094726,-2.97427794178157,
-21.8694174771658)) ;
#57613=CARTESIAN_POINT('Ctrl Pts',(-13.1583867628863,-2.97432607736403,
-21.8694299862965)) ;
#57614=CARTESIAN_POINT('Ctrl Pts',(-13.1583816162999,-2.9743742129465,-21.8694424954271)) ;
#57615=CARTESIAN_POINT('Ctrl Pts',(-13.1582827830485,-2.97529859190629,
-21.8696827164154)) ;
#57616=CARTESIAN_POINT('Ctrl Pts',(-13.1590495899011,-2.98568101501634,
-21.8712515447568)) ;
#57617=CARTESIAN_POINT('Ctrl Pts',(-13.1673405936747,-3.09725857703815,
-21.8880811230034)) ;
#57618=CARTESIAN_POINT('Ctrl Pts',(-13.2225454665839,-3.7480304421894,-21.9821187438248)) ;
#57619=CARTESIAN_POINT('Ctrl Pts',(-13.4559147992043,-6.49920651633227,
-22.379675795358)) ;
#57620=CARTESIAN_POINT('Ctrl Pts',(-14.2193462265786,-15.3848234289498,
-23.6578464502457)) ;
#57621=CARTESIAN_POINT('Ctrl Pts',(-14.2895993929987,-16.2025431677231,
-23.7754751494418)) ;
#57622=CARTESIAN_POINT('',(-8.14947771652619,-2.97427793741671,-24.1867879501258)) ;
#57623=CARTESIAN_POINT('Origin',(-5.46365993374796E-16,-2.97427793741672,
0.)) ;
#57624=CARTESIAN_POINT('',(-8.8698743394829,-16.2025431678319,-26.2829069662568)) ;
#57625=CARTESIAN_POINT('Ctrl Pts',(-8.8698743394858,-16.2025431678319,-26.2829069662558)) ;
#57626=CARTESIAN_POINT('Ctrl Pts',(-8.8690475992033,-16.1872381291413,-26.2804794906608)) ;
#57627=CARTESIAN_POINT('Ctrl Pts',(-8.8682209482893,-16.1719348447295,-26.2780522951228)) ;
#57628=CARTESIAN_POINT('Ctrl Pts',(-8.75369775126741,-14.0518506209721,
-25.9417940804283)) ;
#57629=CARTESIAN_POINT('Ctrl Pts',(-8.62455882373438,-11.6630949877703,
-25.5629575129557)) ;
#57630=CARTESIAN_POINT('Ctrl Pts',(-8.49788878968684,-9.32575037810072,
-25.1923789033979)) ;
#57631=CARTESIAN_POINT('Ctrl Pts',(-8.41856649585192,-7.8609282885068,-24.9601150006645)) ;
#57632=CARTESIAN_POINT('Ctrl Pts',(-8.28260316417309,-5.36388181533702,
-24.5644312808462)) ;
#57633=CARTESIAN_POINT('Ctrl Pts',(-8.22698003060744,-4.34594047322709,
-24.4031938195724)) ;
#57634=CARTESIAN_POINT('Ctrl Pts',(-8.17315345603937,-3.37573518238573,
-24.2497910871311)) ;
#57635=CARTESIAN_POINT('Ctrl Pts',(-8.16013095169145,-3.14458998608287,
-24.213310806901)) ;
#57636=CARTESIAN_POINT('Ctrl Pts',(-8.15322417016401,-3.02954094887778,
-24.1952965060488)) ;
#57637=CARTESIAN_POINT('Ctrl Pts',(-8.15251766614579,-3.01790731126877,
-24.1934776472756)) ;
#57638=CARTESIAN_POINT('Ctrl Pts',(-8.15150361548596,-3.00173213555065,
-24.1909594376427)) ;
#57639=CARTESIAN_POINT('Ctrl Pts',(-8.15108302267982,-2.99513137012668,
-24.1899340908212)) ;
#57640=CARTESIAN_POINT('Ctrl Pts',(-8.15049249698612,-2.98633283447704,
-24.1885774200603)) ;
#57641=CARTESIAN_POINT('Ctrl Pts',(-8.15007714725426,-2.98023825569031,
-24.1876398039442)) ;
#57642=CARTESIAN_POINT('Ctrl Pts',(-8.14968298797736,-2.97566568479222,
-24.1869641494673)) ;
#57643=CARTESIAN_POINT('Ctrl Pts',(-8.1495760041458,-2.97458686961963,-24.1868094545128)) ;
#57644=CARTESIAN_POINT('Ctrl Pts',(-8.14950796797829,-2.97437302247926,
-24.1867945689326)) ;
#57645=CARTESIAN_POINT('Ctrl Pts',(-8.14949284226742,-2.97432548027622,
-24.1867912595821)) ;
#57646=CARTESIAN_POINT('Ctrl Pts',(-8.14947771655654,-2.97427793807318,
-24.1867879502316)) ;
#57647=CARTESIAN_POINT('',(-8.84449214097162,-16.2025431678319,-26.2914592246877)) ;
#57648=CARTESIAN_POINT('Origin',(0.286549277334558,-21.5586464785791,0.850447948841961)) ;
#57649=CARTESIAN_POINT('Ctrl Pts',(-8.14947771655655,-2.97427793807318,
-24.1867879502316)) ;
#57650=CARTESIAN_POINT('Ctrl Pts',(-8.14946923078658,-2.97432589067353,
-24.1867992877722)) ;
#57651=CARTESIAN_POINT('Ctrl Pts',(-8.14946074501662,-2.97437384327389,
-24.1868106253128)) ;
#57652=CARTESIAN_POINT('Ctrl Pts',(-8.14929875494501,-2.97528923989621,
-24.1870270545849)) ;
#57653=CARTESIAN_POINT('Ctrl Pts',(-8.14979835399925,-2.98748257149445,
-24.1890145855308)) ;
#57654=CARTESIAN_POINT('Ctrl Pts',(-8.15269430516147,-3.05983243148465,
-24.2008307822515)) ;
#57655=CARTESIAN_POINT('Ctrl Pts',(-8.16894924936113,-3.37814059840374,
-24.2516329420915)) ;
#57656=CARTESIAN_POINT('Ctrl Pts',(-8.24032645255946,-4.7768625642409,-24.4748868920346)) ;
#57657=CARTESIAN_POINT('Ctrl Pts',(-8.4957008254956,-9.61051691549516,-25.243464810217)) ;
#57658=CARTESIAN_POINT('Ctrl Pts',(-8.62394445730424,-12.0381139511629,
-25.6294704668798)) ;
#57659=CARTESIAN_POINT('Ctrl Pts',(-8.7398048631378,-14.2266206439564,-25.9773756898256)) ;
#57660=CARTESIAN_POINT('Ctrl Pts',(-8.84449214096946,-16.2025431678314,
-26.2914592246884)) ;
#57661=CARTESIAN_POINT('',(-2.75950295924795,-2.97427793707758,-25.3732111056427)) ;
#57662=CARTESIAN_POINT('Origin',(-5.46365993374796E-16,-2.97427793741672,
0.)) ;
#57663=CARTESIAN_POINT('',(-3.01245352594241,-16.2025431678319,-27.5751879984373)) ;
#57664=CARTESIAN_POINT('Ctrl Pts',(-3.01245352594352,-16.2025431678319,
-27.5751879984372)) ;
#57665=CARTESIAN_POINT('Ctrl Pts',(-3.01213020923632,-16.185215473181,-27.5723027580066)) ;
#57666=CARTESIAN_POINT('Ctrl Pts',(-3.01180686736354,-16.1678868184851,
-27.5694173585072)) ;
#57667=CARTESIAN_POINT('Ctrl Pts',(-2.97221120494068,-14.0459096503381,
-27.2160863999648)) ;
#57668=CARTESIAN_POINT('Ctrl Pts',(-2.92752542896347,-11.6569178583153,
-26.8183064787745)) ;
#57669=CARTESIAN_POINT('Ctrl Pts',(-2.88348538207021,-9.31987893564895,
-26.4292124476807)) ;
#57670=CARTESIAN_POINT('Ctrl Pts',(-2.85597258225044,-7.85641330793526,
-26.1855526842642)) ;
#57671=CARTESIAN_POINT('Ctrl Pts',(-2.80828475893858,-5.36133051516146,
-25.7702187256031)) ;
#57672=CARTESIAN_POINT('Ctrl Pts',(-2.78863406182219,-4.34397548551647,
-25.6008912291156)) ;
#57673=CARTESIAN_POINT('Ctrl Pts',(-2.76906671893031,-3.37503715205337,
-25.4397147951663)) ;
#57674=CARTESIAN_POINT('Ctrl Pts',(-2.76420013559178,-3.14436060318559,
-25.4013659265098)) ;
#57675=CARTESIAN_POINT('Ctrl Pts',(-2.76133149427244,-3.02949078756967,
-25.3823177938562)) ;
#57676=CARTESIAN_POINT('Ctrl Pts',(-2.76103271954395,-3.0178669010488,-25.3803912020351)) ;
#57677=CARTESIAN_POINT('Ctrl Pts',(-2.76058392755013,-3.00170195861387,
-25.3777155776922)) ;
#57678=CARTESIAN_POINT('Ctrl Pts',(-2.76039352479921,-2.9951002807134,-25.3766236408899)) ;
#57679=CARTESIAN_POINT('Ctrl Pts',(-2.76010875449308,-2.98631499743371,
-25.3751739431355)) ;
#57680=CARTESIAN_POINT('Ctrl Pts',(-2.75990408935368,-2.98020400131968,
-25.3741662567881)) ;
#57681=CARTESIAN_POINT('Ctrl Pts',(-2.75966514631604,-2.97566119972773,
-25.373426601311)) ;
#57682=CARTESIAN_POINT('Ctrl Pts',(-2.75959564554254,-2.97461343441426,
-25.3732575699952)) ;
#57683=CARTESIAN_POINT('Ctrl Pts',(-2.75952938647569,-2.97437348082648,
-25.3732243344283)) ;
#57684=CARTESIAN_POINT('Ctrl Pts',(-2.75951619495104,-2.97432570844283,
-25.3732177175531)) ;
#57685=CARTESIAN_POINT('Ctrl Pts',(-2.75950300342517,-2.97427793606106,
-25.3732111006667)) ;
#57686=CARTESIAN_POINT('',(-2.98582626636701,-16.2025431678319,-27.5780838874313)) ;
#57687=CARTESIAN_POINT('Origin',(0.0970287445296876,-21.5586464785792,0.892164572691307)) ;
#57688=CARTESIAN_POINT('Ctrl Pts',(-2.75950291268683,-2.97427793673757,
-25.3732111106492)) ;
#57689=CARTESIAN_POINT('Ctrl Pts',(-2.75949693136208,-2.97432677662352,
-25.3732199926138)) ;
#57690=CARTESIAN_POINT('Ctrl Pts',(-2.75949095003733,-2.97437561650947,
-25.3732288745783)) ;
#57691=CARTESIAN_POINT('Ctrl Pts',(-2.75892375064498,-2.97900702423292,
-25.3740711369728)) ;
#57692=CARTESIAN_POINT('Ctrl Pts',(-2.75932604494419,-2.98364704831612,
-25.3748094127723)) ;
#57693=CARTESIAN_POINT('Ctrl Pts',(-2.75952661218359,-3.04515584041083,
-25.3851542688191)) ;
#57694=CARTESIAN_POINT('Ctrl Pts',(-2.76315465789757,-3.28410263517818,
-25.4250316993994)) ;
#57695=CARTESIAN_POINT('Ctrl Pts',(-2.78251290289041,-4.56104030220253,
-25.6381409650497)) ;
#57696=CARTESIAN_POINT('Ctrl Pts',(-2.86857365834589,-9.50103938481345,
-26.4613669104021)) ;
#57697=CARTESIAN_POINT('Ctrl Pts',(-2.91138738464896,-11.9608037313374,
-26.8712784094001)) ;
#57698=CARTESIAN_POINT('Ctrl Pts',(-2.95055606709738,-14.1953706426329,
-27.2436316384425)) ;
#57699=CARTESIAN_POINT('Ctrl Pts',(-2.98582626636797,-16.2025431678314,
-27.5780838874311)) ;
#57700=CARTESIAN_POINT('Origin',(-5.46365993374796E-16,-2.97427793741672,
0.)) ;
#57701=CARTESIAN_POINT('',(26.7317316862594,-16.2025431678319,7.40813002376185)) ;
#57702=CARTESIAN_POINT('Ctrl Pts',(26.7317316862594,-16.2025431678314,7.40813002376151)) ;
#57703=CARTESIAN_POINT('Ctrl Pts',(26.6708612250771,-15.8258476727767,7.39144313065645)) ;
#57704=CARTESIAN_POINT('Ctrl Pts',(26.6087613235262,-15.4415494924405,7.37442275828496)) ;
#57705=CARTESIAN_POINT('Ctrl Pts',(26.3177228462478,-13.6405242351605,7.29467562226099)) ;
#57706=CARTESIAN_POINT('Ctrl Pts',(26.0771464558663,-12.1518647220656,7.22881355838971)) ;
#57707=CARTESIAN_POINT('Ctrl Pts',(25.792202821699,-10.3888908916882,7.15094619732042)) ;
#57708=CARTESIAN_POINT('Ctrl Pts',(25.7373039946257,-10.0492376710507,7.13595081080411)) ;
#57709=CARTESIAN_POINT('Ctrl Pts',(25.6751992047838,-9.66501669817754,7.11899639910692)) ;
#57710=CARTESIAN_POINT('Ctrl Pts',(25.6670200785919,-9.61441555997111,7.11676371273239)) ;
#57711=CARTESIAN_POINT('Ctrl Pts',(25.655407176928,-9.54257140038981,7.11359397120237)) ;
#57712=CARTESIAN_POINT('Ctrl Pts',(25.6520195340659,-9.52161349076768,7.11266932544962)) ;
#57713=CARTESIAN_POINT('Ctrl Pts',(25.5946244020356,-9.16653613429363,7.09700475867469)) ;
#57714=CARTESIAN_POINT('Ctrl Pts',(25.4026983078924,-7.97911008179591,7.04458112870836)) ;
#57715=CARTESIAN_POINT('Ctrl Pts',(25.0403950796436,-5.73851073762623,6.94620342034088)) ;
#57716=CARTESIAN_POINT('Ctrl Pts',(24.876091691589,-4.72268532357717,6.90176444040087)) ;
#57717=CARTESIAN_POINT('Ctrl Pts',(24.6906989359728,-3.57769528729753,6.85238733933921)) ;
#57718=CARTESIAN_POINT('Ctrl Pts',(24.6384207630783,-3.25519700220501,6.83869725874935)) ;
#57719=CARTESIAN_POINT('Ctrl Pts',(24.6073454773866,-3.06433572454096,6.83108487113129)) ;
#57720=CARTESIAN_POINT('Ctrl Pts',(24.6038284005659,-3.04276136762821,6.83024032654945)) ;
#57721=CARTESIAN_POINT('Ctrl Pts',(24.5986470322512,-3.01110082456801,6.82907309089495)) ;
#57722=CARTESIAN_POINT('Ctrl Pts',(24.5972152123349,-3.00236268573874,6.8287573880774)) ;
#57723=CARTESIAN_POINT('Ctrl Pts',(24.5949512353083,-2.9886302619033,6.82831094889558)) ;
#57724=CARTESIAN_POINT('Ctrl Pts',(24.5937055045486,-2.98105415711827,6.82805278954538)) ;
#57725=CARTESIAN_POINT('Ctrl Pts',(24.5927170642124,-2.9753008951146,6.82800959104032)) ;
#57726=CARTESIAN_POINT('Ctrl Pts',(24.5926019604562,-2.97464733466745,6.82801483559427)) ;
#57727=CARTESIAN_POINT('Ctrl Pts',(24.5925339353042,-2.9742779365593,6.82802848779065)) ;
#57728=CARTESIAN_POINT('',(26.724566134977,-16.2025431678319,7.43393800702995)) ;
#57729=CARTESIAN_POINT('Origin',(-0.864714158790687,-21.5586464785792,-0.240086704374448)) ;
#57730=CARTESIAN_POINT('Ctrl Pts',(24.5925339349735,-2.97427793447466,6.82802848788166)) ;
#57731=CARTESIAN_POINT('Ctrl Pts',(24.5922903959867,-2.97295544059358,6.82807736481932)) ;
#57732=CARTESIAN_POINT('Ctrl Pts',(24.5926502825679,-2.97527517096814,6.8282340058834)) ;
#57733=CARTESIAN_POINT('Ctrl Pts',(24.5947125268534,-2.98908868346097,6.8294578061479)) ;
#57734=CARTESIAN_POINT('Ctrl Pts',(24.5969055942541,-3.00247119052961,6.82994048762188)) ;
#57735=CARTESIAN_POINT('Ctrl Pts',(24.6100866411951,-3.08518510694711,6.834269953955)) ;
#57736=CARTESIAN_POINT('Ctrl Pts',(24.6266891374417,-3.18867973050429,6.83929132521917)) ;
#57737=CARTESIAN_POINT('Ctrl Pts',(24.6520865382055,-3.34683414658513,6.84686946441176)) ;
#57738=CARTESIAN_POINT('Ctrl Pts',(24.6617947563325,-3.40723155602974,6.84973021442313)) ;
#57739=CARTESIAN_POINT('Ctrl Pts',(24.6690099532311,-3.45211719949212,6.85185507493831)) ;
#57740=CARTESIAN_POINT('Ctrl Pts',(24.6704849089357,-3.46129178275174,6.85228875962351)) ;
#57741=CARTESIAN_POINT('Ctrl Pts',(24.8262885492609,-4.43038592304249,6.89807351378244)) ;
#57742=CARTESIAN_POINT('Ctrl Pts',(25.2411322159244,-7.00390438792483,7.01572324021616)) ;
#57743=CARTESIAN_POINT('Ctrl Pts',(25.621524497974,-9.36314461801283,7.12325426676193)) ;
#57744=CARTESIAN_POINT('Ctrl Pts',(25.7085353751157,-9.90272468153527,7.14780567066282)) ;
#57745=CARTESIAN_POINT('Ctrl Pts',(25.7365170082255,-10.0762492014801,7.15570246432779)) ;
#57746=CARTESIAN_POINT('Ctrl Pts',(25.7399002083209,-10.0972296242141,7.15665721132822)) ;
#57747=CARTESIAN_POINT('Ctrl Pts',(26.0610066170549,-12.0885198967075,7.24727146087783)) ;
#57748=CARTESIAN_POINT('Ctrl Pts',(26.409490678682,-14.249170043393,7.3453495476889)) ;
#57749=CARTESIAN_POINT('Ctrl Pts',(26.7245661349771,-16.2025431678314,7.43393800702949)) ;
#57750=CARTESIAN_POINT('',(5.97619665355046,-16.2025431678319,27.0878375466411)) ;
#57751=CARTESIAN_POINT('Ctrl Pts',(5.97619665355081,-16.2025431678314,27.0878375466409)) ;
#57752=CARTESIAN_POINT('Ctrl Pts',(5.96072272453984,-15.779208956766,27.0186152627304)) ;
#57753=CARTESIAN_POINT('Ctrl Pts',(5.94488045825097,-15.3459135704608,26.9477650900312)) ;
#57754=CARTESIAN_POINT('Ctrl Pts',(5.89489453658278,-13.9792379428408,26.7242972853165)) ;
#57755=CARTESIAN_POINT('Ctrl Pts',(5.85987132786771,-13.0223166999358,26.5678345002262)) ;
#57756=CARTESIAN_POINT('Ctrl Pts',(5.80809434291493,-11.6092032550686,26.3367939418112)) ;
#57757=CARTESIAN_POINT('Ctrl Pts',(5.79109467281383,-11.1454992507822,26.2609815488546)) ;
#57758=CARTESIAN_POINT('Ctrl Pts',(5.76604719586049,-10.4627424983602,26.149359334853)) ;
#57759=CARTESIAN_POINT('Ctrl Pts',(5.75780507218401,-10.2381528735791,26.1126423647602)) ;
#57760=CARTESIAN_POINT('Ctrl Pts',(5.74405261756366,-9.86355741108647,26.0514029061754)) ;
#57761=CARTESIAN_POINT('Ctrl Pts',(5.73849711874685,-9.71227520462928,26.0266713826372)) ;
#57762=CARTESIAN_POINT('Ctrl Pts',(5.73219963076735,-9.54083766529388,25.9986452802693)) ;
#57763=CARTESIAN_POINT('Ctrl Pts',(5.73142304793564,-9.51969691584835,25.9951892553716)) ;
#57764=CARTESIAN_POINT('Ctrl Pts',(5.71641614781068,-9.11120429329879,25.9284104333817)) ;
#57765=CARTESIAN_POINT('Ctrl Pts',(5.65974887270405,-7.56784943123937,25.6761017421969)) ;
#57766=CARTESIAN_POINT('Ctrl Pts',(5.57709597367415,-5.33563589821568,25.3113304772533)) ;
#57767=CARTESIAN_POINT('Ctrl Pts',(5.54998071858407,-4.60671916329358,25.1922440851709)) ;
#57768=CARTESIAN_POINT('Ctrl Pts',(5.51727804656527,-3.73938880523472,25.0506409639444)) ;
#57769=CARTESIAN_POINT('Ctrl Pts',(5.50753615464755,-3.48384628708339,25.0089437563574)) ;
#57770=CARTESIAN_POINT('Ctrl Pts',(5.49667474050161,-3.20573594642881,24.9636211780588)) ;
#57771=CARTESIAN_POINT('Ctrl Pts',(5.49367323791136,-3.13044865534939,24.9513653690511)) ;
#57772=CARTESIAN_POINT('Ctrl Pts',(5.49016340863078,-3.04571930373455,24.9376015459661)) ;
#57773=CARTESIAN_POINT('Ctrl Pts',(5.48924355592997,-3.02334616904155,24.9339656258311)) ;
#57774=CARTESIAN_POINT('Ctrl Pts',(5.48776174140018,-2.9921585742524,24.9289411704213)) ;
#57775=CARTESIAN_POINT('Ctrl Pts',(5.48756020827974,-2.98773607317881,24.9282267950638)) ;
#57776=CARTESIAN_POINT('Ctrl Pts',(5.48695179424486,-2.97700394873062,24.9265194850504)) ;
#57777=CARTESIAN_POINT('Ctrl Pts',(5.48680471756041,-2.97502954371886,24.9262131248547)) ;
#57778=CARTESIAN_POINT('Ctrl Pts',(5.48671463550852,-2.97427793387919,24.9261040052127)) ;
#57779=CARTESIAN_POINT('',(5.95003858478611,-16.2025431678319,27.0935953729785)) ;
#57780=CARTESIAN_POINT('Origin',(-0.192919915744,-21.5586464785792,-0.876444013123365)) ;
#57781=CARTESIAN_POINT('Ctrl Pts',(5.48671463550852,-2.97427793387919,24.9261040052127)) ;
#57782=CARTESIAN_POINT('Ctrl Pts',(5.48655343436942,-2.97293293385127,24.9259087364526)) ;
#57783=CARTESIAN_POINT('Ctrl Pts',(5.48657474615765,-2.97550366968052,24.9263450877106)) ;
#57784=CARTESIAN_POINT('Ctrl Pts',(5.48650656002357,-2.98896306265492,24.9286692261902)) ;
#57785=CARTESIAN_POINT('Ctrl Pts',(5.4870581876998,-3.00225028492091,24.9308273952644)) ;
#57786=CARTESIAN_POINT('Ctrl Pts',(5.48940856559024,-3.08513378934106,24.9445297544016)) ;
#57787=CARTESIAN_POINT('Ctrl Pts',(5.49278640846088,-3.18963983843306,24.9617155731815)) ;
#57788=CARTESIAN_POINT('Ctrl Pts',(5.49706224508616,-3.31975443705721,24.9830972000661)) ;
#57789=CARTESIAN_POINT('Ctrl Pts',(5.49838046279082,-3.35939593234685,24.9896080397158)) ;
#57790=CARTESIAN_POINT('Ctrl Pts',(5.49982593417466,-3.4027865871652,24.996734084582)) ;
#57791=CARTESIAN_POINT('Ctrl Pts',(5.50011019121751,-3.41129002097857,24.9981303867991)) ;
#57792=CARTESIAN_POINT('Ctrl Pts',(5.53157664010535,-4.35245512534218,25.1526729085225)) ;
#57793=CARTESIAN_POINT('Ctrl Pts',(5.6231120523299,-6.95923681319167,25.5797509022431)) ;
#57794=CARTESIAN_POINT('Ctrl Pts',(5.70685056811174,-9.33462644072451,25.9688468798497)) ;
#57795=CARTESIAN_POINT('Ctrl Pts',(5.72594006926732,-9.87490507692204,26.0573366155415)) ;
#57796=CARTESIAN_POINT('Ctrl Pts',(5.73156501003844,-10.0341421448734,26.0834176111344)) ;
#57797=CARTESIAN_POINT('Ctrl Pts',(5.7322996806034,-10.054939175098,26.0868238922277)) ;
#57798=CARTESIAN_POINT('Ctrl Pts',(5.80304552537078,-12.0575349767993,26.4148222638508)) ;
#57799=CARTESIAN_POINT('Ctrl Pts',(5.88027610174045,-14.2365603955804,26.7716619766563)) ;
#57800=CARTESIAN_POINT('Ctrl Pts',(5.9500385847868,-16.2025431678314,27.0935953729783)) ;
#57801=CARTESIAN_POINT('Origin',(-3.29835915403229E-15,-17.9554309391014,
0.)) ;
#57802=CARTESIAN_POINT('',(0.494365359100647,-15.9320789705494,-29.3036235215755)) ;
#57803=CARTESIAN_POINT('',(0.492460255574504,-15.9108622559522,-29.3036555995867)) ;
#57804=CARTESIAN_POINT('Origin',(-3.92942532412469E-15,-21.3907951629292,
0.)) ;
#57805=CARTESIAN_POINT('',(5.81660547648255,-15.9320789705494,-28.7247950268312)) ;
#57806=CARTESIAN_POINT('Origin',(-3.92942532412469E-15,-21.3907951629292,
0.)) ;
#57807=CARTESIAN_POINT('',(5.81660547648253,-15.9320789705494,-28.7247950268311)) ;
#57808=CARTESIAN_POINT('',(6.78222025653935,-15.9320789748381,-28.5122470677388)) ;
#57809=CARTESIAN_POINT('',(6.7803665240703,-15.9108618774105,-28.5126880067314)) ;
#57810=CARTESIAN_POINT('Origin',(-3.92942532412469E-15,-21.3907951629292,
0.)) ;
#57811=CARTESIAN_POINT('',(11.8555982263102,-15.9320789748381,-26.8028269993353)) ;
#57812=CARTESIAN_POINT('Origin',(-3.92942532412469E-15,-21.3907951629292,
0.)) ;
#57813=CARTESIAN_POINT('',(11.8555981836618,-15.932078964213,-26.8028269424543)) ;
#57814=CARTESIAN_POINT('',(12.7529460606102,-15.932078986503,-26.3876695044702)) ;
#57815=CARTESIAN_POINT('',(12.7512304233236,-15.9108618549279,-26.3884982701394)) ;
#57816=CARTESIAN_POINT('Origin',(-3.92942532412469E-15,-21.3907951629292,
0.)) ;
#57817=CARTESIAN_POINT('',(17.3402362534815,-15.932078986503,-23.6275885730099)) ;
#57818=CARTESIAN_POINT('Origin',(-3.92942532412469E-15,-21.3907951629292,
0.)) ;
#57819=CARTESIAN_POINT('',(17.3402360849801,-15.9320789502307,-23.627588425548)) ;
#57820=CARTESIAN_POINT('',(18.1273581983811,-15.9320789854432,-23.0292340460187)) ;
#57821=CARTESIAN_POINT('',(18.1258608416401,-15.9108618569292,-23.0304122763961)) ;
#57822=CARTESIAN_POINT('Origin',(-3.92942532412468E-15,-21.3907951629292,
0.)) ;
#57823=CARTESIAN_POINT('',(22.0140643019504,-15.9320789854432,-19.3475504627412)) ;
#57824=CARTESIAN_POINT('Origin',(-3.92942532412468E-15,-21.3907951629292,
0.)) ;
#57825=CARTESIAN_POINT('',(22.0140641187248,-15.93207895158,-19.3475503621096)) ;
#57826=CARTESIAN_POINT('',(22.6541552108272,-15.9320789866943,-18.5939771612252)) ;
#57827=CARTESIAN_POINT('',(22.6529461354171,-15.9108618551723,-18.595449711334)) ;
#57828=CARTESIAN_POINT('Origin',(-3.92942532412469E-15,-21.3907951629292,
0.)) ;
#57829=CARTESIAN_POINT('',(25.6585391321031,-15.9320789866943,-14.1628423910863)) ;
#57830=CARTESIAN_POINT('Origin',(-3.92942532412469E-15,-21.3907951629292,
0.)) ;
#57831=CARTESIAN_POINT('',(25.6585389138341,-15.9320789500595,-14.1628423304031)) ;
#57832=CARTESIAN_POINT('',(26.1216692307926,-15.9320789708932,-13.2892868445522)) ;
#57833=CARTESIAN_POINT('',(26.1208051637602,-15.9108618761819,-13.290985048708)) ;
#57834=CARTESIAN_POINT('Origin',(-3.92942532412469E-15,-21.3907951629292,
0.)) ;
#57835=CARTESIAN_POINT('',(28.103249474609,-15.9320789708932,-8.31589545434586)) ;
#57836=CARTESIAN_POINT('Origin',(-3.92942532412469E-15,-21.3907951629292,
0.)) ;
#57837=CARTESIAN_POINT('',(28.1032494677604,-15.9320789699703,-8.31589545421927)) ;
#57838=CARTESIAN_POINT('',(28.3677629681468,-15.9320789705494,-7.36320397554968)) ;
#57839=CARTESIAN_POINT('',(28.3672842077332,-15.9108622559523,-7.3650482198151)) ;
#57840=CARTESIAN_POINT('Origin',(-3.9294253241247E-15,-21.3907951629292,
0.)) ;
#57841=CARTESIAN_POINT('',(29.2338828322227,-15.9320789705494,-2.08010652476853)) ;
#57842=CARTESIAN_POINT('Origin',(-3.9294253241247E-15,-21.3907951629292,
0.)) ;
#57843=CARTESIAN_POINT('',(29.2338828322227,-15.9320789705494,-2.08010652476853)) ;
#57844=CARTESIAN_POINT('',(29.287411634191,-15.9320789705494,-1.09282586534355)) ;
#57845=CARTESIAN_POINT('',(29.2873405249314,-15.9108622559522,-1.09472991153979)) ;
#57846=CARTESIAN_POINT('Origin',(-3.92942532412469E-15,-21.3907951629292,
0.)) ;
#57847=CARTESIAN_POINT('',(28.9975723124842,-15.9320789705494,4.25294587136481)) ;
#57848=CARTESIAN_POINT('Origin',(-3.92942532412469E-15,-21.3907951629292,
0.)) ;
#57849=CARTESIAN_POINT('',(28.9975723124842,-15.9320789705494,4.2529458713648)) ;
#57850=CARTESIAN_POINT('',(28.837613004449,-15.9320790002153,5.22865180923071)) ;
#57851=CARTESIAN_POINT('',(28.8379528519801,-15.9108618570888,5.22677686529081)) ;
#57852=CARTESIAN_POINT('Origin',(-3.9294253241247E-15,-21.3907951629292,
0.)) ;
#57853=CARTESIAN_POINT('',(27.4053672544904,-15.9320790002153,10.387134791801)) ;
#57854=CARTESIAN_POINT('Origin',(-3.9294253241247E-15,-21.3907951629292,
0.)) ;
#57855=CARTESIAN_POINT('',(27.4053669090694,-15.9320789327933,10.3871345576338)) ;
#57856=CARTESIAN_POINT('',(27.0394003853433,-15.932078979868,11.3056431141676)) ;
#57857=CARTESIAN_POINT('',(27.0401351051488,-15.9108618606822,11.3038851399891)) ;
#57858=CARTESIAN_POINT('Origin',(-3.92942532412469E-15,-21.3907951629292,
0.)) ;
#57859=CARTESIAN_POINT('',(24.531718174094,-15.932078979868,16.0356335344338)) ;
#57860=CARTESIAN_POINT('Origin',(-3.92942532412469E-15,-21.3907951629292,
0.)) ;
#57861=CARTESIAN_POINT('',(24.5317180654997,-15.9320789564852,16.0356334188635)) ;
#57862=CARTESIAN_POINT('',(23.9768550750891,-15.9320789856441,16.8539952692808)) ;
#57863=CARTESIAN_POINT('',(23.9779505086143,-15.9108618566337,16.8524363191949)) ;
#57864=CARTESIAN_POINT('Origin',(-3.92942532412468E-15,-21.3907951629292,
0.)) ;
#57865=CARTESIAN_POINT('',(20.5109930276199,-15.9320789856441,20.9343235106773)) ;
#57866=CARTESIAN_POINT('Origin',(-3.92942532412468E-15,-21.3907951629292,
0.)) ;
#57867=CARTESIAN_POINT('',(20.5109929157274,-15.9320789513242,20.9343233307748)) ;
#57868=CARTESIAN_POINT('',(19.7931787380933,-15.9320789860435,21.6142733149332)) ;
#57869=CARTESIAN_POINT('',(19.7945836826822,-15.910861856046,21.6129862941042)) ;
#57870=CARTESIAN_POINT('Origin',(-3.9294253241247E-15,-21.3907951629292,
0.)) ;
#57871=CARTESIAN_POINT('',(15.5311966688983,-15.9320789860435,24.8541478534821)) ;
#57872=CARTESIAN_POINT('Origin',(-3.9294253241247E-15,-21.3907951629292,
0.)) ;
#57873=CARTESIAN_POINT('',(15.5311965964273,-15.9320789508155,24.8541476484462)) ;
#57874=CARTESIAN_POINT('',(14.6839955520831,-15.9320789746107,25.3638920378233)) ;
#57875=CARTESIAN_POINT('',(14.6856444121027,-15.9108618692113,25.3629372329525)) ;
#57876=CARTESIAN_POINT('Origin',(-3.92942532412469E-15,-21.3907951629292,
0.)) ;
#57877=CARTESIAN_POINT('',(9.82517875536679,-15.9320789746107,27.6118200614346)) ;
#57878=CARTESIAN_POINT('Origin',(-3.92942532412469E-15,-21.3907951629292,
0.)) ;
#57879=CARTESIAN_POINT('',(9.82517874764536,-15.9320789645514,27.61181999456)) ;
#57880=CARTESIAN_POINT('',(8.88820398548747,-15.9320790345093,27.9275227055374)) ;
#57881=CARTESIAN_POINT('',(8.89001959178239,-15.9108618212313,27.9269444452518)) ;
#57882=CARTESIAN_POINT('Origin',(-3.9294253241247E-15,-21.3907951629292,
0.)) ;
#57883=CARTESIAN_POINT('',(3.65974695538204,-15.9320790345093,29.078393125799)) ;
#57884=CARTESIAN_POINT('Origin',(-3.9294253241247E-15,-21.3907951629292,
0.)) ;
#57885=CARTESIAN_POINT('',(3.65974705260781,-15.9320788891238,29.0783922312664)) ;
#57886=CARTESIAN_POINT('',(2.6768116432333,-15.9320789705494,29.1852947223283)) ;
#57887=CARTESIAN_POINT('',(2.67870904720401,-15.9108622559523,29.1851206343735)) ;
#57888=CARTESIAN_POINT('Origin',(-3.92942532412468E-15,-21.3907951629292,
0.)) ;
#57889=CARTESIAN_POINT('',(-2.6768116432333,-15.9320789705494,29.1852947223283)) ;
#57890=CARTESIAN_POINT('Origin',(-3.92942532412468E-15,-21.3907951629292,
0.)) ;
#57891=CARTESIAN_POINT('',(-2.67681164323326,-15.9320789705494,29.1852947223282)) ;
#57892=CARTESIAN_POINT('',(-3.65974695538209,-15.9320790345093,29.078393125799)) ;
#57893=CARTESIAN_POINT('',(-3.65785635054521,-15.9108618212313,29.0786306642735)) ;
#57894=CARTESIAN_POINT('Origin',(-3.9294253241247E-15,-21.3907951629292,
0.)) ;
#57895=CARTESIAN_POINT('',(-8.88820398548748,-15.9320790345093,27.9275227055374)) ;
#57896=CARTESIAN_POINT('Origin',(-3.9294253241247E-15,-21.3907951629292,
0.)) ;
#57897=CARTESIAN_POINT('',(-8.88820352164328,-15.9320788891238,27.9275219345056)) ;
#57898=CARTESIAN_POINT('',(-9.8251787553669,-15.9320789746107,27.6118200614345)) ;
#57899=CARTESIAN_POINT('',(-9.82338358996211,-15.9108618692113,27.6124586323977)) ;
#57900=CARTESIAN_POINT('Origin',(-3.92942532412469E-15,-21.3907951629292,
0.)) ;
#57901=CARTESIAN_POINT('',(-14.6839955520832,-15.9320789746107,25.3638920378232)) ;
#57902=CARTESIAN_POINT('Origin',(-3.92942532412469E-15,-21.3907951629292,
0.)) ;
#57903=CARTESIAN_POINT('',(-14.6839955061126,-15.9320789645514,25.3638919886445)) ;
#57904=CARTESIAN_POINT('',(-15.5311966688983,-15.9320789860435,24.8541478534821)) ;
#57905=CARTESIAN_POINT('',(-15.5295806974965,-15.9108618560459,24.8551572732861)) ;
#57906=CARTESIAN_POINT('Origin',(-3.9294253241247E-15,-21.3907951629292,
0.)) ;
#57907=CARTESIAN_POINT('',(-19.7931787380933,-15.9320789860435,21.6142733149332)) ;
#57908=CARTESIAN_POINT('Origin',(-3.9294253241247E-15,-21.3907951629292,
0.)) ;
#57909=CARTESIAN_POINT('',(-19.7931785599191,-15.9320789508155,21.6142731902508)) ;
#57910=CARTESIAN_POINT('',(-20.5109930276199,-15.9320789856441,20.9343235106773)) ;
#57911=CARTESIAN_POINT('',(-20.5096318357506,-15.9108618566336,20.935656723591)) ;
#57912=CARTESIAN_POINT('Origin',(-3.92942532412468E-15,-21.3907951629292,
0.)) ;
#57913=CARTESIAN_POINT('',(-23.9768550750892,-15.9320789856441,16.8539952692808)) ;
#57914=CARTESIAN_POINT('Origin',(-3.92942532412468E-15,-21.3907951629292,
0.)) ;
#57915=CARTESIAN_POINT('',(-23.9768548794545,-15.9320789513242,16.8539951879673)) ;
#57916=CARTESIAN_POINT('',(-24.531718174094,-15.932078979868,16.0356335344337)) ;
#57917=CARTESIAN_POINT('',(-24.5306754334589,-15.9108618606822,16.0372282063037)) ;
#57918=CARTESIAN_POINT('Origin',(-3.92942532412469E-15,-21.3907951629292,
0.)) ;
#57919=CARTESIAN_POINT('',(-27.0394003853434,-15.932078979868,11.3056431141676)) ;
#57920=CARTESIAN_POINT('Origin',(-3.92942532412469E-15,-21.3907951629292,
0.)) ;
#57921=CARTESIAN_POINT('',(-27.0394002287454,-15.9320789564852,11.3056430891418)) ;
#57922=CARTESIAN_POINT('',(-27.4053672544904,-15.9320790002153,10.387134791801)) ;
#57923=CARTESIAN_POINT('',(-27.404691820706,-15.9108618570887,10.3889165606763)) ;
#57924=CARTESIAN_POINT('Origin',(-3.92942532412469E-15,-21.3907951629292,
0.)) ;
#57925=CARTESIAN_POINT('',(-28.837613004449,-15.9320790002153,5.22865180923068)) ;
#57926=CARTESIAN_POINT('Origin',(-3.92942532412469E-15,-21.3907951629292,
0.)) ;
#57927=CARTESIAN_POINT('',(-28.8376125877467,-15.9320789327933,5.22865183179534)) ;
#57928=CARTESIAN_POINT('',(-28.9975723124843,-15.9320789705494,4.25294587136478)) ;
#57929=CARTESIAN_POINT('',(-28.9972957564644,-15.9108622559522,4.25483106769728)) ;
#57930=CARTESIAN_POINT('Origin',(-3.92942532412469E-15,-21.3907951629292,
0.)) ;
#57931=CARTESIAN_POINT('',(-29.287411634191,-15.9320789705494,-1.09282586534359)) ;
#57932=CARTESIAN_POINT('Origin',(-3.92942532412469E-15,-21.3907951629292,
0.)) ;
#57933=CARTESIAN_POINT('',(-29.287411634191,-15.9320789705494,-1.09282586534359)) ;
#57934=CARTESIAN_POINT('',(-29.2338828322227,-15.9320789705494,-2.08010652476856)) ;
#57935=CARTESIAN_POINT('',(-29.2340180034144,-15.9108622559522,-2.07820595190936)) ;
#57936=CARTESIAN_POINT('Origin',(-3.9294253241247E-15,-21.3907951629292,
0.)) ;
#57937=CARTESIAN_POINT('',(-28.3677629681468,-15.9320789705494,-7.36320397554972)) ;
#57938=CARTESIAN_POINT('Origin',(-3.9294253241247E-15,-21.3907951629292,
0.)) ;
#57939=CARTESIAN_POINT('',(-28.3677629681468,-15.9320789705494,-7.3632039755497)) ;
#57940=CARTESIAN_POINT('',(-28.103249474609,-15.9320789708932,-8.31589545434591)) ;
#57941=CARTESIAN_POINT('',(-28.1037900199178,-15.9108618761818,-8.31406834735388)) ;
#57942=CARTESIAN_POINT('Origin',(-3.92942532412469E-15,-21.3907951629292,
0.)) ;
#57943=CARTESIAN_POINT('',(-26.1216692307926,-15.9320789708932,-13.2892868445522)) ;
#57944=CARTESIAN_POINT('Origin',(-3.92942532412469E-15,-21.3907951629292,
0.)) ;
#57945=CARTESIAN_POINT('',(-26.1216692257335,-15.9320789699703,-13.2892868399344)) ;
#57946=CARTESIAN_POINT('',(-25.658539132103,-15.9320789866943,-14.1628423910863)) ;
#57947=CARTESIAN_POINT('',(-25.6594595719309,-15.9108618551722,-14.161174141197)) ;
#57948=CARTESIAN_POINT('Origin',(-3.92942532412469E-15,-21.3907951629292,
0.)) ;
#57949=CARTESIAN_POINT('',(-22.6541552108272,-15.9320789866943,-18.5939771612253)) ;
#57950=CARTESIAN_POINT('Origin',(-3.92942532412469E-15,-21.3907951629292,
0.)) ;
#57951=CARTESIAN_POINT('',(-22.6541550736643,-15.9320789500595,-18.5939769809197)) ;
#57952=CARTESIAN_POINT('',(-22.0140643019503,-15.9320789854432,-19.3475504627413)) ;
#57953=CARTESIAN_POINT('',(-22.0153218696111,-15.9108618569291,-19.3461190901096)) ;
#57954=CARTESIAN_POINT('Origin',(-3.92942532412468E-15,-21.3907951629291,
0.)) ;
#57955=CARTESIAN_POINT('',(-18.1273581983811,-15.9320789854432,-23.0292340460188)) ;
#57956=CARTESIAN_POINT('Origin',(-3.92942532412468E-15,-21.3907951629291,
0.)) ;
#57957=CARTESIAN_POINT('',(-18.1273581078167,-15.93207895158,-23.0292338576138)) ;
#57958=CARTESIAN_POINT('',(-17.3402362534815,-15.932078986503,-23.6275885730099)) ;
#57959=CARTESIAN_POINT('',(-17.3417720969185,-15.9108618549278,-23.6264609876381)) ;
#57960=CARTESIAN_POINT('Origin',(-3.92942532412468E-15,-21.3907951629292,
0.)) ;
#57961=CARTESIAN_POINT('',(-12.7529460606102,-15.932078986503,-26.3876695044702)) ;
#57962=CARTESIAN_POINT('Origin',(-3.92942532412468E-15,-21.3907951629292,
0.)) ;
#57963=CARTESIAN_POINT('',(-12.7529460092534,-15.9320789502307,-26.3876692865248)) ;
#57964=CARTESIAN_POINT('',(-11.8555982263102,-15.9320789748381,-26.8028269993354)) ;
#57965=CARTESIAN_POINT('',(-11.8573408147833,-15.9108618774106,-26.8020561967176)) ;
#57966=CARTESIAN_POINT('Origin',(-3.92942532412469E-15,-21.3907951629292,
0.)) ;
#57967=CARTESIAN_POINT('',(-6.78222025653932,-15.9320789748381,-28.5122470677388)) ;
#57968=CARTESIAN_POINT('Origin',(-3.92942532412469E-15,-21.3907951629292,
0.)) ;
#57969=CARTESIAN_POINT('',(-6.78222025606846,-15.932078964213,-28.5122469966465)) ;
#57970=CARTESIAN_POINT('',(-5.81660547648251,-15.9320789705494,-28.7247950268312)) ;
#57971=CARTESIAN_POINT('',(-5.8184729355711,-15.9108622559522,-28.7244168139326)) ;
#57972=CARTESIAN_POINT('Origin',(-3.9294253241247E-15,-21.3907951629292,
0.)) ;
#57973=CARTESIAN_POINT('',(-0.494365359100612,-15.9320789705494,-29.3036235215755)) ;
#57974=CARTESIAN_POINT('Origin',(-3.9294253241247E-15,-21.3907951629292,
0.)) ;
#57975=CARTESIAN_POINT('',(-0.494365359100623,-15.9320789705494,-29.3036235215755)) ;
#57976=CARTESIAN_POINT('',(-1.87947417050994E-15,-20.,-29.3077933083081)) ;
#57977=CARTESIAN_POINT('',(-8.68211344379605E-15,-17.9554309391014,-29.3077933083081)) ;
#57978=CARTESIAN_POINT('Origin',(-3.67394039744206E-15,-20.,0.)) ;
#57979=CARTESIAN_POINT('Origin',(-1.4236519040088E-15,-7.75,0.)) ;
#57980=CARTESIAN_POINT('',(1.88995598193963E-15,1.11022302462516E-15,-30.8653235080594)) ;
#57981=CARTESIAN_POINT('Origin',(-3.47179281571763E-31,-1.88995598193962E-15,
0.)) ;
#57982=CARTESIAN_POINT('',(-7.61344957909942E-16,-15.5,-34.0685435652414)) ;
#57983=CARTESIAN_POINT('',(5.6437440768064E-16,-7.75,-32.4669335366504)) ;
#57984=CARTESIAN_POINT('Origin',(-2.8473038080176E-15,-15.5,0.)) ;
#57985=CARTESIAN_POINT('',(-0.0148206788859343,-15.0366437072152,33.9727834182319)) ;
#57986=CARTESIAN_POINT('',(9.58677831405906E-9,-1.901536240759,31.2582937677921)) ;
#57987=CARTESIAN_POINT('Ctrl Pts',(-0.0148206796830926,-15.0366437072144,
33.9727834182323)) ;
#57988=CARTESIAN_POINT('Ctrl Pts',(-0.0147761934970794,-14.9636265798866,
33.9576937635085)) ;
#57989=CARTESIAN_POINT('Ctrl Pts',(-0.014731452265485,-14.8904290787823,
33.9425668329)) ;
#57990=CARTESIAN_POINT('Ctrl Pts',(-0.01434327996254,-14.2574947912553,
33.8117651948258)) ;
#57991=CARTESIAN_POINT('Ctrl Pts',(-0.0139852279340405,-13.6878788033261,
33.6940488603458)) ;
#57992=CARTESIAN_POINT('Ctrl Pts',(-0.0132371778195199,-12.5352441626078,
33.4558464085617)) ;
#57993=CARTESIAN_POINT('Ctrl Pts',(-0.0128472164427587,-11.9522255098215,
33.3353602912582)) ;
#57994=CARTESIAN_POINT('Ctrl Pts',(-0.012031151377517,-10.7794869194086,
33.093003175074)) ;
#57995=CARTESIAN_POINT('Ctrl Pts',(-0.0116051245489098,-10.1897669817304,
32.9711321761835)) ;
#57996=CARTESIAN_POINT('Ctrl Pts',(-0.0109330916398328,-9.30518714838486,
32.7883256929664)) ;
#57997=CARTESIAN_POINT('Ctrl Pts',(-0.0107035427670526,-9.01032721998394,
32.727390201878)) ;
#57998=CARTESIAN_POINT('Ctrl Pts',(-0.0102317470018941,-8.42144506509216,
32.6056923384334)) ;
#57999=CARTESIAN_POINT('Ctrl Pts',(-0.00998950899209841,-8.12742283859438,
32.5449299660763)) ;
#58000=CARTESIAN_POINT('Ctrl Pts',(-0.00949001810971001,-7.54105375785668,
32.4237514523057)) ;
#58001=CARTESIAN_POINT('Ctrl Pts',(-0.00923278420232808,-7.24870690362007,
32.363335310893)) ;
#58002=CARTESIAN_POINT('Ctrl Pts',(-0.00869987323933532,-6.66652623865879,
32.2430223714091)) ;
#58003=CARTESIAN_POINT('Ctrl Pts',(-0.00842423445942805,-6.37669242790047,
32.183125573331)) ;
#58004=CARTESIAN_POINT('Ctrl Pts',(-0.00799293179098999,-5.94445474907251,
32.0937997182736)) ;
#58005=CARTESIAN_POINT('Ctrl Pts',(-0.00784617116632075,-5.8007943635198,
32.0641109905068)) ;
#58006=CARTESIAN_POINT('Ctrl Pts',(-0.00754567856593524,-5.51441598220198,
32.0049282884094)) ;
#58007=CARTESIAN_POINT('Ctrl Pts',(-0.00739194776214034,-5.37169798643552,
31.9754343140794)) ;
#58008=CARTESIAN_POINT('Ctrl Pts',(-0.00707620189734833,-5.0873090933607,
31.9166627578568)) ;
#58009=CARTESIAN_POINT('Ctrl Pts',(-0.00691419331811431,-4.94563819605463,
31.887385175965)) ;
#58010=CARTESIAN_POINT('Ctrl Pts',(-0.00658008599236392,-4.66344820909719,
31.8290680437289)) ;
#58011=CARTESIAN_POINT('Ctrl Pts',(-0.00640800046290111,-4.52292911943078,
31.8000284933815)) ;
#58012=CARTESIAN_POINT('Ctrl Pts',(-0.00605114898957075,-4.24314745782051,
31.7422090635241)) ;
#58013=CARTESIAN_POINT('Ctrl Pts',(-0.0058664094908114,-4.10388488678362,
31.7134291842014)) ;
#58014=CARTESIAN_POINT('Ctrl Pts',(-0.00548031482479414,-3.82672097435253,
31.6561507360658)) ;
#58015=CARTESIAN_POINT('Ctrl Pts',(-0.00527901892921338,-3.68881963287913,
31.6276521672366)) ;
#58016=CARTESIAN_POINT('Ctrl Pts',(-0.00495976082686647,-3.48306707796744,
31.5851315268619)) ;
#58017=CARTESIAN_POINT('Ctrl Pts',(-0.00485042867486194,-3.41466613604316,
31.570995848916)) ;
#58018=CARTESIAN_POINT('Ctrl Pts',(-0.00462466717946779,-3.27824382794845,
31.5428029358115)) ;
#58019=CARTESIAN_POINT('Ctrl Pts',(-0.00450823986138664,-3.2102224617746,
31.5287457006532)) ;
#58020=CARTESIAN_POINT('Ctrl Pts',(-0.00426647698023381,-3.07457239569776,
31.5007123783991)) ;
#58021=CARTESIAN_POINT('Ctrl Pts',(-0.00414115714718083,-3.00694369580828,
31.4867362913064)) ;
#58022=CARTESIAN_POINT('Ctrl Pts',(-0.00387889601227492,-2.87209205434656,
31.4588679707746)) ;
#58023=CARTESIAN_POINT('Ctrl Pts',(-0.00374199348527815,-2.80486911270198,
31.4449757373206)) ;
#58024=CARTESIAN_POINT('Ctrl Pts',(-0.00346465861919957,-2.67661413836906,
31.4184706781625)) ;
#58025=CARTESIAN_POINT('Ctrl Pts',(-0.0033186339604559,-2.61231067593153,
31.4051817816902)) ;
#58026=CARTESIAN_POINT('Ctrl Pts',(-0.00307592509832223,-2.51355910906303,
31.3847738705318)) ;
#58027=CARTESIAN_POINT('Ctrl Pts',(-0.00299104803530146,-2.48025919132693,
31.3778921390891)) ;
#58028=CARTESIAN_POINT('Ctrl Pts',(-0.00281217424207543,-2.41327667158013,
31.3640495910111)) ;
#58029=CARTESIAN_POINT('Ctrl Pts',(-0.00271819528239995,-2.37959406952389,
31.3570887743664)) ;
#58030=CARTESIAN_POINT('Ctrl Pts',(-0.00251912676833825,-2.31222895652059,
31.3431671599055)) ;
#58031=CARTESIAN_POINT('Ctrl Pts',(-0.00241408123887382,-2.27854645923592,
31.3362063649129)) ;
#58032=CARTESIAN_POINT('Ctrl Pts',(-0.00224540359278948,-2.22830986861511,
31.3258245156846)) ;
#58033=CARTESIAN_POINT('Ctrl Pts',(-0.00218730809007332,-2.21161219769834,
31.3223737898337)) ;
#58034=CARTESIAN_POINT('Ctrl Pts',(-0.0020665726407671,-2.17836041986871,
31.3155020069411)) ;
#58035=CARTESIAN_POINT('Ctrl Pts',(-0.00200393495611065,-2.16180631294789,
31.3120809498982)) ;
#58036=CARTESIAN_POINT('Ctrl Pts',(-0.00187287329576513,-2.12888951005409,
31.3052783926287)) ;
#58037=CARTESIAN_POINT('Ctrl Pts',(-0.00180446694445819,-2.11252681791942,
31.3018968931955)) ;
#58038=CARTESIAN_POINT('Ctrl Pts',(-0.00165981089476397,-2.08004069522962,
31.2951833399147)) ;
#58039=CARTESIAN_POINT('Ctrl Pts',(-0.00158360917355472,-2.06391726446957,
31.291851286025)) ;
#58040=CARTESIAN_POINT('Ctrl Pts',(-0.00146057179251287,-2.03994745220908,
31.2868977058982)) ;
#58041=CARTESIAN_POINT('Ctrl Pts',(-0.00141807818111219,-2.03199340463373,
31.2852539294864)) ;
#58042=CARTESIAN_POINT('Ctrl Pts',(-0.00132928283223824,-2.01616307091637,
31.281982446771)) ;
#58043=CARTESIAN_POINT('Ctrl Pts',(-0.00128298191126172,-2.00828678476986,
31.280354740467)) ;
#58044=CARTESIAN_POINT('Ctrl Pts',(-0.00118517612253733,-1.99261795861226,
31.2771166347607)) ;
#58045=CARTESIAN_POINT('Ctrl Pts',(-0.00113369979187007,-1.98482541877565,
31.2755062353946)) ;
#58046=CARTESIAN_POINT('Ctrl Pts',(-0.00105070864777337,-1.97320391184726,
31.2731045450879)) ;
#58047=CARTESIAN_POINT('Ctrl Pts',(-0.00102207037490944,-1.96934129344584,
31.2723062997975)) ;
#58048=CARTESIAN_POINT('Ctrl Pts',(-0.000962302516201868,-1.9616392413869,
31.2707146005552)) ;
#58049=CARTESIAN_POINT('Ctrl Pts',(-0.000931174692610054,-1.9577998077162,
31.2699211466007)) ;
#58050=CARTESIAN_POINT('Ctrl Pts',(-0.000865532982845733,-1.9501397428687,
31.2683381243983)) ;
#58051=CARTESIAN_POINT('Ctrl Pts',(-0.000829293872646199,-1.94611557964085,
31.2675064943974)) ;
#58052=CARTESIAN_POINT('Ctrl Pts',(-0.000748920269517818,-1.93787585622421,
31.2658036804696)) ;
#58053=CARTESIAN_POINT('Ctrl Pts',(-0.000704858395548698,-1.93366029535625,
31.2649324964023)) ;
#58054=CARTESIAN_POINT('Ctrl Pts',(-0.000630605424405322,-1.92733721691345,
31.2636257746236)) ;
#58055=CARTESIAN_POINT('Ctrl Pts',(-0.000604477929136395,-1.92522958117288,
31.2631902124922)) ;
#58056=CARTESIAN_POINT('Ctrl Pts',(-0.000548532542702596,-1.92103837449027,
31.2623240614392)) ;
#58057=CARTESIAN_POINT('Ctrl Pts',(-0.000518750289895745,-1.91895480309204,
31.2618934724234)) ;
#58058=CARTESIAN_POINT('Ctrl Pts',(-0.000469852903473204,-1.91586546722132,
31.2612550330144)) ;
#58059=CARTESIAN_POINT('Ctrl Pts',(-0.000452838239228457,-1.91484169594687,
31.2610434613515)) ;
#58060=CARTESIAN_POINT('Ctrl Pts',(-0.000416879002336717,-1.91280916054715,
31.2606234193898)) ;
#58061=CARTESIAN_POINT('Ctrl Pts',(-0.000397937068286648,-1.9118003963771,
31.2604149490818)) ;
#58062=CARTESIAN_POINT('Ctrl Pts',(-0.000357192200659911,-1.9098008749712,
31.2600017297628)) ;
#58063=CARTESIAN_POINT('Ctrl Pts',(-0.000335428304312129,-1.90881011956137,
31.2597969811292)) ;
#58064=CARTESIAN_POINT('Ctrl Pts',(-0.000299075801589961,-1.90733975547413,
31.259493116992)) ;
#58065=CARTESIAN_POINT('Ctrl Pts',(-0.000286330749186815,-1.90685226278536,
31.2593923721857)) ;
#58066=CARTESIAN_POINT('Ctrl Pts',(-0.000258978203130866,-1.90588291853958,
31.2591920483642)) ;
#58067=CARTESIAN_POINT('Ctrl Pts',(-0.000244394768655416,-1.90540106633159,
31.2590924692146)) ;
#58068=CARTESIAN_POINT('Ctrl Pts',(-0.000219952978457789,-1.90467591230858,
31.2589426095278)) ;
#58069=CARTESIAN_POINT('Ctrl Pts',(-0.000210792012095635,-1.90441732984955,
31.2588891711064)) ;
#58070=CARTESIAN_POINT('Ctrl Pts',(-0.000190504227060032,-1.9038880529221,
31.2587797912063)) ;
#58071=CARTESIAN_POINT('Ctrl Pts',(-0.000179382359458563,-1.90361735827164,
31.2587238496901)) ;
#58072=CARTESIAN_POINT('Ctrl Pts',(-0.000154443127708429,-1.90307628163011,
31.2586120312716)) ;
#58073=CARTESIAN_POINT('Ctrl Pts',(-0.000140721200959569,-1.90280593840711,
31.2585561623812)) ;
#58074=CARTESIAN_POINT('Ctrl Pts',(-1.07819935174354E-5,-1.90163368866297,
31.2583139062895)) ;
#58075=CARTESIAN_POINT('Ctrl Pts',(-5.38608092278449E-6,-1.90158500930527,
31.2583038462567)) ;
#58076=CARTESIAN_POINT('Ctrl Pts',(9.83167186641764E-9,-1.90153632994757,
31.2582937862238)) ;
#58077=CARTESIAN_POINT('',(0.0148206788852317,-15.0366437072152,33.9727834182319)) ;
#58078=CARTESIAN_POINT('Origin',(0.,-21.6462763158693,-1.36594255531499)) ;
#58079=CARTESIAN_POINT('Ctrl Pts',(9.83167186641764E-9,-1.90153632994757,
31.2582937862238)) ;
#58080=CARTESIAN_POINT('Ctrl Pts',(5.40498507600443E-6,-1.90158500938597,
31.2583038462733)) ;
#58081=CARTESIAN_POINT('Ctrl Pts',(1.08001384804997E-5,-1.90163368882437,
31.2583139063229)) ;
#58082=CARTESIAN_POINT('Ctrl Pts',(0.000140721346216588,-1.90280594305982,
31.2585561633427)) ;
#58083=CARTESIAN_POINT('Ctrl Pts',(0.000154443545858063,-1.90307628603679,
31.2586120321823)) ;
#58084=CARTESIAN_POINT('Ctrl Pts',(0.000179382728467112,-1.90361736221603,
31.2587238505053)) ;
#58085=CARTESIAN_POINT('Ctrl Pts',(0.000190504320645866,-1.90388805664502,
31.2587797919757)) ;
#58086=CARTESIAN_POINT('Ctrl Pts',(0.00021079206978046,-1.90441733312078,
31.2588891717824)) ;
#58087=CARTESIAN_POINT('Ctrl Pts',(0.000219952985965777,-1.90467591536023,
31.2589426101585)) ;
#58088=CARTESIAN_POINT('Ctrl Pts',(0.000244394767151704,-1.90540106911698,
31.2590924697902)) ;
#58089=CARTESIAN_POINT('Ctrl Pts',(0.000258978255278715,-1.90588292126836,
31.2591920489281)) ;
#58090=CARTESIAN_POINT('Ctrl Pts',(0.000286330784955126,-1.90685226540366,
31.2593923727268)) ;
#58091=CARTESIAN_POINT('Ctrl Pts',(0.000299075816320136,-1.9073397580372,
31.2594931175217)) ;
#58092=CARTESIAN_POINT('Ctrl Pts',(0.000335428305529032,-1.90881012195651,
31.2597969816242)) ;
#58093=CARTESIAN_POINT('Ctrl Pts',(0.000357192224140643,-1.90980087725246,
31.2600017302343)) ;
#58094=CARTESIAN_POINT('Ctrl Pts',(0.000397937081915845,-1.91180039842972,
31.260414949506)) ;
#58095=CARTESIAN_POINT('Ctrl Pts',(0.000416879027904655,-1.91280916248412,
31.2606234197901)) ;
#58096=CARTESIAN_POINT('Ctrl Pts',(0.000452838258712398,-1.9148416976513,
31.2610434617038)) ;
#58097=CARTESIAN_POINT('Ctrl Pts',(0.000469852938162042,-1.9158654688083,
31.2612550333424)) ;
#58098=CARTESIAN_POINT('Ctrl Pts',(0.000518750313335333,-1.91895480432564,
31.2618934726783)) ;
#58099=CARTESIAN_POINT('Ctrl Pts',(0.000548532557564341,-1.92103837548551,
31.2623240616449)) ;
#58100=CARTESIAN_POINT('Ctrl Pts',(0.000604477934722621,-1.92522958168858,
31.2631902125987)) ;
#58101=CARTESIAN_POINT('Ctrl Pts',(0.000630605459915997,-1.92733721718753,
31.2636257746802)) ;
#58102=CARTESIAN_POINT('Ctrl Pts',(0.00070485841900451,-1.93366029490678,
31.2649324963094)) ;
#58103=CARTESIAN_POINT('Ctrl Pts',(0.000748920258238895,-1.93787585529259,
31.2658036802771)) ;
#58104=CARTESIAN_POINT('Ctrl Pts',(0.000829293852258837,-1.94611557776626,
31.26750649401)) ;
#58105=CARTESIAN_POINT('Ctrl Pts',(0.000865532986477288,-1.9501397405333,
31.2683381239156)) ;
#58106=CARTESIAN_POINT('Ctrl Pts',(0.000931174692604608,-1.95779980495566,
31.2699211460302)) ;
#58107=CARTESIAN_POINT('Ctrl Pts',(0.000962302480328251,-1.96163923864022,
31.2707145999876)) ;
#58108=CARTESIAN_POINT('Ctrl Pts',(0.00102207033992775,-1.9693412907264,
31.2723062992355)) ;
#58109=CARTESIAN_POINT('Ctrl Pts',(0.00105070862597898,-1.97320390914139,
31.2731045445287)) ;
#58110=CARTESIAN_POINT('Ctrl Pts',(0.00113369977366347,-1.98482541611087,
31.2755062348439)) ;
#58111=CARTESIAN_POINT('Ctrl Pts',(0.00118517610350443,-1.99261795597505,
31.2771166342157)) ;
#58112=CARTESIAN_POINT('Ctrl Pts',(0.0012829818947538,-2.00828678218809,
31.2803547399334)) ;
#58113=CARTESIAN_POINT('Ctrl Pts',(0.00132928283070744,-2.01616306836236,
31.2819824462432)) ;
#58114=CARTESIAN_POINT('Ctrl Pts',(0.00141807818099176,-2.03199340213575,
31.2852539289702)) ;
#58115=CARTESIAN_POINT('Ctrl Pts',(0.00146057177435883,-2.03994744973935,
31.2868977053878)) ;
#58116=CARTESIAN_POINT('Ctrl Pts',(0.00158360915669288,-2.06391726208467,
31.2918512855321)) ;
#58117=CARTESIAN_POINT('Ctrl Pts',(0.001659810895993,-2.08004069290168,
31.2951833394336)) ;
#58118=CARTESIAN_POINT('Ctrl Pts',(0.00180446694663054,-2.11252681570644,
31.3018968927381)) ;
#58119=CARTESIAN_POINT('Ctrl Pts',(0.00187287328849277,-2.12888950789906,
31.3052783921833)) ;
#58120=CARTESIAN_POINT('Ctrl Pts',(0.00200393494937599,-2.16180631090932,
31.3120809494769)) ;
#58121=CARTESIAN_POINT('Ctrl Pts',(0.00206657262782834,-2.17836041788876,
31.3155020065319)) ;
#58122=CARTESIAN_POINT('Ctrl Pts',(0.00218730807792908,-2.21161219583605,
31.3223737894488)) ;
#58123=CARTESIAN_POINT('Ctrl Pts',(0.00224540358654324,-2.22830986681189,
31.3258245153119)) ;
#58124=CARTESIAN_POINT('Ctrl Pts',(0.00241408123334814,-2.27854645761049,
31.336206364577)) ;
#58125=CARTESIAN_POINT('Ctrl Pts',(0.00251912676155658,-2.31222895501437,
31.3431671595943)) ;
#58126=CARTESIAN_POINT('Ctrl Pts',(0.00271819527582991,-2.37959406825606,
31.3570887741044)) ;
#58127=CARTESIAN_POINT('Ctrl Pts',(0.00281217424613174,-2.41327667043147,
31.3640495907737)) ;
#58128=CARTESIAN_POINT('Ctrl Pts',(0.00299104804018365,-2.48025919041532,
31.3778921389007)) ;
#58129=CARTESIAN_POINT('Ctrl Pts',(0.00307592509813755,-2.51355910826926,
31.3847738703678)) ;
#58130=CARTESIAN_POINT('Ctrl Pts',(0.00331863396146083,-2.61231067548724,
31.4051817815983)) ;
#58131=CARTESIAN_POINT('Ctrl Pts',(0.00346465861835736,-2.67661413815233,
31.4184706781177)) ;
#58132=CARTESIAN_POINT('Ctrl Pts',(0.0037419934849328,-2.80486911270198,
31.4449757373206)) ;
#58133=CARTESIAN_POINT('Ctrl Pts',(0.00387889601224861,-2.87209205434656,
31.4588679707746)) ;
#58134=CARTESIAN_POINT('Ctrl Pts',(0.00414115714715684,-3.00694369580827,
31.4867362913064)) ;
#58135=CARTESIAN_POINT('Ctrl Pts',(0.0042664769804943,-3.07457239569777,
31.5007123783991)) ;
#58136=CARTESIAN_POINT('Ctrl Pts',(0.00450823986163544,-3.2102224617746,
31.5287457006532)) ;
#58137=CARTESIAN_POINT('Ctrl Pts',(0.00462466717990583,-3.27824382794846,
31.5428029358115)) ;
#58138=CARTESIAN_POINT('Ctrl Pts',(0.00485042867526996,-3.41466613604315,
31.570995848916)) ;
#58139=CARTESIAN_POINT('Ctrl Pts',(0.00495976082741732,-3.48306707796744,
31.5851315268619)) ;
#58140=CARTESIAN_POINT('Ctrl Pts',(0.00527901892971909,-3.68881963287913,
31.6276521672366)) ;
#58141=CARTESIAN_POINT('Ctrl Pts',(0.00548031481950349,-3.82672097435253,
31.6561507360658)) ;
#58142=CARTESIAN_POINT('Ctrl Pts',(0.00586640948546941,-4.10388488678362,
31.7134291842014)) ;
#58143=CARTESIAN_POINT('Ctrl Pts',(0.0060511489907128,-4.2431474578205,
31.7422090635241)) ;
#58144=CARTESIAN_POINT('Ctrl Pts',(0.00640800046407745,-4.52292911943078,
31.8000284933815)) ;
#58145=CARTESIAN_POINT('Ctrl Pts',(0.00658008599084795,-4.66344820909719,
31.8290680437289)) ;
#58146=CARTESIAN_POINT('Ctrl Pts',(0.00691419331657868,-4.94563819605463,
31.887385175965)) ;
#58147=CARTESIAN_POINT('Ctrl Pts',(0.0070762018962943,-5.08730909336069,
31.9166627578568)) ;
#58148=CARTESIAN_POINT('Ctrl Pts',(0.00739194776104187,-5.37169798643551,
31.9754343140794)) ;
#58149=CARTESIAN_POINT('Ctrl Pts',(0.00754567856520655,-5.51441598220197,
32.0049282884094)) ;
#58150=CARTESIAN_POINT('Ctrl Pts',(0.00784617116563057,-5.80079436351979,
32.0641109905068)) ;
#58151=CARTESIAN_POINT('Ctrl Pts',(0.00799293179047366,-5.94445474907251,
32.0937997182736)) ;
#58152=CARTESIAN_POINT('Ctrl Pts',(0.00842423445892503,-6.37669242790047,
32.183125573331)) ;
#58153=CARTESIAN_POINT('Ctrl Pts',(0.00869987323869593,-6.66652623865878,
32.2430223714091)) ;
#58154=CARTESIAN_POINT('Ctrl Pts',(0.00923278420170785,-7.24870690362006,
32.363335310893)) ;
#58155=CARTESIAN_POINT('Ctrl Pts',(0.00949001810909513,-7.54105375785668,
32.4237514523057)) ;
#58156=CARTESIAN_POINT('Ctrl Pts',(0.00998950899150371,-8.12742283859435,
32.5449299660763)) ;
#58157=CARTESIAN_POINT('Ctrl Pts',(0.0102317469989513,-8.42144506509215,
32.6056923384334)) ;
#58158=CARTESIAN_POINT('Ctrl Pts',(0.0107035427641363,-9.01032721998393,
32.727390201878)) ;
#58159=CARTESIAN_POINT('Ctrl Pts',(0.0109330916392549,-9.30518714838485,
32.7883256929664)) ;
#58160=CARTESIAN_POINT('Ctrl Pts',(0.011605124548404,-10.1897669817304,
32.9711321761835)) ;
#58161=CARTESIAN_POINT('Ctrl Pts',(0.0120311513767769,-10.7794869194086,
33.093003175074)) ;
#58162=CARTESIAN_POINT('Ctrl Pts',(0.0128472164422006,-11.9522255098215,
33.3353602912582)) ;
#58163=CARTESIAN_POINT('Ctrl Pts',(0.0132371778185301,-12.5352441626078,
33.4558464085617)) ;
#58164=CARTESIAN_POINT('Ctrl Pts',(0.0139852279330011,-13.6878788033261,
33.6940488603458)) ;
#58165=CARTESIAN_POINT('Ctrl Pts',(0.0143432799612731,-14.2574947912552,
33.8117651948258)) ;
#58166=CARTESIAN_POINT('Ctrl Pts',(0.0147314522641499,-14.8904290787823,
33.9425668329)) ;
#58167=CARTESIAN_POINT('Ctrl Pts',(0.0147761934957339,-14.9636265798866,
33.9576937635085)) ;
#58168=CARTESIAN_POINT('Ctrl Pts',(0.014820679681735,-15.0366437072144,
33.9727834182323)) ;
#58169=CARTESIAN_POINT('',(14.2782523899403,-15.0366437072153,30.8266401270693)) ;
#58170=CARTESIAN_POINT('',(14.2513506240286,-15.0366437072153,30.8390862093169)) ;
#58171=CARTESIAN_POINT('Origin',(-0.573544392334149,-21.6462763158694,-1.23969588788643)) ;
#58172=CARTESIAN_POINT('',(13.1250168957584,-1.901536243719,28.3692590808765)) ;
#58173=CARTESIAN_POINT('Ctrl Pts',(13.1250169039853,-1.90153633586757,28.369259098053)) ;
#58174=CARTESIAN_POINT('Ctrl Pts',(13.1250269478319,-1.90158489539068,28.3692655085023)) ;
#58175=CARTESIAN_POINT('Ctrl Pts',(13.1251996720784,-1.90241997455468,28.3693757491368)) ;
#58176=CARTESIAN_POINT('Ctrl Pts',(13.1252567763422,-1.90282053169335,28.3694405386005)) ;
#58177=CARTESIAN_POINT('Ctrl Pts',(13.1252930337436,-1.90309401349771,28.3694860372096)) ;
#58178=CARTESIAN_POINT('Ctrl Pts',(13.1253632958455,-1.90364136769095,28.3695781655761)) ;
#58179=CARTESIAN_POINT('Ctrl Pts',(13.1253972100022,-1.9039152012528,28.3696248283824)) ;
#58180=CARTESIAN_POINT('Ctrl Pts',(13.1254621893454,-1.90445061351417,28.3697166815804)) ;
#58181=CARTESIAN_POINT('Ctrl Pts',(13.1254932500133,-1.90471219239629,28.3697618741041)) ;
#58182=CARTESIAN_POINT('Ctrl Pts',(13.1255792249785,-1.9054458353377,28.3698891517338)) ;
#58183=CARTESIAN_POINT('Ctrl Pts',(13.1256348435025,-1.90593335789139,28.3699744310004)) ;
#58184=CARTESIAN_POINT('Ctrl Pts',(13.1257449190649,-1.90691410886923,28.3701468261471)) ;
#58185=CARTESIAN_POINT('Ctrl Pts',(13.1257993541738,-1.90740733794508,28.3702339523212)) ;
#58186=CARTESIAN_POINT('Ctrl Pts',(13.1259616328036,-1.90889500365118,28.3704976225806)) ;
#58187=CARTESIAN_POINT('Ctrl Pts',(13.1260684852153,-1.90989741674749,28.3706764414799)) ;
#58188=CARTESIAN_POINT('Ctrl Pts',(13.1262812303969,-1.91192046485291,28.3710386724698)) ;
#58189=CARTESIAN_POINT('Ctrl Pts',(13.1263870873956,-1.91294109803394,28.3712221006936)) ;
#58190=CARTESIAN_POINT('Ctrl Pts',(13.1265983616806,-1.91499754756168,28.3715926178508)) ;
#58191=CARTESIAN_POINT('Ctrl Pts',(13.1267037766399,-1.91603336395173,28.3717797078706)) ;
#58192=CARTESIAN_POINT('Ctrl Pts',(13.1270196437705,-1.91915904650413,28.3723453045198)) ;
#58193=CARTESIAN_POINT('Ctrl Pts',(13.1272297591902,-1.92126713079265,28.3727281152986)) ;
#58194=CARTESIAN_POINT('Ctrl Pts',(13.1276487985653,-1.92550764503829,28.3734998317072)) ;
#58195=CARTESIAN_POINT('Ctrl Pts',(13.1278576900239,-1.92764007545159,28.3738887524756)) ;
#58196=CARTESIAN_POINT('Ctrl Pts',(13.1284806092693,-1.93403753795706,28.3750572910872)) ;
#58197=CARTESIAN_POINT('Ctrl Pts',(13.1288909375366,-1.93830268824026,28.3758386474229)) ;
#58198=CARTESIAN_POINT('Ctrl Pts',(13.1296877148954,-1.94663933648012,28.3773683122489)) ;
#58199=CARTESIAN_POINT('Ctrl Pts',(13.1300740977459,-1.95071083511603,28.3781166515402)) ;
#58200=CARTESIAN_POINT('Ctrl Pts',(13.1308065738439,-1.95846141420779,28.379542614647)) ;
#58201=CARTESIAN_POINT('Ctrl Pts',(13.1311721109147,-1.96234642274043,28.3802581335656)) ;
#58202=CARTESIAN_POINT('Ctrl Pts',(13.1319029492433,-1.97013989960687,28.3816946224065)) ;
#58203=CARTESIAN_POINT('Ctrl Pts',(13.1322682488701,-1.974048367954,28.3824155930864)) ;
#58204=CARTESIAN_POINT('Ctrl Pts',(13.1333644330489,-1.98580782403353,28.3845861267117)) ;
#58205=CARTESIAN_POINT('Ctrl Pts',(13.1340956458595,-1.99369286238981,28.3860432912726)) ;
#58206=CARTESIAN_POINT('Ctrl Pts',(13.1355607255424,-2.00954767943326,28.3889756882594)) ;
#58207=CARTESIAN_POINT('Ctrl Pts',(13.1362945663458,-2.01751745794586,28.3904509327061)) ;
#58208=CARTESIAN_POINT('Ctrl Pts',(13.1377656003264,-2.03353569925263,28.3934177874007)) ;
#58209=CARTESIAN_POINT('Ctrl Pts',(13.138502792754,-2.04158416205131,28.394909397996)) ;
#58210=CARTESIAN_POINT('Ctrl Pts',(13.1407197670541,-2.06583849778387,28.399406540668)) ;
#58211=CARTESIAN_POINT('Ctrl Pts',(13.1422050381934,-2.08215331459392,28.4024343401622)) ;
#58212=CARTESIAN_POINT('Ctrl Pts',(13.1451895153445,-2.11502504894364,28.4085386196463)) ;
#58213=CARTESIAN_POINT('Ctrl Pts',(13.1466886775721,-2.13158196668823,28.4116151199393)) ;
#58214=CARTESIAN_POINT('Ctrl Pts',(13.1496985589263,-2.16488949245127,28.4178068779039)) ;
#58215=CARTESIAN_POINT('Ctrl Pts',(13.151209261612,-2.1816400966306,28.4209221423076)) ;
#58216=CARTESIAN_POINT('Ctrl Pts',(13.1542391277507,-2.21528657271386,28.427181834879)) ;
#58217=CARTESIAN_POINT('Ctrl Pts',(13.1557582891559,-2.23218244462569,28.4303262639956)) ;
#58218=CARTESIAN_POINT('Ctrl Pts',(13.1603232595078,-2.28301534196996,28.439789169183)) ;
#58219=CARTESIAN_POINT('Ctrl Pts',(13.1633766205547,-2.31709764872116,28.4461372325071)) ;
#58220=CARTESIAN_POINT('Ctrl Pts',(13.1694732902846,-2.38526238067128,28.4588380368451)) ;
#58221=CARTESIAN_POINT('Ctrl Pts',(13.1725165575778,-2.41934479220568,28.4651907938965)) ;
#58222=CARTESIAN_POINT('Ctrl Pts',(13.1785611978818,-2.48712238762728,28.4778275168357)) ;
#58223=CARTESIAN_POINT('Ctrl Pts',(13.1815625546765,-2.52081757156001,28.4841114902361)) ;
#58224=CARTESIAN_POINT('Ctrl Pts',(13.1904549255812,-2.6207413071602,28.5027505372084)) ;
#58225=CARTESIAN_POINT('Ctrl Pts',(13.1962343453641,-2.68580804227443,28.5148926888216)) ;
#58226=CARTESIAN_POINT('Ctrl Pts',(13.20775574064,-2.81566304839315,28.5391309080581)) ;
#58227=CARTESIAN_POINT('Ctrl Pts',(13.2137900707651,-2.88376182393009,28.5518455351887)) ;
#58228=CARTESIAN_POINT('Ctrl Pts',(13.2258838404761,-3.02037041957963,28.5773567693237)) ;
#58229=CARTESIAN_POINT('Ctrl Pts',(13.2319432444941,-3.08888023976489,28.5901533928)) ;
#58230=CARTESIAN_POINT('Ctrl Pts',(13.2440884526074,-3.22629766229947,28.6158250026112)) ;
#58231=CARTESIAN_POINT('Ctrl Pts',(13.2501742422778,-3.29520526463518,28.6286999956163)) ;
#58232=CARTESIAN_POINT('Ctrl Pts',(13.2623727032053,-3.43340499038686,28.6545251021062)) ;
#58233=CARTESIAN_POINT('Ctrl Pts',(13.268485372607,-3.50269711380624,28.6674752164491)) ;
#58234=CARTESIAN_POINT('Ctrl Pts',(13.2868637167533,-3.71113037540774,28.7064337048146)) ;
#58235=CARTESIAN_POINT('Ctrl Pts',(13.2991698265153,-3.85082840427815,28.7325501781858)) ;
#58236=CARTESIAN_POINT('Ctrl Pts',(13.3238866282531,-4.13160342647603,28.7850487366164)) ;
#58237=CARTESIAN_POINT('Ctrl Pts',(13.336297265978,-4.27268041988289,28.8114308467927)) ;
#58238=CARTESIAN_POINT('Ctrl Pts',(13.3612174575322,-4.55610729697891,28.8644391466752)) ;
#58239=CARTESIAN_POINT('Ctrl Pts',(13.373726987082,-4.69845717975854,28.8910653474071)) ;
#58240=CARTESIAN_POINT('Ctrl Pts',(13.3988381015789,-4.98432375945421,28.9445408484739)) ;
#58241=CARTESIAN_POINT('Ctrl Pts',(13.4114396744345,-5.12784045638525,28.9713901544063)) ;
#58242=CARTESIAN_POINT('Ctrl Pts',(13.436727309626,-5.41593459099438,29.0252912128394)) ;
#58243=CARTESIAN_POINT('Ctrl Pts',(13.4494133660345,-5.56051202867017,29.0523429680818)) ;
#58244=CARTESIAN_POINT('Ctrl Pts',(13.4748619542698,-5.85062157186436,29.1066284795457)) ;
#58245=CARTESIAN_POINT('Ctrl Pts',(13.4876244850246,-5.99615367738409,29.1338622362626)) ;
#58246=CARTESIAN_POINT('Ctrl Pts',(13.5260143312979,-6.43402288686051,29.2158060422649)) ;
#58247=CARTESIAN_POINT('Ctrl Pts',(13.5517439698395,-6.7276328790384,29.2707585944021)) ;
#58248=CARTESIAN_POINT('Ctrl Pts',(13.6034073853403,-7.31739864832443,29.3811489411672)) ;
#58249=CARTESIAN_POINT('Ctrl Pts',(13.6293411273095,-7.6135544254662,29.436586751991)) ;
#58250=CARTESIAN_POINT('Ctrl Pts',(13.6813422113443,-8.20756317967979,29.5477870239103)) ;
#58251=CARTESIAN_POINT('Ctrl Pts',(13.7074095360699,-8.50541615674834,29.6035494930274)) ;
#58252=CARTESIAN_POINT('Ctrl Pts',(13.759606248396,-9.10197072662847,29.7152389516399)) ;
#58253=CARTESIAN_POINT('Ctrl Pts',(13.7857356278777,-9.40067231944697,29.7711659448926)) ;
#58254=CARTESIAN_POINT('Ctrl Pts',(13.8641086058114,-10.2967771460885,29.9389539496253)) ;
#58255=CARTESIAN_POINT('Ctrl Pts',(13.916337185494,-10.8941804126697,30.0508219169838)) ;
#58256=CARTESIAN_POINT('Ctrl Pts',(14.0201724215159,-12.0821983504006,30.2732997895653)) ;
#58257=CARTESIAN_POINT('Ctrl Pts',(14.071779007624,-12.6728130216019,30.3839097272913)) ;
#58258=CARTESIAN_POINT('Ctrl Pts',(14.1753539738539,-13.8584258096385,30.6059603498131)) ;
#58259=CARTESIAN_POINT('Ctrl Pts',(14.2272846073097,-14.4529998121294,30.7173219252823)) ;
#58260=CARTESIAN_POINT('Ctrl Pts',(14.2782523900528,-15.0366437072152,30.8266401270172)) ;
#58261=CARTESIAN_POINT('Ctrl Pts',(14.2513506239141,-15.0366437072152,30.8390862093698)) ;
#58262=CARTESIAN_POINT('Ctrl Pts',(14.2498487196638,-15.0192244618052,30.8358146216817)) ;
#58263=CARTESIAN_POINT('Ctrl Pts',(14.2483459834305,-15.0017954802462,30.8325412019439)) ;
#58264=CARTESIAN_POINT('Ctrl Pts',(14.1979681755858,-14.4175024637988,30.7228022408249)) ;
#58265=CARTESIAN_POINT('Ctrl Pts',(14.1482238960184,-13.8404650786097,30.6144223190429)) ;
#58266=CARTESIAN_POINT('Ctrl Pts',(14.0475863486083,-12.6728130223236,30.3951024433868)) ;
#58267=CARTESIAN_POINT('Ctrl Pts',(13.9966930472133,-12.0821983512294,30.2841625050364)) ;
#58268=CARTESIAN_POINT('Ctrl Pts',(13.8943503623223,-10.894180413714,30.0609941048191)) ;
#58269=CARTESIAN_POINT('Ctrl Pts',(13.842900908589,-10.2967771472412,29.9487656754368)) ;
#58270=CARTESIAN_POINT('Ctrl Pts',(13.7657568491019,-9.40067232076225,29.7804091125241)) ;
#58271=CARTESIAN_POINT('Ctrl Pts',(13.7400472188986,-9.10197072799794,29.7242879225883)) ;
#58272=CARTESIAN_POINT('Ctrl Pts',(13.6887131872663,-8.50541615822605,29.6121993454108)) ;
#58273=CARTESIAN_POINT('Ctrl Pts',(13.6630887777184,-8.20756318121152,29.5562319619242)) ;
#58274=CARTESIAN_POINT('Ctrl Pts',(13.6120009385489,-7.61355442710567,29.4446091779631)) ;
#58275=CARTESIAN_POINT('Ctrl Pts',(13.5865374915885,-7.31739865001763,29.388953785511)) ;
#58276=CARTESIAN_POINT('Ctrl Pts',(13.5358483446611,-6.72763288083859,29.27811269413)) ;
#58277=CARTESIAN_POINT('Ctrl Pts',(13.5106226096945,-6.43402288871397,29.222927011386)) ;
#58278=CARTESIAN_POINT('Ctrl Pts',(13.4730212100658,-5.99615367931698,29.1406184311406)) ;
#58279=CARTESIAN_POINT('Ctrl Pts',(13.4605269614545,-5.85062157382364,29.1132605538929)) ;
#58280=CARTESIAN_POINT('Ctrl Pts',(13.4356276714686,-5.5605120306821,29.0587209100092)) ;
#58281=CARTESIAN_POINT('Ctrl Pts',(13.4232226290259,-5.41593459303255,29.0315391438679)) ;
#58282=CARTESIAN_POINT('Ctrl Pts',(13.3985121557589,-5.12784045847568,28.977371061906)) ;
#58283=CARTESIAN_POINT('Ctrl Pts',(13.3862067190029,-4.98432376157065,28.9503847488305)) ;
#58284=CARTESIAN_POINT('Ctrl Pts',(13.3617063123363,-4.69845718192687,28.8966267042463)) ;
#58285=CARTESIAN_POINT('Ctrl Pts',(13.3495113303281,-4.55610729917304,28.869854978331)) ;
#58286=CARTESIAN_POINT('Ctrl Pts',(13.3252434057812,-4.27268042212843,28.8165449076082)) ;
#58287=CARTESIAN_POINT('Ctrl Pts',(13.3131704391221,-4.13160342874717,28.790006574167)) ;
#58288=CARTESIAN_POINT('Ctrl Pts',(13.2891593483905,-3.85082840660023,28.7371815190693)) ;
#58289=CARTESIAN_POINT('Ctrl Pts',(13.2772211700524,-3.71113037775515,28.7108948225007)) ;
#58290=CARTESIAN_POINT('Ctrl Pts',(13.2594263764353,-3.50269711619146,28.6716663549198)) ;
#58291=CARTESIAN_POINT('Ctrl Pts',(13.2535135490082,-3.43340499278465,28.658623783837)) ;
#58292=CARTESIAN_POINT('Ctrl Pts',(13.2417277490737,-3.29520526705806,28.6326077600474)) ;
#58293=CARTESIAN_POINT('Ctrl Pts',(13.2358547747125,-3.22629766473483,28.6196343081985)) ;
#58294=CARTESIAN_POINT('Ctrl Pts',(13.2241514889807,-3.08888024222519,28.5937582433277)) ;
#58295=CARTESIAN_POINT('Ctrl Pts',(13.2183211631902,-3.02037042205235,28.5808556369805)) ;
#58296=CARTESIAN_POINT('Ctrl Pts',(13.2067068091968,-2.88376182642761,28.5551226015214)) ;
#58297=CARTESIAN_POINT('Ctrl Pts',(13.2009227454198,-2.81566305090302,28.5422921888514)) ;
#58298=CARTESIAN_POINT('Ctrl Pts',(13.1899080877081,-2.68580804467985,28.5178195278291)) ;
#58299=CARTESIAN_POINT('Ctrl Pts',(13.1843953175679,-2.62074130944303,28.5055540109265)) ;
#58300=CARTESIAN_POINT('Ctrl Pts',(13.1759461421688,-2.52081757365458,28.4867099198361)) ;
#58301=CARTESIAN_POINT('Ctrl Pts',(13.1730997733076,-2.48712238965837,28.4803542413676)) ;
#58302=CARTESIAN_POINT('Ctrl Pts',(13.1673817598006,-2.41934479410906,28.4675664047515)) ;
#58303=CARTESIAN_POINT('Ctrl Pts',(13.1645100989313,-2.38526238251044,28.4611342540995)) ;
#58304=CARTESIAN_POINT('Ctrl Pts',(13.1587769281494,-2.3170976504319,28.4482652772108)) ;
#58305=CARTESIAN_POINT('Ctrl Pts',(13.1559153792237,-2.2830153436165,28.4418284721351)) ;
#58306=CARTESIAN_POINT('Ctrl Pts',(13.1516584111466,-2.23218244617646,28.4322230698995)) ;
#58307=CARTESIAN_POINT('Ctrl Pts',(13.1502453308303,-2.21528657423275,28.4290295624378)) ;
#58308=CARTESIAN_POINT('Ctrl Pts',(13.1474359244531,-2.18164009808608,28.4226678743052)) ;
#58309=CARTESIAN_POINT('Ctrl Pts',(13.1460395963361,-2.16488949387522,28.4194996945841)) ;
#58310=CARTESIAN_POINT('Ctrl Pts',(13.1432690292635,-2.13158196804943,28.4131972180285)) ;
#58311=CARTESIAN_POINT('Ctrl Pts',(13.1418947745461,-2.11502505027367,28.4100629293605)) ;
#58312=CARTESIAN_POINT('Ctrl Pts',(13.1391744339186,-2.08215331586202,28.4038364472936)) ;
#58313=CARTESIAN_POINT('Ctrl Pts',(13.1378283041887,-2.06583849902119,28.4007442741215)) ;
#58314=CARTESIAN_POINT('Ctrl Pts',(13.1358359914392,-2.04158416324294,28.3961431919376)) ;
#58315=CARTESIAN_POINT('Ctrl Pts',(13.135176390713,-2.0335357004291,28.3946156835952)) ;
#58316=CARTESIAN_POINT('Ctrl Pts',(13.1338674938624,-2.01751745909216,28.3915738162696)) ;
#58317=CARTESIAN_POINT('Ctrl Pts',(13.1332181969884,-2.00954768056451,28.3900594576326)) ;
#58318=CARTESIAN_POINT('Ctrl Pts',(13.1319317077644,-1.99369286349119,28.3870444358944)) ;
#58319=CARTESIAN_POINT('Ctrl Pts',(13.1312944893827,-1.98580782512015,28.3855437848765)) ;
#58320=CARTESIAN_POINT('Ctrl Pts',(13.1303498456158,-1.97404836901842,28.3833031411859)) ;
#58321=CARTESIAN_POINT('Ctrl Pts',(13.1300368390763,-1.97013990066385,28.3825579771459)) ;
#58322=CARTESIAN_POINT('Ctrl Pts',(13.1294151364984,-1.96234642378273,28.3810709967266)) ;
#58323=CARTESIAN_POINT('Ctrl Pts',(13.1291064388203,-1.95846141524282,28.3803291811031)) ;
#58324=CARTESIAN_POINT('Ctrl Pts',(13.128493818823,-1.95071083608938,28.3788477666453)) ;
#58325=CARTESIAN_POINT('Ctrl Pts',(13.1281736019689,-1.9466393373964,28.3780688156913)) ;
#58326=CARTESIAN_POINT('Ctrl Pts',(13.1275235722031,-1.93830268903959,28.3764712581725)) ;
#58327=CARTESIAN_POINT('Ctrl Pts',(13.1271936929168,-1.93403753869634,28.3756526821611)) ;
#58328=CARTESIAN_POINT('Ctrl Pts',(13.1267063464949,-1.92764007610111,28.3744214208619)) ;
#58329=CARTESIAN_POINT('Ctrl Pts',(13.1265451593027,-1.92550764565787,28.3740104297428)) ;
#58330=CARTESIAN_POINT('Ctrl Pts',(13.1262282666799,-1.92126713135282,28.3731914552007)) ;
#58331=CARTESIAN_POINT('Ctrl Pts',(13.1260725287054,-1.91915904703525,28.3727834867303)) ;
#58332=CARTESIAN_POINT('Ctrl Pts',(13.1258459404436,-1.91603336443895,28.3721765852679)) ;
#58333=CARTESIAN_POINT('Ctrl Pts',(13.1257715916756,-1.91499754803343,28.371975122494)) ;
#58334=CARTESIAN_POINT('Ctrl Pts',(13.1256259736314,-1.91294109847689,28.3715742295187)) ;
#58335=CARTESIAN_POINT('Ctrl Pts',(13.1255547020259,-1.91192046528262,28.3713748003851)) ;
#58336=CARTESIAN_POINT('Ctrl Pts',(13.1254163516264,-1.90989741714894,28.3709781506974)) ;
#58337=CARTESIAN_POINT('Ctrl Pts',(13.1253492373508,-1.90889500403652,28.370780946975)) ;
#58338=CARTESIAN_POINT('Ctrl Pts',(13.1252533348394,-1.90740733830955,28.3704865678484)) ;
#58339=CARTESIAN_POINT('Ctrl Pts',(13.1252221711284,-1.90691410922708,28.3703886751776)) ;
#58340=CARTESIAN_POINT('Ctrl Pts',(13.1251620394976,-1.90593335823539,28.3701931735045)) ;
#58341=CARTESIAN_POINT('Ctrl Pts',(13.1251330495881,-1.90544583567611,28.3700955745277)) ;
#58342=CARTESIAN_POINT('Ctrl Pts',(13.1250917024319,-1.90471219292145,28.3699476499174)) ;
#58343=CARTESIAN_POINT('Ctrl Pts',(13.1250773667852,-1.90445061424685,28.3698947196222)) ;
#58344=CARTESIAN_POINT('Ctrl Pts',(13.1250494265139,-1.90391520239999,28.3697857304192)) ;
#58345=CARTESIAN_POINT('Ctrl Pts',(13.1250358172642,-1.90364136904213,28.369729673609)) ;
#58346=CARTESIAN_POINT('Ctrl Pts',(13.1250110872508,-1.90309401527264,28.3696164799516)) ;
#58347=CARTESIAN_POINT('Ctrl Pts',(13.1249998825665,-1.90282053368396,28.3695593907705)) ;
#58348=CARTESIAN_POINT('Ctrl Pts',(13.1250156134575,-1.90163370102003,28.3692818656094)) ;
#58349=CARTESIAN_POINT('Ctrl Pts',(13.1250162587214,-1.9015850184438,28.3692704818312)) ;
#58350=CARTESIAN_POINT('Ctrl Pts',(13.1250169039853,-1.90153633586757,28.369259098053)) ;
#58351=CARTESIAN_POINT('',(25.9023611320436,-15.0366437072153,21.982218282509)) ;
#58352=CARTESIAN_POINT('',(25.8831717248497,-15.0366437072153,22.0048097991466)) ;
#58353=CARTESIAN_POINT('Origin',(-1.04106958514518,-21.6462763158693,-0.884292476110772)) ;
#58354=CARTESIAN_POINT('',(23.8238854240696,-1.9015362404957,20.2361906635364)) ;
#58355=CARTESIAN_POINT('Ctrl Pts',(23.8238854382361,-1.90153632942096,20.2361906752451)) ;
#58356=CARTESIAN_POINT('Ctrl Pts',(23.8238972397902,-1.90158489009019,20.236192282953)) ;
#58357=CARTESIAN_POINT('Ctrl Pts',(23.8241008025455,-1.90242250380941,20.2362200140004)) ;
#58358=CARTESIAN_POINT('Ctrl Pts',(23.8241800405353,-1.90282422716847,20.2362549662449)) ;
#58359=CARTESIAN_POINT('Ctrl Pts',(23.8242321897855,-1.90309850455843,20.2362811264257)) ;
#58360=CARTESIAN_POINT('Ctrl Pts',(23.8243349160092,-1.90364745004718,20.2363354225369)) ;
#58361=CARTESIAN_POINT('Ctrl Pts',(23.8243854246561,-1.90392207929595,20.2363636265058)) ;
#58362=CARTESIAN_POINT('Ctrl Pts',(23.8244832306668,-1.90445904680028,20.2364198915188)) ;
#58363=CARTESIAN_POINT('Ctrl Pts',(23.8245305247551,-1.90472138524212,20.2364479564785)) ;
#58364=CARTESIAN_POINT('Ctrl Pts',(23.824662358658,-1.90545718058384,20.2365276307242)) ;
#58365=CARTESIAN_POINT('Ctrl Pts',(23.8247488851777,-1.90594614106352,20.2365818501438)) ;
#58366=CARTESIAN_POINT('Ctrl Pts',(23.8249216560831,-1.90692978464094,20.2366924479152)) ;
#58367=CARTESIAN_POINT('Ctrl Pts',(23.8250078848634,-1.90742446839044,20.2367488448471)) ;
#58368=CARTESIAN_POINT('Ctrl Pts',(23.8252666035088,-1.90891652156313,20.2369205519908)) ;
#58369=CARTESIAN_POINT('Ctrl Pts',(23.8254391508834,-1.9099218908987,20.237038348235)) ;
#58370=CARTESIAN_POINT('Ctrl Pts',(23.8257853090816,-1.91195090507058,20.2372785226529)) ;
#58371=CARTESIAN_POINT('Ctrl Pts',(23.8259588941782,-1.91297454807863,20.2374009305311)) ;
#58372=CARTESIAN_POINT('Ctrl Pts',(23.8263072074963,-1.9150370619197,20.2376492615341)) ;
#58373=CARTESIAN_POINT('Ctrl Pts',(23.8264819340572,-1.91607593279612,20.2377751866276)) ;
#58374=CARTESIAN_POINT('Ctrl Pts',(23.8270075940328,-1.91921083239654,20.2381570567528)) ;
#58375=CARTESIAN_POINT('Ctrl Pts',(23.8273600354879,-1.92132513283609,20.2384170590922)) ;
#58376=CARTESIAN_POINT('Ctrl Pts',(23.8280664039129,-1.92557815084124,20.23894310934)) ;
#58377=CARTESIAN_POINT('Ctrl Pts',(23.8284203077438,-1.9277168688624,20.2392091846352)) ;
#58378=CARTESIAN_POINT('Ctrl Pts',(23.8294793530247,-1.93413319420295,20.2400106041034)) ;
#58379=CARTESIAN_POINT('Ctrl Pts',(23.8301818629063,-1.93841091972006,20.2405490841293)) ;
#58380=CARTESIAN_POINT('Ctrl Pts',(23.8315512366694,-1.94677214683963,20.2416060095999)) ;
#58381=CARTESIAN_POINT('Ctrl Pts',(23.8322180532724,-1.95085564912166,20.2421245109221)) ;
#58382=CARTESIAN_POINT('Ctrl Pts',(23.8334852560765,-1.95862918241561,20.2431141173015)) ;
#58383=CARTESIAN_POINT('Ctrl Pts',(23.8341192980611,-1.96252574910842,20.243611530175)) ;
#58384=CARTESIAN_POINT('Ctrl Pts',(23.8353894653667,-1.97034241205852,20.2446114143533)) ;
#58385=CARTESIAN_POINT('Ctrl Pts',(23.8360255895339,-1.97426250832905,20.2451138870204)) ;
#58386=CARTESIAN_POINT('Ctrl Pts',(23.837937434196,-1.98605694944873,20.2466281194029)) ;
#58387=CARTESIAN_POINT('Ctrl Pts',(23.8392166575569,-1.99396544619106,20.2476466572173)) ;
#58388=CARTESIAN_POINT('Ctrl Pts',(23.8417851342223,-2.00986743205398,20.2496990560114)) ;
#58389=CARTESIAN_POINT('Ctrl Pts',(23.843074368885,-2.01786092099999,20.2507329388821)) ;
#58390=CARTESIAN_POINT('Ctrl Pts',(23.8456627856708,-2.03392681721801,20.2528141859325)) ;
#58391=CARTESIAN_POINT('Ctrl Pts',(23.8469619672685,-2.04199922449445,20.2538615507317)) ;
#58392=CARTESIAN_POINT('Ctrl Pts',(23.8508738250851,-2.06632571772129,20.2570216762299)) ;
#58393=CARTESIAN_POINT('Ctrl Pts',(23.8535008798689,-2.0826890716089,20.2591523897619)) ;
#58394=CARTESIAN_POINT('Ctrl Pts',(23.858788182709,-2.11565860024936,20.2634522521349)) ;
#58395=CARTESIAN_POINT('Ctrl Pts',(23.8614483995056,-2.13226477520709,20.2656214378429)) ;
#58396=CARTESIAN_POINT('Ctrl Pts',(23.8667956808139,-2.1656713915056,20.2699902155389)) ;
#58397=CARTESIAN_POINT('Ctrl Pts',(23.869482733217,-2.18247182900697,20.2721898205565)) ;
#58398=CARTESIAN_POINT('Ctrl Pts',(23.8748768260301,-2.21621840381591,20.2766120092876)) ;
#58399=CARTESIAN_POINT('Ctrl Pts',(23.8775838649755,-2.23316454113134,20.2788345947272)) ;
#58400=CARTESIAN_POINT('Ctrl Pts',(23.8857242748928,-2.28414866676852,20.2855261523041)) ;
#58401=CARTESIAN_POINT('Ctrl Pts',(23.8911769860505,-2.31833236849097,20.2900188701501)) ;
#58402=CARTESIAN_POINT('Ctrl Pts',(23.902075238584,-2.38669989038716,20.2990127845743)) ;
#58403=CARTESIAN_POINT('Ctrl Pts',(23.9075207490885,-2.42088369689579,20.3035140131346)) ;
#58404=CARTESIAN_POINT('Ctrl Pts',(23.9183446729951,-2.48886293005225,20.3124714841742)) ;
#58405=CARTESIAN_POINT('Ctrl Pts',(23.9237230748093,-2.52265835674563,20.3169277403104)) ;
#58406=CARTESIAN_POINT('Ctrl Pts',(23.9396669654899,-2.62287936398345,20.3301497626395)) ;
#58407=CARTESIAN_POINT('Ctrl Pts',(23.9500412146539,-2.6881396713304,20.3387686942727)) ;
#58408=CARTESIAN_POINT('Ctrl Pts',(23.9707393778284,-2.81840077289416,20.3559829746962)) ;
#58409=CARTESIAN_POINT('Ctrl Pts',(23.9815899155693,-2.88672198231194,20.3650182794143)) ;
#58410=CARTESIAN_POINT('Ctrl Pts',(24.0033483989575,-3.02377678830098,20.3831529455601)) ;
#58411=CARTESIAN_POINT('Ctrl Pts',(24.014256319173,-3.09251038494502,20.3922523369516)) ;
#58412=CARTESIAN_POINT('Ctrl Pts',(24.03612921706,-3.23037665966399,20.410511341564)) ;
#58413=CARTESIAN_POINT('Ctrl Pts',(24.0470941844152,-3.29950933772532,20.4196709669254)) ;
#58414=CARTESIAN_POINT('Ctrl Pts',(24.0690802477411,-3.43816047088516,20.4380472859567)) ;
#58415=CARTESIAN_POINT('Ctrl Pts',(24.0801013423862,-3.50767892598712,20.4472639811866)) ;
#58416=CARTESIAN_POINT('Ctrl Pts',(24.1132469194986,-3.71679300160785,20.474995535766)) ;
#58417=CARTESIAN_POINT('Ctrl Pts',(24.1354537658879,-3.85694733178598,20.4935917805061)) ;
#58418=CARTESIAN_POINT('Ctrl Pts',(24.1800745931133,-4.13863946071678,20.5309820442909)) ;
#58419=CARTESIAN_POINT('Ctrl Pts',(24.2024885351756,-4.28017725954893,20.5497761090088)) ;
#58420=CARTESIAN_POINT('Ctrl Pts',(24.2475093203922,-4.56452990514295,20.5875447978751)) ;
#58421=CARTESIAN_POINT('Ctrl Pts',(24.2701161461079,-4.70734475099467,20.6065194422633)) ;
#58422=CARTESIAN_POINT('Ctrl Pts',(24.3155076113059,-4.99414506800992,20.6446330803387)) ;
#58423=CARTESIAN_POINT('Ctrl Pts',(24.3382922421449,-5.13813053918853,20.6637720842065)) ;
#58424=CARTESIAN_POINT('Ctrl Pts',(24.384023726511,-5.42716568699795,20.702198825054)) ;
#58425=CARTESIAN_POINT('Ctrl Pts',(24.4069705758003,-5.57221536362646,20.7214865670219)) ;
#58426=CARTESIAN_POINT('Ctrl Pts',(24.453010585758,-5.86327250296127,20.7601955450431)) ;
#58427=CARTESIAN_POINT('Ctrl Pts',(24.4761037456608,-6.0092799656689,20.7796167819971)) ;
#58428=CARTESIAN_POINT('Ctrl Pts',(24.5455785124947,-6.44857940435679,20.8380582440759)) ;
#58429=CARTESIAN_POINT('Ctrl Pts',(24.5921554554228,-6.74314842620376,20.8772561613807)) ;
#58430=CARTESIAN_POINT('Ctrl Pts',(24.6856996519804,-7.33484057012121,20.9560078084074)) ;
#58431=CARTESIAN_POINT('Ctrl Pts',(24.7326668806052,-7.63196369222536,20.9955615675779)) ;
#58432=CARTESIAN_POINT('Ctrl Pts',(24.82685976589,-8.22791267989474,21.0749083918998)) ;
#58433=CARTESIAN_POINT('Ctrl Pts',(24.8740854101562,-8.52673854545668,21.1147014716412)) ;
#58434=CARTESIAN_POINT('Ctrl Pts',(24.9686625303249,-9.12524166409269,21.1944112711994)) ;
#58435=CARTESIAN_POINT('Ctrl Pts',(25.0160140004293,-9.42491891717367,21.2343279978436)) ;
#58436=CARTESIAN_POINT('Ctrl Pts',(25.1580575855592,-10.3239507246136,21.3540909375572)) ;
#58437=CARTESIAN_POINT('Ctrl Pts',(25.2527389752251,-10.9233053117369,21.4339497879505)) ;
#58438=CARTESIAN_POINT('Ctrl Pts',(25.4410055391706,-12.1152037164723,21.5927839145526)) ;
#58439=CARTESIAN_POINT('Ctrl Pts',(25.5345906632723,-12.7077475341359,21.6717592498504)) ;
#58440=CARTESIAN_POINT('Ctrl Pts',(25.7201261119685,-13.8825790586843,21.8283605922029)) ;
#58441=CARTESIAN_POINT('Ctrl Pts',(25.8120639293555,-14.4647882730915,21.9059762674555)) ;
#58442=CARTESIAN_POINT('Ctrl Pts',(25.9023611320477,-15.0366437072153,21.9822182825043)) ;
#58443=CARTESIAN_POINT('Ctrl Pts',(25.8831717248466,-15.0366437072153,22.0048097991503)) ;
#58444=CARTESIAN_POINT('Ctrl Pts',(25.8826584335355,-15.0333766938331,22.0043711940518)) ;
#58445=CARTESIAN_POINT('Ctrl Pts',(25.8821450893183,-15.0301093425198,22.0039325433645)) ;
#58446=CARTESIAN_POINT('Ctrl Pts',(25.7922804814445,-14.458135719157,21.9271435098704)) ;
#58447=CARTESIAN_POINT('Ctrl Pts',(25.701329838895,-13.8792135356312,21.8494149308997)) ;
#58448=CARTESIAN_POINT('Ctrl Pts',(25.5173038766047,-12.7077475344918,21.6921108285546)) ;
#58449=CARTESIAN_POINT('Ctrl Pts',(25.4242285328903,-12.1152037168811,21.612535333405)) ;
#58450=CARTESIAN_POINT('Ctrl Pts',(25.237028663492,-10.923305312252,21.4524453969325)) ;
#58451=CARTESIAN_POINT('Ctrl Pts',(25.1429040876147,-10.323950725182,21.3719310146869)) ;
#58452=CARTESIAN_POINT('Ctrl Pts',(25.0017387475006,-9.42491891782229,21.2511341250345)) ;
#58453=CARTESIAN_POINT('Ctrl Pts',(24.9546872475854,-9.12524166476805,21.2108642461908)) ;
#58454=CARTESIAN_POINT('Ctrl Pts',(24.8607266279542,-8.52673854618542,21.1304286461072)) ;
#58455=CARTESIAN_POINT('Ctrl Pts',(24.8138175024392,-8.22791268065011,21.090262931693)) ;
#58456=CARTESIAN_POINT('Ctrl Pts',(24.7202772386849,-7.63196369303388,21.0101477819253)) ;
#58457=CARTESIAN_POINT('Ctrl Pts',(24.6736460880534,-7.33484057095624,20.970198361162)) ;
#58458=CARTESIAN_POINT('Ctrl Pts',(24.5807981071967,-6.74314842709155,20.8906270656642)) ;
#58459=CARTESIAN_POINT('Ctrl Pts',(24.5345812519569,-6.44857940527084,20.8510052203684)) ;
#58460=CARTESIAN_POINT('Ctrl Pts',(24.4656699006792,-6.00927996662213,20.7919004542311)) ;
#58461=CARTESIAN_POINT('Ctrl Pts',(24.4427684514381,-5.86327250392753,20.7722535180421)) ;
#58462=CARTESIAN_POINT('Ctrl Pts',(24.3971209605381,-5.57221536461865,20.73308243087)) ;
#58463=CARTESIAN_POINT('Ctrl Pts',(24.3743749181146,-5.42716568800309,20.7135582807878)) ;
#58464=CARTESIAN_POINT('Ctrl Pts',(24.3290558602293,-5.13813054021944,20.6746459939591)) ;
#58465=CARTESIAN_POINT('Ctrl Pts',(24.306482840531,-4.99414506905368,20.6552578622012)) ;
#58466=CARTESIAN_POINT('Ctrl Pts',(24.2615277697454,-4.707344752064,20.616630460914)) ;
#58467=CARTESIAN_POINT('Ctrl Pts',(24.2391457100099,-4.56452990622502,20.5973912015613)) ;
#58468=CARTESIAN_POINT('Ctrl Pts',(24.1945910136002,-4.28017726065633,20.5590737905393)) ;
#58469=CARTESIAN_POINT('Ctrl Pts',(24.1724183597702,-4.1386394618368,20.539995659358)) ;
#58470=CARTESIAN_POINT('Ctrl Pts',(24.1283018092702,-3.85694733293112,20.5020117151243)) ;
#58471=CARTESIAN_POINT('Ctrl Pts',(24.1063578737995,-3.71679300276549,20.4831059477265)) ;
#58472=CARTESIAN_POINT('Ctrl Pts',(24.0736292825901,-3.50767892716341,20.4548834793968)) ;
#58473=CARTESIAN_POINT('Ctrl Pts',(24.062750988598,-3.43816047206766,20.4454986662434)) ;
#58474=CARTESIAN_POINT('Ctrl Pts',(24.0410598003719,-3.29950933892018,20.4267751934111)) ;
#58475=CARTESIAN_POINT('Ctrl Pts',(24.0302469048117,-3.23037666086501,20.417436535294)) ;
#58476=CARTESIAN_POINT('Ctrl Pts',(24.0086897936963,-3.09251038615833,20.3988057577573)) ;
#58477=CARTESIAN_POINT('Ctrl Pts',(23.9979455678243,-3.02377678952043,20.3895136504882)) ;
#58478=CARTESIAN_POINT('Ctrl Pts',(23.9765296674114,-2.8867219835436,20.3709756644882)) ;
#58479=CARTESIAN_POINT('Ctrl Pts',(23.9658579674197,-2.81840077413193,20.3617298156971)) ;
#58480=CARTESIAN_POINT('Ctrl Pts',(23.9455218687335,-2.68813967234734,20.3440892799348)) ;
#58481=CARTESIAN_POINT('Ctrl Pts',(23.9353381116194,-2.62287936476213,20.3352460836472)) ;
#58482=CARTESIAN_POINT('Ctrl Pts',(23.9197108347794,-2.52265835715845,20.321651314572)) ;
#58483=CARTESIAN_POINT('Ctrl Pts',(23.9144431544326,-2.48886293034172,20.317064707008)) ;
#58484=CARTESIAN_POINT('Ctrl Pts',(23.9038525683769,-2.42088369693709,20.3078325293342)) ;
#58485=CARTESIAN_POINT('Ctrl Pts',(23.8985296510698,-2.38669989030367,20.3031869728647)) ;
#58486=CARTESIAN_POINT('Ctrl Pts',(23.8878910766815,-2.31833236815792,20.2938873416141)) ;
#58487=CARTESIAN_POINT('Ctrl Pts',(23.8825753930318,-2.28414866631064,20.2892333024744)) ;
#58488=CARTESIAN_POINT('Ctrl Pts',(23.8746550147401,-2.23316454048736,20.2822827035826)) ;
#58489=CARTESIAN_POINT('Ctrl Pts',(23.8720237583063,-2.21621840311006,20.2799709000535)) ;
#58490=CARTESIAN_POINT('Ctrl Pts',(23.8667871580548,-2.18247182817792,20.2753632967057)) ;
#58491=CARTESIAN_POINT('Ctrl Pts',(23.8641818127718,-2.16567139061522,20.2730674986103)) ;
#58492=CARTESIAN_POINT('Ctrl Pts',(23.8590054932055,-2.13226477419477,20.2684974491529)) ;
#58493=CARTESIAN_POINT('Ctrl Pts',(23.8564345080252,-2.11565859917642,20.2662232118455)) ;
#58494=CARTESIAN_POINT('Ctrl Pts',(23.8513358993637,-2.08268907041563,20.2617012014733)) ;
#58495=CARTESIAN_POINT('Ctrl Pts',(23.8488082445528,-2.06632571646822,20.2594534652275)) ;
#58496=CARTESIAN_POINT('Ctrl Pts',(23.8450568807162,-2.04199922315259,20.2561043915805)) ;
#58497=CARTESIAN_POINT('Ctrl Pts',(23.8438131291648,-2.03392681584675,20.2549917694768)) ;
#58498=CARTESIAN_POINT('Ctrl Pts',(23.8413405401307,-2.01786091957008,20.2527741594364)) ;
#58499=CARTESIAN_POINT('Ctrl Pts',(23.8401117021167,-2.00986743059477,20.2516691721247)) ;
#58500=CARTESIAN_POINT('Ctrl Pts',(23.8376708072609,-1.99396544467382,20.2494665723942)) ;
#58501=CARTESIAN_POINT('Ctrl Pts',(23.8364587318387,-1.98605694790282,20.2483689819058)) ;
#58502=CARTESIAN_POINT('Ctrl Pts',(23.8346551451098,-1.97426250674009,20.2467272984177)) ;
#58503=CARTESIAN_POINT('Ctrl Pts',(23.834056378304,-1.97034241045512,20.2461808452601)) ;
#58504=CARTESIAN_POINT('Ctrl Pts',(23.8328641758709,-1.9625257474765,20.245089173729)) ;
#58505=CARTESIAN_POINT('Ctrl Pts',(23.8322707390673,-1.9586291807694,20.2445439567363)) ;
#58506=CARTESIAN_POINT('Ctrl Pts',(23.8310891586813,-1.95085564771088,20.2434535479286)) ;
#58507=CARTESIAN_POINT('Ctrl Pts',(23.8304696089611,-1.94677214569123,20.2428793998139)) ;
#58508=CARTESIAN_POINT('Ctrl Pts',(23.8292050669332,-1.93841091910833,20.2416990570549)) ;
#58509=CARTESIAN_POINT('Ctrl Pts',(23.8285600271676,-1.93413319386599,20.2410929180656)) ;
#58510=CARTESIAN_POINT('Ctrl Pts',(23.8275978307824,-1.92771686893724,20.2401774793944)) ;
#58511=CARTESIAN_POINT('Ctrl Pts',(23.8272780053549,-1.92557815105288,20.2398712839446)) ;
#58512=CARTESIAN_POINT('Ctrl Pts',(23.8266446073645,-1.92132513332065,20.239259326347)) ;
#58513=CARTESIAN_POINT('Ctrl Pts',(23.8263310115037,-1.91921083301692,20.238953591482)) ;
#58514=CARTESIAN_POINT('Ctrl Pts',(23.8258691296441,-1.91607593361768,20.2384966360183)) ;
#58515=CARTESIAN_POINT('Ctrl Pts',(23.8257165958113,-1.91503706280771,20.2383445836466)) ;
#58516=CARTESIAN_POINT('Ctrl Pts',(23.8254151853864,-1.912974549099,20.2380410343312)) ;
#58517=CARTESIAN_POINT('Ctrl Pts',(23.8252663071272,-1.91195090615706,20.2378895393365)) ;
#58518=CARTESIAN_POINT('Ctrl Pts',(23.8249732944991,-1.90992189211548,20.2375867971581)) ;
#58519=CARTESIAN_POINT('Ctrl Pts',(23.8248291348807,-1.90891652284042,20.237435580283)) ;
#58520=CARTESIAN_POINT('Ctrl Pts',(23.8246178337073,-1.90742446976331,20.237208049006)) ;
#58521=CARTESIAN_POINT('Ctrl Pts',(23.8245482295593,-1.90692978604951,20.2371320800555)) ;
#58522=CARTESIAN_POINT('Ctrl Pts',(23.8244111375301,-1.90594614253486,20.2369794778838)) ;
#58523=CARTESIAN_POINT('Ctrl Pts',(23.8243436339605,-1.90545718208726,20.2369028629261)) ;
#58524=CARTESIAN_POINT('Ctrl Pts',(23.8242436809488,-1.90472138673829,20.2367856555915)) ;
#58525=CARTESIAN_POINT('Ctrl Pts',(23.8242083343078,-1.90445904825293,20.2367435249956)) ;
#58526=CARTESIAN_POINT('Ctrl Pts',(23.8241369872358,-1.90392208066598,20.2366561100854)) ;
#58527=CARTESIAN_POINT('Ctrl Pts',(23.8241009834238,-1.90364745137547,20.2366108296914)) ;
#58528=CARTESIAN_POINT('Ctrl Pts',(23.8240307833116,-1.90309850580222,20.2365182408545)) ;
#58529=CARTESIAN_POINT('Ctrl Pts',(23.823996530879,-1.9028242283647,20.236471010896)) ;
#58530=CARTESIAN_POINT('Ctrl Pts',(23.8238938369784,-1.90163369618714,20.2362118689699)) ;
#58531=CARTESIAN_POINT('Ctrl Pts',(23.8238896376073,-1.90158501280405,20.2362012721075)) ;
#58532=CARTESIAN_POINT('Ctrl Pts',(23.8238854382361,-1.90153632942096,20.2361906752451)) ;
#58533=CARTESIAN_POINT('',(32.7384401598282,-15.0366437072153,9.07440183902105)) ;
#58534=CARTESIAN_POINT('',(32.7305102571632,-15.0366437072153,9.10296276716598)) ;
#58535=CARTESIAN_POINT('Origin',(-1.31615393895548,-21.6462763158694,-0.365428342349794)) ;
#58536=CARTESIAN_POINT('',(30.1189287294544,-1.90153624409553,8.36247938752316)) ;
#58537=CARTESIAN_POINT('Ctrl Pts',(30.1189287479468,-1.90153633662063,8.36247939239298)) ;
#58538=CARTESIAN_POINT('Ctrl Pts',(30.1189401385585,-1.90158489480086,8.36247587712654)) ;
#58539=CARTESIAN_POINT('Ctrl Pts',(30.1191353360247,-1.9024170216435,8.36241563706908)) ;
#58540=CARTESIAN_POINT('Ctrl Pts',(30.1192214019803,-1.90281621653025,8.36241402382017)) ;
#58541=CARTESIAN_POINT('Ctrl Pts',(30.1192793604866,-1.90308876899224,8.36241581627159)) ;
#58542=CARTESIAN_POINT('Ctrl Pts',(30.1193946823344,-1.90363426439912,8.36242184640268)) ;
#58543=CARTESIAN_POINT('Ctrl Pts',(30.1194520122693,-1.9039071685372,8.36242617442493)) ;
#58544=CARTESIAN_POINT('Ctrl Pts',(30.1195637149721,-1.90444076412458,8.36243604721865)) ;
#58545=CARTESIAN_POINT('Ctrl Pts',(30.119618086374,-1.90470145576606,8.36244159705791)) ;
#58546=CARTESIAN_POINT('Ctrl Pts',(30.1197702395338,-1.9054325846776,8.3624583701444)) ;
#58547=CARTESIAN_POINT('Ctrl Pts',(30.1198709015847,-1.90591842777427,8.36247112013853)) ;
#58548=CARTESIAN_POINT('Ctrl Pts',(30.1200728704408,-1.90689580028702,8.36249869047458)) ;
#58549=CARTESIAN_POINT('Ctrl Pts',(30.1201741709541,-1.90738733034979,8.36251353397729)) ;
#58550=CARTESIAN_POINT('Ctrl Pts',(30.1204791499426,-1.90886987163284,8.36256032589338)) ;
#58551=CARTESIAN_POINT('Ctrl Pts',(30.1206839159759,-1.90986883193724,8.36259449775017)) ;
#58552=CARTESIAN_POINT('Ctrl Pts',(30.1210963164293,-1.91188491186432,8.3626665380976)) ;
#58553=CARTESIAN_POINT('Ctrl Pts',(30.1213039399985,-1.91290202966046,8.362704444259)) ;
#58554=CARTESIAN_POINT('Ctrl Pts',(30.1217216830286,-1.91495139626056,8.3627829555271)) ;
#58555=CARTESIAN_POINT('Ctrl Pts',(30.1219318017981,-1.91598364510872,8.3628235631576)) ;
#58556=CARTESIAN_POINT('Ctrl Pts',(30.122565199736,-1.91909856243828,8.36294846757877)) ;
#58557=CARTESIAN_POINT('Ctrl Pts',(30.122991529876,-1.92119938645565,8.36303580047106)) ;
#58558=CARTESIAN_POINT('Ctrl Pts',(30.123848049114,-1.92542529670216,8.36321530951135)) ;
#58559=CARTESIAN_POINT('Ctrl Pts',(30.1242782287435,-1.92755038338676,8.36330752011368)) ;
#58560=CARTESIAN_POINT('Ctrl Pts',(30.1255676923907,-1.93392581469217,8.36358815687788)) ;
#58561=CARTESIAN_POINT('Ctrl Pts',(30.1264259082826,-1.93817627749712,8.36378052137526)) ;
#58562=CARTESIAN_POINT('Ctrl Pts',(30.1281018297584,-1.94648421837564,8.36416207931785)) ;
#58563=CARTESIAN_POINT('Ctrl Pts',(30.1289195159722,-1.95054169712835,8.36435134305257)) ;
#58564=CARTESIAN_POINT('Ctrl Pts',(30.1304751568044,-1.95826546741375,8.36471485519461)) ;
#58565=CARTESIAN_POINT('Ctrl Pts',(30.131254439218,-1.96213697736357,8.36489878055514)) ;
#58566=CARTESIAN_POINT('Ctrl Pts',(30.1328169909108,-1.96990337558838,8.36527033107019)) ;
#58567=CARTESIAN_POINT('Ctrl Pts',(30.1336002597047,-1.97379826387693,8.36545795798234)) ;
#58568=CARTESIAN_POINT('Ctrl Pts',(30.1359560375186,-1.98551686150977,8.36602554379915)) ;
#58569=CARTESIAN_POINT('Ctrl Pts',(30.1375345305293,-1.99337450320726,8.36641016223176)) ;
#58570=CARTESIAN_POINT('Ctrl Pts',(30.1407069492262,-2.00917423257069,8.36718904807286)) ;
#58571=CARTESIAN_POINT('Ctrl Pts',(30.1423008672139,-2.01711632006207,8.36758334307332)) ;
#58572=CARTESIAN_POINT('Ctrl Pts',(30.1455032942253,-2.03307890599031,8.36837995145598)) ;
#58573=CARTESIAN_POINT('Ctrl Pts',(30.147111803032,-2.04109940443164,8.36878226562087)) ;
#58574=CARTESIAN_POINT('Ctrl Pts',(30.1519577546552,-2.06526946862637,8.36999950998952)) ;
#58575=CARTESIAN_POINT('Ctrl Pts',(30.1552156492126,-2.08152759979058,8.37082464380675)) ;
#58576=CARTESIAN_POINT('Ctrl Pts',(30.161777398163,-2.11428512181414,8.37249574630261)) ;
#58577=CARTESIAN_POINT('Ctrl Pts',(30.1650812397105,-2.13078451287836,8.37334176140317)) ;
#58578=CARTESIAN_POINT('Ctrl Pts',(30.1717258126984,-2.16397631245258,8.37505002748482)) ;
#58579=CARTESIAN_POINT('Ctrl Pts',(30.175066538635,-2.18066871712369,8.37591229532295)) ;
#58580=CARTESIAN_POINT('Ctrl Pts',(30.181775597047,-2.21419828956957,8.37764922719805)) ;
#58581=CARTESIAN_POINT('Ctrl Pts',(30.1851439289196,-2.23103545735225,8.37852389341123)) ;
#58582=CARTESIAN_POINT('Ctrl Pts',(30.1952762466849,-2.28169173768762,8.38116132325939)) ;
#58583=CARTESIAN_POINT('Ctrl Pts',(30.2020675740848,-2.31565562693768,8.38293744815023)) ;
#58584=CARTESIAN_POINT('Ctrl Pts',(30.2156472914047,-2.38358352388148,8.38650036927385)) ;
#58585=CARTESIAN_POINT('Ctrl Pts',(30.2224356667714,-2.41754751791137,8.38828720736706)) ;
#58586=CARTESIAN_POINT('Ctrl Pts',(30.2359331378935,-2.48508962397494,8.39184833848321)) ;
#58587=CARTESIAN_POINT('Ctrl Pts',(30.2426422288818,-2.51866773605419,8.393622648711)) ;
#58588=CARTESIAN_POINT('Ctrl Pts',(30.2625357546531,-2.61824429305133,8.39889310449012)) ;
#58589=CARTESIAN_POINT('Ctrl Pts',(30.2754864731247,-2.68308495837333,8.40233666363732)) ;
#58590=CARTESIAN_POINT('Ctrl Pts',(30.3013241640144,-2.81246585314203,8.40922129508462)) ;
#58591=CARTESIAN_POINT('Ctrl Pts',(30.314869539521,-2.8803050131185,8.41283935709915)) ;
#58592=CARTESIAN_POINT('Ctrl Pts',(30.3420387230831,-3.01639281064624,8.4201093040508)) ;
#58593=CARTESIAN_POINT('Ctrl Pts',(30.3556625207004,-3.08464144827008,8.42376122663904)) ;
#58594=CARTESIAN_POINT('Ctrl Pts',(30.3829866355126,-3.22153498923157,8.43109557879761)) ;
#58595=CARTESIAN_POINT('Ctrl Pts',(30.3966869484653,-3.2901798925557,8.43477802363559)) ;
#58596=CARTESIAN_POINT('Ctrl Pts',(30.4241619433415,-3.42785275438354,8.44217096126773)) ;
#58597=CARTESIAN_POINT('Ctrl Pts',(30.437936624721,-3.49688071289066,8.44588145602008)) ;
#58598=CARTESIAN_POINT('Ctrl Pts',(30.4793687882844,-3.70451935672761,8.45705207429126)) ;
#58599=CARTESIAN_POINT('Ctrl Pts',(30.5071344189108,-3.84368480971854,8.46455122679989)) ;
#58600=CARTESIAN_POINT('Ctrl Pts',(30.5629347866261,-4.12338942313901,8.47964145340705)) ;
#58601=CARTESIAN_POINT('Ctrl Pts',(30.5909695077761,-4.26392858364792,8.48723258497366)) ;
#58602=CARTESIAN_POINT('Ctrl Pts',(30.6472880555991,-4.54627494231513,8.50249717923564)) ;
#58603=CARTESIAN_POINT('Ctrl Pts',(30.6755718749747,-4.68808213956468,8.51017066751273)) ;
#58604=CARTESIAN_POINT('Ctrl Pts',(30.7323682666508,-4.97285889995491,8.52559164977468)) ;
#58605=CARTESIAN_POINT('Ctrl Pts',(30.7608808353976,-5.11582846311061,8.53333915657121)) ;
#58606=CARTESIAN_POINT('Ctrl Pts',(30.8181141662874,-5.40282428630946,8.54890059787569)) ;
#58607=CARTESIAN_POINT('Ctrl Pts',(30.8468349266871,-5.54685054635029,8.55671453866051)) ;
#58608=CARTESIAN_POINT('Ctrl Pts',(30.9044639496286,-5.8358540948004,8.57240174475533)) ;
#58609=CARTESIAN_POINT('Ctrl Pts',(30.9333722118556,-5.98083138321102,8.58027501119716)) ;
#58610=CARTESIAN_POINT('Ctrl Pts',(31.0203470861221,-6.41703128872674,8.60397360662014)) ;
#58611=CARTESIAN_POINT('Ctrl Pts',(31.0786638052327,-6.70952194142243,8.61987765788934)) ;
#58612=CARTESIAN_POINT('Ctrl Pts',(31.1957973094387,-7.29703932648007,8.65184374517469)) ;
#58613=CARTESIAN_POINT('Ctrl Pts',(31.2546140842477,-7.59206605887567,8.6679058182651)) ;
#58614=CARTESIAN_POINT('Ctrl Pts',(31.3725802794297,-8.18381025341842,8.70013793087388)) ;
#58615=CARTESIAN_POINT('Ctrl Pts',(31.431729694701,-8.48052771556226,8.71630798876412)) ;
#58616=CARTESIAN_POINT('Ctrl Pts',(31.5501934566931,-9.07480802049958,8.74870711107049)) ;
#58617=CARTESIAN_POINT('Ctrl Pts',(31.6095078010264,-9.37237086329999,8.76493618408882)) ;
#58618=CARTESIAN_POINT('Ctrl Pts',(31.7874463810178,-10.2650594398744,8.81363947865428)) ;
#58619=CARTESIAN_POINT('Ctrl Pts',(31.9060662026799,-10.8601852063993,8.84612962326616)) ;
#58620=CARTESIAN_POINT('Ctrl Pts',(32.1419495440396,-12.04367402468,8.91077083857098)) ;
#58621=CARTESIAN_POINT('Ctrl Pts',(32.2592130430851,-12.6320370764873,8.94292198368229)) ;
#58622=CARTESIAN_POINT('Ctrl Pts',(32.4910381898069,-13.7952376555442,9.00650732543321)) ;
#58623=CARTESIAN_POINT('Ctrl Pts',(32.6124966123284,-14.4046812756116,9.03983394617206)) ;
#58624=CARTESIAN_POINT('Ctrl Pts',(32.7316800387708,-15.0027225758531,9.07254634846712)) ;
#58625=CARTESIAN_POINT('Ctrl Pts',(32.7384401599474,-15.0366437072151,9.07440183859066)) ;
#58626=CARTESIAN_POINT('Ctrl Pts',(32.7305102570438,-15.0366437072151,9.10296276759541)) ;
#58627=CARTESIAN_POINT('Ctrl Pts',(32.7237611936063,-15.0027225758262,9.10106745107396)) ;
#58628=CARTESIAN_POINT('Ctrl Pts',(32.7170046769115,-14.9687639419481,9.09917000900167)) ;
#58629=CARTESIAN_POINT('Ctrl Pts',(32.5978878264882,-14.3700751826827,9.06571767526185)) ;
#58630=CARTESIAN_POINT('Ctrl Pts',(32.4835188253644,-13.795237655408,9.03358962842959)) ;
#58631=CARTESIAN_POINT('Ctrl Pts',(32.2520961165689,-12.6320370762946,8.96855483622168)) ;
#58632=CARTESIAN_POINT('Ctrl Pts',(32.1350423990285,-12.0436740244586,8.9356481263927)) ;
#58633=CARTESIAN_POINT('Ctrl Pts',(31.8995980373515,-10.8601852061203,8.86942584911774)) ;
#58634=CARTESIAN_POINT('Ctrl Pts',(31.7812073725445,-10.2650594395664,8.83611035608409)) ;
#58635=CARTESIAN_POINT('Ctrl Pts',(31.6036302519827,-9.37237086294862,8.78610520227785)) ;
#58636=CARTESIAN_POINT('Ctrl Pts',(31.5444393691944,-9.07480802013375,8.76943146095126)) ;
#58637=CARTESIAN_POINT('Ctrl Pts',(31.4262293521357,-8.4805277151675,8.73611843196877)) ;
#58638=CARTESIAN_POINT('Ctrl Pts',(31.3672102154762,-8.18381025300921,8.71947915291443)) ;
#58639=CARTESIAN_POINT('Ctrl Pts',(31.2495126446032,-7.59206605843769,8.68627954296213)) ;
#58640=CARTESIAN_POINT('Ctrl Pts',(31.1908342052898,-7.29703932602775,8.66971923043497)) ;
#58641=CARTESIAN_POINT('Ctrl Pts',(31.0739872820367,-6.7095219409415,8.63672097181969)) ;
#58642=CARTESIAN_POINT('Ctrl Pts',(31.0158187877964,-6.41703128823159,8.62028306280528)) ;
#58643=CARTESIAN_POINT('Ctrl Pts',(30.9290758403507,-5.98083138269464,8.59574914245178)) ;
#58644=CARTESIAN_POINT('Ctrl Pts',(30.9002464955277,-5.83585409427698,8.58759164120349)) ;
#58645=CARTESIAN_POINT('Ctrl Pts',(30.8427790540515,-5.5468505458128,8.57132247125625)) ;
#58646=CARTESIAN_POINT('Ctrl Pts',(30.8141409570852,-5.40282428576498,8.56321080368639)) ;
#58647=CARTESIAN_POINT('Ctrl Pts',(30.7570774057057,-5.11582846255216,8.54703787183943)) ;
#58648=CARTESIAN_POINT('Ctrl Pts',(30.7286519495495,-4.9728588993895,8.53897661384235)) ;
#58649=CARTESIAN_POINT('Ctrl Pts',(30.672035206872,-4.68808213898542,8.52290859435385)) ;
#58650=CARTESIAN_POINT('Ctrl Pts',(30.6438439167901,-4.54627494172898,8.51490184567515)) ;
#58651=CARTESIAN_POINT('Ctrl Pts',(30.5877172444839,-4.26392858304801,8.49894617824804)) ;
#58652=CARTESIAN_POINT('Ctrl Pts',(30.5597818553244,-4.12338942253229,8.49099728517994)) ;
#58653=CARTESIAN_POINT('Ctrl Pts',(30.504189085279,-3.8436848090982,8.47515935932977)) ;
#58654=CARTESIAN_POINT('Ctrl Pts',(30.4765316884238,-3.70451935610049,8.46727038400322)) ;
#58655=CARTESIAN_POINT('Ctrl Pts',(30.4352711864115,-3.49688071225345,8.45548149669456)) ;
#58656=CARTESIAN_POINT('Ctrl Pts',(30.4215552919392,-3.42785275374295,8.45155927063588)) ;
#58657=CARTESIAN_POINT('Ctrl Pts',(30.3942016879009,-3.29017989190842,8.44372912271403)) ;
#58658=CARTESIAN_POINT('Ctrl Pts',(30.3805639777915,-3.22153498858096,8.43982120280978)) ;
#58659=CARTESIAN_POINT('Ctrl Pts',(30.3533698603856,-3.08464144761279,8.43201864230363)) ;
#58660=CARTESIAN_POINT('Ctrl Pts',(30.3398134488531,-3.01639280998565,8.4281240169703)) ;
#58661=CARTESIAN_POINT('Ctrl Pts',(30.3127852897537,-2.88030501245129,8.4203461458039)) ;
#58662=CARTESIAN_POINT('Ctrl Pts',(30.2993135317183,-2.8124658524715,8.41646293761831)) ;
#58663=CARTESIAN_POINT('Ctrl Pts',(30.2736249225872,-2.68308495780993,8.40904136228668)) ;
#58664=CARTESIAN_POINT('Ctrl Pts',(30.2607526663507,-2.61824429260388,8.40531520779866)) ;
#58665=CARTESIAN_POINT('Ctrl Pts',(30.2409895522636,-2.51866773578479,8.39957505172038)) ;
#58666=CARTESIAN_POINT('Ctrl Pts',(30.2343260670344,-2.48508962376557,8.39763648444005)) ;
#58667=CARTESIAN_POINT('Ctrl Pts',(30.2209247071845,-2.41754751782276,8.39372919189985)) ;
#58668=CARTESIAN_POINT('Ctrl Pts',(30.2141868277782,-2.38358352385361,8.39176048384098)) ;
#58669=CARTESIAN_POINT('Ctrl Pts',(30.2007140718384,-2.31565562703126,8.3878123227368)) ;
#58670=CARTESIAN_POINT('Ctrl Pts',(30.1939791861965,-2.28169173784196,8.38583291305283)) ;
#58671=CARTESIAN_POINT('Ctrl Pts',(30.1839374998947,-2.23103545759718,8.38286905824464)) ;
#58672=CARTESIAN_POINT('Ctrl Pts',(30.1806003830226,-2.21419828984458,8.38188196578363)) ;
#58673=CARTESIAN_POINT('Ctrl Pts',(30.1739561962611,-2.18066871745867,8.37991138738601)) ;
#58674=CARTESIAN_POINT('Ctrl Pts',(30.1706491257674,-2.16397631281742,8.37892790362093)) ;
#58675=CARTESIAN_POINT('Ctrl Pts',(30.1640749725642,-2.13078451330256,8.37696600844302)) ;
#58676=CARTESIAN_POINT('Ctrl Pts',(30.1608078858836,-2.11428512226784,8.37598761429832)) ;
#58677=CARTESIAN_POINT('Ctrl Pts',(30.1543238608813,-2.08152760030284,8.37403657548676)) ;
#58678=CARTESIAN_POINT('Ctrl Pts',(30.1511069096249,-2.06526946916755,8.37306397724891)) ;
#58679=CARTESIAN_POINT('Ctrl Pts',(30.1463270661805,-2.04109940501605,8.37160863277271)) ;
#58680=CARTESIAN_POINT('Ctrl Pts',(30.1447413892533,-2.03307890658913,8.37112408562097)) ;
#58681=CARTESIAN_POINT('Ctrl Pts',(30.1415866721682,-2.0171163206894,8.37015564163571)) ;
#58682=CARTESIAN_POINT('Ctrl Pts',(30.1400176317903,-2.0091742332121,8.36967174559335)) ;
#58683=CARTESIAN_POINT('Ctrl Pts',(30.1368977644696,-1.99337450387689,8.36870358682289)) ;
#58684=CARTESIAN_POINT('Ctrl Pts',(30.1353469298989,-1.9855168621936,8.36821935170382)) ;
#58685=CARTESIAN_POINT('Ctrl Pts',(30.1330357437207,-1.97379826458171,8.3674911613461)) ;
#58686=CARTESIAN_POINT('Ctrl Pts',(30.1322678624578,-1.96990337630014,8.3672481135615)) ;
#58687=CARTESIAN_POINT('Ctrl Pts',(30.1307374245282,-1.96213697808921,8.3667608997356)) ;
#58688=CARTESIAN_POINT('Ctrl Pts',(30.1299748673744,-1.95826546814638,8.36651673543883)) ;
#58689=CARTESIAN_POINT('Ctrl Pts',(30.1284544952475,-1.95054169771239,8.36602619678552)) ;
#58690=CARTESIAN_POINT('Ctrl Pts',(30.1276562792614,-1.94648421879626,8.36576680750224)) ;
#58691=CARTESIAN_POINT('Ctrl Pts',(30.1260235401834,-1.93817627758352,8.36522972036066)) ;
#58692=CARTESIAN_POINT('Ctrl Pts',(30.1251889974474,-1.93392581460767,8.36495209272972)) ;
#58693=CARTESIAN_POINT('Ctrl Pts',(30.1239394278513,-1.92755038304578,8.3645277703813)) ;
#58694=CARTESIAN_POINT('Ctrl Pts',(30.1235232858035,-1.92542529627582,8.36438500091296)) ;
#58695=CARTESIAN_POINT('Ctrl Pts',(30.122696824537,-1.92119938585934,8.36409723271207)) ;
#58696=CARTESIAN_POINT('Ctrl Pts',(30.1222864956636,-1.91909856175708,8.36395226840083)) ;
#58697=CARTESIAN_POINT('Ctrl Pts',(30.1216793691147,-1.91598364430227,8.36373274289128)) ;
#58698=CARTESIAN_POINT('Ctrl Pts',(30.1214783919202,-1.9149513954132,8.36365921025158)) ;
#58699=CARTESIAN_POINT('Ctrl Pts',(30.1210799690045,-1.9129020287308,8.36351111415669)) ;
#58700=CARTESIAN_POINT('Ctrl Pts',(30.1208825225924,-1.91188491089433,8.36343655315723)) ;
#58701=CARTESIAN_POINT('Ctrl Pts',(30.1204920136106,-1.90986883088622,8.36328566679216)) ;
#58702=CARTESIAN_POINT('Ctrl Pts',(30.1202989409095,-1.90886987054035,8.36320937932708)) ;
#58703=CARTESIAN_POINT('Ctrl Pts',(30.1200134937087,-1.90738732919764,8.36309224022347)) ;
#58704=CARTESIAN_POINT('Ctrl Pts',(30.1199190410322,-1.90689579911753,8.363052733028)) ;
#58705=CARTESIAN_POINT('Ctrl Pts',(30.1197317685678,-1.90591842656552,8.3629722310425)) ;
#58706=CARTESIAN_POINT('Ctrl Pts',(30.1196389422281,-1.90543258344669,8.36293125935027)) ;
#58707=CARTESIAN_POINT('Ctrl Pts',(30.1194999212751,-1.90470145455269,8.3628671883431)) ;
#58708=CARTESIAN_POINT('Ctrl Pts',(30.1194504715158,-1.90444076295015,8.36284391237914)) ;
#58709=CARTESIAN_POINT('Ctrl Pts',(30.1193496683133,-1.90390716744248,8.36279478319485)) ;
#58710=CARTESIAN_POINT('Ctrl Pts',(30.1192983134635,-1.90363426334997,8.36276893489634)) ;
#58711=CARTESIAN_POINT('Ctrl Pts',(30.1191963902662,-1.9030887680236,8.36271464724955)) ;
#58712=CARTESIAN_POINT('Ctrl Pts',(30.1191458039838,-1.90281621559788,8.36268630247529)) ;
#58713=CARTESIAN_POINT('Ctrl Pts',(30.1189452598859,-1.90163369988215,8.36249513250655)) ;
#58714=CARTESIAN_POINT('Ctrl Pts',(30.1189370039164,-1.90158501825139,8.36248726244976)) ;
#58715=CARTESIAN_POINT('Ctrl Pts',(30.1189287479468,-1.90153633662063,8.36247939239298)) ;
#58716=CARTESIAN_POINT('',(33.5228460028118,-15.0366437072153,-5.51081016788309)) ;
#58717=CARTESIAN_POINT('',(33.5276414405314,-15.0366437072153,-5.48155929182947)) ;
#58718=CARTESIAN_POINT('Origin',(-1.34794834185301,-21.6462763158694,0.22098491377524)) ;
#58719=CARTESIAN_POINT('',(30.846513338502,-1.90153624401898,-5.05702918454341)) ;
#58720=CARTESIAN_POINT('Ctrl Pts',(30.8465133573145,-1.90153633646753,-5.05702918788586)) ;
#58721=CARTESIAN_POINT('Ctrl Pts',(30.8465222174296,-1.90158489349469,-5.05703716995786)) ;
#58722=CARTESIAN_POINT('Ctrl Pts',(30.8466735947567,-1.90241450269135,-5.05717354569428)) ;
#58723=CARTESIAN_POINT('Ctrl Pts',(30.8467507979956,-1.90281253748369,-5.05721107343719)) ;
#58724=CARTESIAN_POINT('Ctrl Pts',(30.8468039942045,-1.90308429852252,-5.05723373643577)) ;
#58725=CARTESIAN_POINT('Ctrl Pts',(30.8469108725669,-1.90362821098621,-5.05727659697971)) ;
#58726=CARTESIAN_POINT('Ctrl Pts',(30.8469645623025,-1.90390032361635,-5.05729669871857)) ;
#58727=CARTESIAN_POINT('Ctrl Pts',(30.8470697757015,-1.90443237212193,-5.05733456015849)) ;
#58728=CARTESIAN_POINT('Ctrl Pts',(30.8471213002402,-1.90469230818705,-5.0573523147612)) ;
#58729=CARTESIAN_POINT('Ctrl Pts',(30.8472660029257,-1.9054212966801,-5.05740087187633)) ;
#58730=CARTESIAN_POINT('Ctrl Pts',(30.8473624268972,-1.90590571009083,-5.05743149773807)) ;
#58731=CARTESIAN_POINT('Ctrl Pts',(30.8475567254483,-1.90688020657611,-5.05749114352901)) ;
#58732=CARTESIAN_POINT('Ctrl Pts',(30.8476546040474,-1.90737029029904,-5.05752013976912)) ;
#58733=CARTESIAN_POINT('Ctrl Pts',(30.8479501620357,-1.90884846925176,-5.05760553053476)) ;
#58734=CARTESIAN_POINT('Ctrl Pts',(30.8481497568644,-1.90984449025548,-5.05766036572074)) ;
#58735=CARTESIAN_POINT('Ctrl Pts',(30.8485530904156,-1.91185463829672,-5.05776788797037)) ;
#58736=CARTESIAN_POINT('Ctrl Pts',(30.8487568350939,-1.91286876350774,-5.05782053637219)) ;
#58737=CARTESIAN_POINT('Ctrl Pts',(30.8491677134176,-1.91491210053778,-5.0579244329126)) ;
#58738=CARTESIAN_POINT('Ctrl Pts',(30.8493748474824,-1.91594131239982,-5.05797567854647)) ;
#58739=CARTESIAN_POINT('Ctrl Pts',(30.8500002927029,-1.91904706548742,-5.05812789724197)) ;
#58740=CARTESIAN_POINT('Ctrl Pts',(30.8504226362961,-1.92114170896659,-5.05822739720598)) ;
#58741=CARTESIAN_POINT('Ctrl Pts',(30.8512728440463,-1.92535518708964,-5.0584236247972)) ;
#58742=CARTESIAN_POINT('Ctrl Pts',(30.8517007140664,-1.92747402218885,-5.05852031724317)) ;
#58743=CARTESIAN_POINT('Ctrl Pts',(30.8529850289116,-1.93383069872744,-5.05880631432421)) ;
#58744=CARTESIAN_POINT('Ctrl Pts',(30.8538421570137,-1.9380686583443,-5.05899160211352)) ;
#58745=CARTESIAN_POINT('Ctrl Pts',(30.8555184296128,-1.94635216115927,-5.05934807613925)) ;
#58746=CARTESIAN_POINT('Ctrl Pts',(30.8563375860309,-1.95039770503674,-5.05951919052795)) ;
#58747=CARTESIAN_POINT('Ctrl Pts',(30.8578974438038,-1.95809865321679,-5.05984161264589)) ;
#58748=CARTESIAN_POINT('Ctrl Pts',(30.8586795936983,-1.96195867181558,-5.06000146823871)) ;
#58749=CARTESIAN_POINT('Ctrl Pts',(30.8602490506149,-1.96970201797824,-5.06031949703638)) ;
#58750=CARTESIAN_POINT('Ctrl Pts',(30.8610363579311,-1.9735853455555,-5.06047766846358)) ;
#58751=CARTESIAN_POINT('Ctrl Pts',(30.8634056537684,-1.98526916037067,-5.06095042086467)) ;
#58752=CARTESIAN_POINT('Ctrl Pts',(30.864995008453,-1.99310347927764,-5.06126328654964)) ;
#58753=CARTESIAN_POINT('Ctrl Pts',(30.8681917232794,-2.00885631246943,-5.06188674003531)) ;
#58754=CARTESIAN_POINT('Ctrl Pts',(30.8697990880122,-2.01677482657967,-5.06219729960863)) ;
#58755=CARTESIAN_POINT('Ctrl Pts',(30.8730303783887,-2.03269003305421,-5.06281726598735)) ;
#58756=CARTESIAN_POINT('Ctrl Pts',(30.8746543041626,-2.04068672542293,-5.06312667200092)) ;
#58757=CARTESIAN_POINT('Ctrl Pts',(30.8795488777629,-2.06478504921205,-5.06405411240299)) ;
#58758=CARTESIAN_POINT('Ctrl Pts',(30.8828423047139,-2.08099492385557,-5.06467146935712)) ;
#58759=CARTESIAN_POINT('Ctrl Pts',(30.8894794710646,-2.11365521686435,-5.06590655965855)) ;
#58760=CARTESIAN_POINT('Ctrl Pts',(30.8928232182896,-2.13010563543453,-5.0665242455345)) ;
#58761=CARTESIAN_POINT('Ctrl Pts',(30.8995508921739,-2.16319891724182,-5.06776036095689)) ;
#58762=CARTESIAN_POINT('Ctrl Pts',(30.9029348209093,-2.17984177664019,-5.06837877293634)) ;
#58763=CARTESIAN_POINT('Ctrl Pts',(30.9097328497242,-2.21327182895652,-5.06961593039811)) ;
#58764=CARTESIAN_POINT('Ctrl Pts',(30.9131469501731,-2.23005902188247,-5.07023467363518)) ;
#58765=CARTESIAN_POINT('Ctrl Pts',(30.9234195990794,-2.28056494806296,-5.07209017971721)) ;
#58766=CARTESIAN_POINT('Ctrl Pts',(30.9303084833242,-2.31442802843042,-5.07332629036645)) ;
#58767=CARTESIAN_POINT('Ctrl Pts',(30.944088063969,-2.38215430760561,-5.07578760930222)) ;
#58768=CARTESIAN_POINT('Ctrl Pts',(30.950978764724,-2.41601749274999,-5.07701277357059)) ;
#58769=CARTESIAN_POINT('Ctrl Pts',(30.9646831779117,-2.48335912659609,-5.07944125064379)) ;
#58770=CARTESIAN_POINT('Ctrl Pts',(30.9714968932376,-2.51683757534333,-5.0806445458594)) ;
#58771=CARTESIAN_POINT('Ctrl Pts',(30.9917045603659,-2.61611857900844,-5.08420404090918)) ;
#58772=CARTESIAN_POINT('Ctrl Pts',(31.004865014558,-2.68076679099434,-5.08650996413046)) ;
#58773=CARTESIAN_POINT('Ctrl Pts',(31.0311232411281,-2.80974421165781,-5.09109666028362)) ;
#58774=CARTESIAN_POINT('Ctrl Pts',(31.0448908713434,-2.87736249833903,-5.09349292481004)) ;
#58775=CARTESIAN_POINT('Ctrl Pts',(31.0725112415595,-3.01300721611788,-5.09828766776301)) ;
#58776=CARTESIAN_POINT('Ctrl Pts',(31.08636398788,-3.081033647288,-5.10068610773375)) ;
#58777=CARTESIAN_POINT('Ctrl Pts',(31.114151471521,-3.21748148519082,-5.10548740352965)) ;
#58778=CARTESIAN_POINT('Ctrl Pts',(31.1280862113957,-3.28590289190996,-5.10789024375613)) ;
#58779=CARTESIAN_POINT('Ctrl Pts',(31.1560347071644,-3.42312751338264,-5.11270166654699)) ;
#58780=CARTESIAN_POINT('Ctrl Pts',(31.1700484633858,-3.4919307281396,-5.11511024711247)) ;
#58781=CARTESIAN_POINT('Ctrl Pts',(31.2122039196158,-3.69889333451627,-5.12234582513575)) ;
#58782=CARTESIAN_POINT('Ctrl Pts',(31.240459789465,-3.83760568758789,-5.1271827661939)) ;
#58783=CARTESIAN_POINT('Ctrl Pts',(31.2972534436847,-4.1163996286529,-5.13688609625301)) ;
#58784=CARTESIAN_POINT('Ctrl Pts',(31.3257912376979,-4.25648121672555,-5.14175242653772)) ;
#58785=CARTESIAN_POINT('Ctrl Pts',(31.383126632306,-4.53790830204276,-5.15151484518891)) ;
#58786=CARTESIAN_POINT('Ctrl Pts',(31.4119242370105,-4.67925379837917,-5.15641090732875)) ;
#58787=CARTESIAN_POINT('Ctrl Pts',(31.4697573566568,-4.96310337250663,-5.16623180664519)) ;
#58788=CARTESIAN_POINT('Ctrl Pts',(31.498792873749,-5.10560745031275,-5.17115663072387)) ;
#58789=CARTESIAN_POINT('Ctrl Pts',(31.5570800476211,-5.39166886241539,-5.18103330707449)) ;
#58790=CARTESIAN_POINT('Ctrl Pts',(31.586331705452,-5.53522619670961,-5.1859851529319)) ;
#58791=CARTESIAN_POINT('Ctrl Pts',(31.6450294699151,-5.82328879730879,-5.19591364069515)) ;
#58792=CARTESIAN_POINT('Ctrl Pts',(31.674475576737,-5.96779406361505,-5.20089028144113)) ;
#58793=CARTESIAN_POINT('Ctrl Pts',(31.7630731119485,-6.40257377433977,-5.21585357516904)) ;
#58794=CARTESIAN_POINT('Ctrl Pts',(31.8224837418014,-6.69411212587316,-5.22587367466452)) ;
#58795=CARTESIAN_POINT('Ctrl Pts',(31.9418234967792,-7.27971665165263,-5.24598021423759)) ;
#58796=CARTESIAN_POINT('Ctrl Pts',(32.0017526281241,-7.57378282593234,-5.25606661641785)) ;
#58797=CARTESIAN_POINT('Ctrl Pts',(32.1219569994905,-8.16360039960541,-5.27628094520372)) ;
#58798=CARTESIAN_POINT('Ctrl Pts',(32.1822322425905,-8.45935179899548,-5.28640885302693)) ;
#58799=CARTESIAN_POINT('Ctrl Pts',(32.3029566284287,-9.05169722610276,-5.30668029492975)) ;
#58800=CARTESIAN_POINT('Ctrl Pts',(32.36340577261,-9.34829125382689,-5.31682382021219)) ;
#58801=CARTESIAN_POINT('Ctrl Pts',(32.5447559097541,-10.2380733851616,-5.34723796026816)) ;
#58802=CARTESIAN_POINT('Ctrl Pts',(32.6656595787642,-10.8312615215168,-5.36749229368494)) ;
#58803=CARTESIAN_POINT('Ctrl Pts',(32.9060980789528,-12.0108970979659,-5.40773998693454)) ;
#58804=CARTESIAN_POINT('Ctrl Pts',(33.0256329226131,-12.5973445381112,-5.42773327069192)) ;
#58805=CARTESIAN_POINT('Ctrl Pts',(33.2619584102353,-13.7567579308779,-5.46723756451734)) ;
#58806=CARTESIAN_POINT('Ctrl Pts',(33.3787490601544,-14.3297238834965,-5.48674853824458)) ;
#58807=CARTESIAN_POINT('Ctrl Pts',(33.5032839103796,-14.9406748975524,-5.50754381324112)) ;
#58808=CARTESIAN_POINT('Ctrl Pts',(33.513072690413,-14.9886972685039,-5.50917831400048)) ;
#58809=CARTESIAN_POINT('Ctrl Pts',(33.5228460026744,-15.0366437072149,-5.51081016871875)) ;
#58810=CARTESIAN_POINT('Ctrl Pts',(33.527641440668,-15.0366437072149,-5.48155929099309)) ;
#58811=CARTESIAN_POINT('Ctrl Pts',(33.5178586766078,-14.9886972685318,-5.4799850897331)) ;
#58812=CARTESIAN_POINT('Ctrl Pts',(33.5080604095794,-14.9406748976083,-5.47840845711907)) ;
#58813=CARTESIAN_POINT('Ctrl Pts',(33.3834046007263,-14.329723883609,-5.45835099718485)) ;
#58814=CARTESIAN_POINT('Ctrl Pts',(33.266497687206,-13.7567579310195,-5.43954920008858)) ;
#58815=CARTESIAN_POINT('Ctrl Pts',(33.0299293079761,-12.5973445383116,-5.40152647960156)) ;
#58816=CARTESIAN_POINT('Ctrl Pts',(32.9102678482249,-12.0108970981961,-5.38230551986948)) ;
#58817=CARTESIAN_POINT('Ctrl Pts',(32.6695643910199,-10.8312615218069,-5.34367399299853)) ;
#58818=CARTESIAN_POINT('Ctrl Pts',(32.5485224060297,-10.2380733854818,-5.32426334977515)) ;
#58819=CARTESIAN_POINT('Ctrl Pts',(32.3669540920221,-9.3482912541922,-5.29518002976905)) ;
#58820=CARTESIAN_POINT('Ctrl Pts',(32.3064304257025,-9.0516972264831,-5.28549106944013)) ;
#58821=CARTESIAN_POINT('Ctrl Pts',(32.1855528762123,-8.45935179940588,-5.26615388452188)) ;
#58822=CARTESIAN_POINT('Ctrl Pts',(32.1251989944828,-8.16360040003082,-5.25650565113774)) ;
#58823=CARTESIAN_POINT('Ctrl Pts',(32.0048324746615,-7.57378282638767,-5.23728038420972)) ;
#58824=CARTESIAN_POINT('Ctrl Pts',(31.9448198396494,-7.2797166521229,-5.22770333188501)) ;
#58825=CARTESIAN_POINT('Ctrl Pts',(31.8253070935512,-6.69411212637314,-5.20865199150334)) ;
#58826=CARTESIAN_POINT('Ctrl Pts',(31.7658069886711,-6.40257377485455,-5.19917766554801)) ;
#58827=CARTESIAN_POINT('Ctrl Pts',(31.6770694508902,-5.9677940641519,-5.185068349742)) ;
#58828=CARTESIAN_POINT('Ctrl Pts',(31.6475757053778,-5.82328879785296,-5.18038229216232)) ;
#58829=CARTESIAN_POINT('Ctrl Pts',(31.5887804014113,-5.53522619726841,-5.17104876906804)) ;
#58830=CARTESIAN_POINT('Ctrl Pts',(31.5594788431478,-5.39166886298147,-5.16640130239347)) ;
#58831=CARTESIAN_POINT('Ctrl Pts',(31.5010891801201,-5.10560745089334,-5.15714978225379)) ;
#58832=CARTESIAN_POINT('Ctrl Pts',(31.4720010764086,-4.96310337309446,-5.15254572237146)) ;
#58833=CARTESIAN_POINT('Ctrl Pts',(31.4140595090003,-4.67925379898137,-5.14338632515737)) ;
#58834=CARTESIAN_POINT('Ctrl Pts',(31.3852060474466,-4.53790830265215,-5.13883097473451)) ;
#58835=CARTESIAN_POINT('Ctrl Pts',(31.3277548237149,-4.25648121734925,-5.12977508249897)) ;
#58836=CARTESIAN_POINT('Ctrl Pts',(31.2991570660168,-4.11639962928367,-5.12527451452018)) ;
#58837=CARTESIAN_POINT('Ctrl Pts',(31.2422380913601,-3.83760568823281,-5.11633560532754)) ;
#58838=CARTESIAN_POINT('Ctrl Pts',(31.213916884013,-3.69889333516823,-5.11189720538476)) ;
#58839=CARTESIAN_POINT('Ctrl Pts',(31.1716578011018,-3.49193072880207,-5.10529372216643)) ;
#58840=CARTESIAN_POINT('Ctrl Pts',(31.1576085571185,-3.42312751404861,-5.10310160737705)) ;
#58841=CARTESIAN_POINT('Ctrl Pts',(31.1295867818156,-3.28590289258288,-5.09873716997887)) ;
#58842=CARTESIAN_POINT('Ctrl Pts',(31.1156142508242,-3.21748148586721,-5.09656484537069)) ;
#58843=CARTESIAN_POINT('Ctrl Pts',(31.0877482927399,-3.08103364797132,-5.09224222251172)) ;
#58844=CARTESIAN_POINT('Ctrl Pts',(31.0738548682071,-3.01300721680465,-5.09009190866395)) ;
#58845=CARTESIAN_POINT('Ctrl Pts',(31.0461493680224,-2.87736249903269,-5.08581643555565)) ;
#58846=CARTESIAN_POINT('Ctrl Pts',(31.0323372986602,-2.80974421235489,-5.08369123783789)) ;
#58847=CARTESIAN_POINT('Ctrl Pts',(31.0059890678275,-2.6807667914274,-5.07965354306197)) ;
#58848=CARTESIAN_POINT('Ctrl Pts',(30.9927812368087,-2.61611857916068,-5.07763660534097)) ;
#58849=CARTESIAN_POINT('Ctrl Pts',(30.9724948246683,-2.51683757506432,-5.07455743306453)) ;
#58850=CARTESIAN_POINT('Ctrl Pts',(30.9656535716986,-2.48335912617165,-5.07352210985946)) ;
#58851=CARTESIAN_POINT('Ctrl Pts',(30.951891124577,-2.41601749203304,-5.07144762374931)) ;
#58852=CARTESIAN_POINT('Ctrl Pts',(30.9449699332981,-2.3821543067416,-5.07040844326081)) ;
#58853=CARTESIAN_POINT('Ctrl Pts',(30.9311257670399,-2.3144280272722,-5.06834107876254)) ;
#58854=CARTESIAN_POINT('Ctrl Pts',(30.9242028019896,-2.28056494675763,-5.06731285164283)) ;
#58855=CARTESIAN_POINT('Ctrl Pts',(30.913875427701,-2.23005902035775,-5.06579115534548)) ;
#58856=CARTESIAN_POINT('Ctrl Pts',(30.9104424789034,-2.21327182735896,-5.065287381856)) ;
#58857=CARTESIAN_POINT('Ctrl Pts',(30.9036052790388,-2.17984177489741,-5.06428915704125)) ;
#58858=CARTESIAN_POINT('Ctrl Pts',(30.9002010283375,-2.16319891542671,-5.06379470347773)) ;
#58859=CARTESIAN_POINT('Ctrl Pts',(30.8934308332709,-2.1301056334757,-5.06281795560951)) ;
#58860=CARTESIAN_POINT('Ctrl Pts',(30.8900648925502,-2.11365521483403,-5.06233564397707)) ;
#58861=CARTESIAN_POINT('Ctrl Pts',(30.8833807945581,-2.08099492168341,-5.06138682384278)) ;
#58862=CARTESIAN_POINT('Ctrl Pts',(30.8800626450252,-2.06478504696959,-5.06092026787666)) ;
#58863=CARTESIAN_POINT('Ctrl Pts',(30.8751281536704,-2.04068672307579,-5.06023631487228)) ;
#58864=CARTESIAN_POINT('Ctrl Pts',(30.8734904414429,-2.03269003067224,-5.06001100246102)) ;
#58865=CARTESIAN_POINT('Ctrl Pts',(30.8702303426428,-2.01677482412858,-5.059566759604)) ;
#58866=CARTESIAN_POINT('Ctrl Pts',(30.8686079562032,-2.00885630998394,-5.05934782834478)) ;
#58867=CARTESIAN_POINT('Ctrl Pts',(30.8653795095944,-1.99310347672373,-5.05891793008136)) ;
#58868=CARTESIAN_POINT('Ctrl Pts',(30.863773454092,-1.98526915778259,-5.05870693483445)) ;
#58869=CARTESIAN_POINT('Ctrl Pts',(30.8613772328026,-1.9735853429167,-5.05839842036086)) ;
#58870=CARTESIAN_POINT('Ctrl Pts',(30.8605806341427,-1.9697020153227,-5.0582969236015)) ;
#58871=CARTESIAN_POINT('Ctrl Pts',(30.8589917862301,-1.96195866912642,-5.05809717460429)) ;
#58872=CARTESIAN_POINT('Ctrl Pts',(30.858199537266,-1.95809865051073,-5.05799892058861)) ;
#58873=CARTESIAN_POINT('Ctrl Pts',(30.8566183832002,-1.95039770220822,-5.05780639995442)) ;
#58874=CARTESIAN_POINT('Ctrl Pts',(30.8557874699109,-1.94635215821993,-5.05770699916629)) ;
#58875=CARTESIAN_POINT('Ctrl Pts',(30.8540851221175,-1.93806865517772,-5.05750957649875)) ;
#58876=CARTESIAN_POINT('Ctrl Pts',(30.8532136992519,-1.93383069544475,-5.0574114827615)) ;
#58877=CARTESIAN_POINT('Ctrl Pts',(30.8519052948742,-1.92747401873175,-5.05727242510519)) ;
#58878=CARTESIAN_POINT('Ctrl Pts',(30.8514689484325,-1.92535518357459,-5.05722743646948)) ;
#58879=CARTESIAN_POINT('Ctrl Pts',(30.8506005905671,-1.92114170533599,-5.05714191953601)) ;
#58880=CARTESIAN_POINT('Ctrl Pts',(30.8501685848271,-1.9190470617987,-5.05710135598556)) ;
#58881=CARTESIAN_POINT('Ctrl Pts',(30.8495272760002,-1.91594130862596,-5.05704590089974)) ;
#58882=CARTESIAN_POINT('Ctrl Pts',(30.8493146219259,-1.91491209673629,-5.0570283257986)) ;
#58883=CARTESIAN_POINT('Ctrl Pts',(30.8488920774437,-1.91286875965011,-5.05699558960563)) ;
#58884=CARTESIAN_POINT('Ctrl Pts',(30.8486821874486,-1.9118546344095,-5.05698042594019)) ;
#58885=CARTESIAN_POINT('Ctrl Pts',(30.8482656350974,-1.90984448631342,-5.05695353473325)) ;
#58886=CARTESIAN_POINT('Ctrl Pts',(30.8480589794452,-1.90884846528467,-5.05694176863321)) ;
#58887=CARTESIAN_POINT('Ctrl Pts',(30.8477516275676,-1.90737028629171,-5.05692831735834)) ;
#58888=CARTESIAN_POINT('Ctrl Pts',(30.8476496140468,-1.90688020255704,-5.05692454300991)) ;
#58889=CARTESIAN_POINT('Ctrl Pts',(30.8474464414083,-1.90590570604561,-5.05691902672418)) ;
#58890=CARTESIAN_POINT('Ctrl Pts',(30.8473452860647,-1.90542129261717,-5.05691726093279)) ;
#58891=CARTESIAN_POINT('Ctrl Pts',(30.8471926538241,-1.90469230450297,-5.05691707244812)) ;
#58892=CARTESIAN_POINT('Ctrl Pts',(30.8471381574318,-1.9044323688528,-5.05691744588009)) ;
#58893=CARTESIAN_POINT('Ctrl Pts',(30.8470263625795,-1.90390032118951,-5.05691973060544)) ;
#58894=CARTESIAN_POINT('Ctrl Pts',(30.8469690648644,-1.90362820899944,-5.05692163712989)) ;
#58895=CARTESIAN_POINT('Ctrl Pts',(30.8468540959934,-1.90308429739362,-5.05692812760186)) ;
#58896=CARTESIAN_POINT('Ctrl Pts',(30.8467964482283,-1.90281253677263,-5.05693261842809)) ;
#58897=CARTESIAN_POINT('Ctrl Pts',(30.8465349543911,-1.90163369810809,-5.05702182057777)) ;
#58898=CARTESIAN_POINT('Ctrl Pts',(30.8465241558528,-1.90158501728781,-5.05702550423181)) ;
#58899=CARTESIAN_POINT('Ctrl Pts',(30.8465133573145,-1.90153633646753,-5.05702918788586)) ;
#58900=CARTESIAN_POINT('',(28.1105818993065,-15.0366437072153,-19.0773535407052)) ;
#58901=CARTESIAN_POINT('',(28.12721624477,-15.0366437072153,-19.0528197166357)) ;
#58902=CARTESIAN_POINT('Origin',(-1.13057562514854,-21.6462763158694,0.766549294070821)) ;
#58903=CARTESIAN_POINT('',(25.8721458475363,-1.90153624261815,-17.5417501561681)) ;
#58904=CARTESIAN_POINT('Ctrl Pts',(25.8721458629685,-1.90153633366587,-17.541750166936)) ;
#58905=CARTESIAN_POINT('Ctrl Pts',(25.8721505680015,-1.90158489404723,-17.541761110063)) ;
#58906=CARTESIAN_POINT('Ctrl Pts',(25.872231662671,-1.90242186758655,-17.5419497228258)) ;
#58907=CARTESIAN_POINT('Ctrl Pts',(25.8722864941205,-1.90282329671317,-17.5420166801772)) ;
#58908=CARTESIAN_POINT('Ctrl Pts',(25.8723256207478,-1.90309737338209,-17.5420599024175)) ;
#58909=CARTESIAN_POINT('Ctrl Pts',(25.87240535646,-1.90364591739461,-17.542144304304)) ;
#58910=CARTESIAN_POINT('Ctrl Pts',(25.8724460128044,-1.90392034589288,-17.5421853999427)) ;
#58911=CARTESIAN_POINT('Ctrl Pts',(25.8725263299213,-1.90445692101583,-17.5422645367358)) ;
#58912=CARTESIAN_POINT('Ctrl Pts',(25.8725659935202,-1.90471906782239,-17.5423025737883)) ;
#58913=CARTESIAN_POINT('Ctrl Pts',(25.8726779452118,-1.90545432006084,-17.5424082166215)) ;
#58914=CARTESIAN_POINT('Ctrl Pts',(25.8727532776597,-1.90594291769499,-17.5424770373722)) ;
#58915=CARTESIAN_POINT('Ctrl Pts',(25.8729059462109,-1.90692583135594,-17.542613829521)) ;
#58916=CARTESIAN_POINT('Ctrl Pts',(25.8729832960174,-1.90742014803357,-17.5426817809481)) ;
#58917=CARTESIAN_POINT('Ctrl Pts',(25.8732177773336,-1.90891109407639,-17.5428849930091)) ;
#58918=CARTESIAN_POINT('Ctrl Pts',(25.8733773182412,-1.909915717438,-17.5430196438642)) ;
#58919=CARTESIAN_POINT('Ctrl Pts',(25.8737010965169,-1.91194322613707,-17.5432887438504)) ;
#58920=CARTESIAN_POINT('Ctrl Pts',(25.873865355643,-1.91296610964748,-17.543423160218)) ;
#58921=CARTESIAN_POINT('Ctrl Pts',(25.8741975644926,-1.91502709322433,-17.5436921532795)) ;
#58922=CARTESIAN_POINT('Ctrl Pts',(25.8743655156668,-1.91606519333414,-17.5438267278498)) ;
#58923=CARTESIAN_POINT('Ctrl Pts',(25.8748737080304,-1.91919776711167,-17.5442307815105)) ;
#58924=CARTESIAN_POINT('Ctrl Pts',(25.8752182593229,-1.92131049897224,-17.5445006273183)) ;
#58925=CARTESIAN_POINT('Ctrl Pts',(25.8759135806846,-1.92556036178824,-17.545040131977)) ;
#58926=CARTESIAN_POINT('Ctrl Pts',(25.8762643709515,-1.92769749319939,-17.5453097612064)) ;
#58927=CARTESIAN_POINT('Ctrl Pts',(25.877319104743,-1.93410905870646,-17.5461152268159)) ;
#58928=CARTESIAN_POINT('Ctrl Pts',(25.8780253649344,-1.93838361099844,-17.5466476898942)) ;
#58929=CARTESIAN_POINT('Ctrl Pts',(25.8794090677594,-1.9467386359022,-17.5476836482434)) ;
#58930=CARTESIAN_POINT('Ctrl Pts',(25.8800865515514,-1.95081910919327,-17.5481870830604)) ;
#58931=CARTESIAN_POINT('Ctrl Pts',(25.8813781226031,-1.95858685031422,-17.5491426562885)) ;
#58932=CARTESIAN_POINT('Ctrl Pts',(25.8820265367721,-1.96248050050301,-17.5496201673265)) ;
#58933=CARTESIAN_POINT('Ctrl Pts',(25.8833287929376,-1.97029131284115,-17.5505758423184)) ;
#58934=CARTESIAN_POINT('Ctrl Pts',(25.8839826359515,-1.97420847500389,-17.5510540047764)) ;
#58935=CARTESIAN_POINT('Ctrl Pts',(25.8859516548851,-1.98599408824657,-17.5524900126839)) ;
#58936=CARTESIAN_POINT('Ctrl Pts',(25.887274293954,-1.99389666566597,-17.5534494179564)) ;
#58937=CARTESIAN_POINT('Ctrl Pts',(25.8899370080667,-2.00978674928339,-17.5553737876842)) ;
#58938=CARTESIAN_POINT('Ctrl Pts',(25.8912770992061,-2.01777425530681,-17.5563387283357)) ;
#58939=CARTESIAN_POINT('Ctrl Pts',(25.8939729216926,-2.03382812662241,-17.5582745822623)) ;
#58940=CARTESIAN_POINT('Ctrl Pts',(25.8953286535016,-2.04189449191906,-17.5592454948569)) ;
#58941=CARTESIAN_POINT('Ctrl Pts',(25.8994170370107,-2.06620277743539,-17.5621671920232)) ;
#58942=CARTESIAN_POINT('Ctrl Pts',(25.9021708189187,-2.08255388382099,-17.5641270200586)) ;
#58943=CARTESIAN_POINT('Ctrl Pts',(25.9077242644949,-2.11549873574347,-17.5680683583183)) ;
#58944=CARTESIAN_POINT('Ctrl Pts',(25.9105239553166,-2.13209248148531,-17.5700498285693)) ;
#58945=CARTESIAN_POINT('Ctrl Pts',(25.9161597913601,-2.16547409398065,-17.5740304885995)) ;
#58946=CARTESIAN_POINT('Ctrl Pts',(25.9189959458912,-2.18226195689482,-17.5760296632346)) ;
#58947=CARTESIAN_POINT('Ctrl Pts',(25.9246957238415,-2.21598327350102,-17.5800411132428)) ;
#58948=CARTESIAN_POINT('Ctrl Pts',(25.9275593485239,-2.23291672720091,-17.5820533867552)) ;
#58949=CARTESIAN_POINT('Ctrl Pts',(25.9361782978858,-2.28386269296286,-17.5881024187311)) ;
#58950=CARTESIAN_POINT('Ctrl Pts',(25.9419616569795,-2.3180208093972,-17.5921514488495)) ;
#58951=CARTESIAN_POINT('Ctrl Pts',(25.9535346243998,-2.38633716071619,-17.6002403357774)) ;
#58952=CARTESIAN_POINT('Ctrl Pts',(25.959324255279,-2.42049538193591,-17.6042801542918)) ;
#58953=CARTESIAN_POINT('Ctrl Pts',(25.9708422681443,-2.488423735256,-17.6123072114952)) ;
#58954=CARTESIAN_POINT('Ctrl Pts',(25.9765706601812,-2.52219386740186,-17.616294435377)) ;
#58955=CARTESIAN_POINT('Ctrl Pts',(25.9935634036828,-2.62233986322234,-17.6281111292612)) ;
#58956=CARTESIAN_POINT('Ctrl Pts',(26.0046352573757,-2.68755132592453,-17.6357957174787)) ;
#58957=CARTESIAN_POINT('Ctrl Pts',(26.0267419583726,-2.81770994402766,-17.6511221421599)) ;
#58958=CARTESIAN_POINT('Ctrl Pts',(26.0383411847504,-2.88597501380354,-17.6591534154139)) ;
#58959=CARTESIAN_POINT('Ctrl Pts',(26.0616166564067,-3.02291720165828,-17.6752541057803)) ;
#58960=CARTESIAN_POINT('Ctrl Pts',(26.0732929237367,-3.09159431980986,-17.6833234903958)) ;
#58961=CARTESIAN_POINT('Ctrl Pts',(26.0967186911401,-3.22934730962459,-17.6995010917953)) ;
#58962=CARTESIAN_POINT('Ctrl Pts',(26.1084682001473,-3.29842318127411,-17.7076092953976)) ;
#58963=CARTESIAN_POINT('Ctrl Pts',(26.1320371662318,-3.43696038462189,-17.7238644839388)) ;
#58964=CARTESIAN_POINT('Ctrl Pts',(26.1438566244585,-3.50642171632358,-17.7320114671818)) ;
#58965=CARTESIAN_POINT('Ctrl Pts',(26.1794154334704,-3.71536396265693,-17.7565098653357)) ;
#58966=CARTESIAN_POINT('Ctrl Pts',(26.2032551570819,-3.85540312786147,-17.7729188191408)) ;
#58967=CARTESIAN_POINT('Ctrl Pts',(26.2511803855432,-4.13686379005994,-17.8058832750933)) ;
#58968=CARTESIAN_POINT('Ctrl Pts',(26.2752659240111,-4.27828528713331,-17.8224387276865)) ;
#58969=CARTESIAN_POINT('Ctrl Pts',(26.3236624029499,-4.56240427986944,-17.8556870807628)) ;
#58970=CARTESIAN_POINT('Ctrl Pts',(26.3479733582527,-4.7051017746222,-17.8723799590352)) ;
#58971=CARTESIAN_POINT('Ctrl Pts',(26.3968010309501,-4.99166642754464,-17.9058929718701)) ;
#58972=CARTESIAN_POINT('Ctrl Pts',(26.4213177558355,-5.13553358572935,-17.9227130953899)) ;
#58973=CARTESIAN_POINT('Ctrl Pts',(26.4705377650822,-5.42433123310099,-17.9564697631733)) ;
#58974=CARTESIAN_POINT('Ctrl Pts',(26.4952410531139,-5.56926172228562,-17.9734063020221)) ;
#58975=CARTESIAN_POINT('Ctrl Pts',(26.5448152636506,-5.8600796997275,-18.0073845556476)) ;
#58976=CARTESIAN_POINT('Ctrl Pts',(26.569686186818,-6.00596718798611,-18.0244262694466)) ;
#58977=CARTESIAN_POINT('Ctrl Pts',(26.6445222918619,-6.44490565398653,-18.0756919075071)) ;
#58978=CARTESIAN_POINT('Ctrl Pts',(26.6947107654887,-6.73923262825523,-18.1100563912884)) ;
#58979=CARTESIAN_POINT('Ctrl Pts',(26.7955346120393,-7.3304385783359,-18.1790660152525)) ;
#58980=CARTESIAN_POINT('Ctrl Pts',(26.8461700066388,-7.62731755418156,-18.2137111234783)) ;
#58981=CARTESIAN_POINT('Ctrl Pts',(26.9477402734718,-8.22277685021324,-18.283186169508)) ;
#58982=CARTESIAN_POINT('Ctrl Pts',(26.9986751564425,-8.52135717039598,-18.3180160914743)) ;
#58983=CARTESIAN_POINT('Ctrl Pts',(27.1006975970256,-9.11936849871233,-18.3877640259897)) ;
#58984=CARTESIAN_POINT('Ctrl Pts',(27.1517851596633,-9.41879950685285,-18.4226820311287)) ;
#58985=CARTESIAN_POINT('Ctrl Pts',(27.3050572428128,-10.3170925794686,-18.5274222073615)) ;
#58986=CARTESIAN_POINT('Ctrl Pts',(27.4072510673143,-10.9159546767068,-18.5972306681566)) ;
#58987=CARTESIAN_POINT('Ctrl Pts',(27.6104950296067,-12.1068736981433,-18.7360283725215)) ;
#58988=CARTESIAN_POINT('Ctrl Pts',(27.7115452108907,-12.6989306223933,-18.8050175519609)) ;
#58989=CARTESIAN_POINT('Ctrl Pts',(27.9125385133627,-13.8764819135214,-18.9422120174696)) ;
#58990=CARTESIAN_POINT('Ctrl Pts',(28.0124536696358,-14.4618113899862,-19.0103978272271)) ;
#58991=CARTESIAN_POINT('Ctrl Pts',(28.1105818992948,-15.0366437072153,-19.0773535407226)) ;
#58992=CARTESIAN_POINT('Ctrl Pts',(28.1272162447826,-15.0366437072153,-19.0528197166172)) ;
#58993=CARTESIAN_POINT('Ctrl Pts',(28.1260439213675,-15.0298036697796,-19.0520298964312)) ;
#58994=CARTESIAN_POINT('Ctrl Pts',(28.124871342501,-15.0229621460442,-19.0512399056728)) ;
#58995=CARTESIAN_POINT('Ctrl Pts',(28.0263071912092,-14.4478805128969,-18.9848353170201)) ;
#58996=CARTESIAN_POINT('Ctrl Pts',(27.9271614144017,-13.869434029792,-18.9180494439821)) ;
#58997=CARTESIAN_POINT('Ctrl Pts',(27.7265237475049,-12.6989306224415,-18.7829258632544)) ;
#58998=CARTESIAN_POINT('Ctrl Pts',(27.6250318781892,-12.1068736981987,-18.7145881249272)) ;
#58999=CARTESIAN_POINT('Ctrl Pts',(27.4208636967858,-10.9159546767766,-18.5771535417749)) ;
#59000=CARTESIAN_POINT('Ctrl Pts',(27.3181874281729,-10.3170925795457,-18.5080566328121)) ;
#59001=CARTESIAN_POINT('Ctrl Pts',(27.1641543967029,-9.41879950694078,-18.4044387713905)) ;
#59002=CARTESIAN_POINT('Ctrl Pts',(27.1128069266329,-9.11936849880387,-18.3699041010365)) ;
#59003=CARTESIAN_POINT('Ctrl Pts',(27.0102503212534,-8.52135717049476,-18.300944000657)) ;
#59004=CARTESIAN_POINT('Ctrl Pts',(26.9590411909696,-8.2227768503156,-18.2665185632173)) ;
#59005=CARTESIAN_POINT('Ctrl Pts',(26.8569054593982,-7.62731755429113,-18.1978775152843)) ;
#59006=CARTESIAN_POINT('Ctrl Pts',(26.805978868849,-7.33043857844908,-18.1636618889539)) ;
#59007=CARTESIAN_POINT('Ctrl Pts',(26.7045517821677,-6.73923262837554,-18.0955419776217)) ;
#59008=CARTESIAN_POINT('Ctrl Pts',(26.6540513076982,-6.4449056541104,-18.0616376606576)) ;
#59009=CARTESIAN_POINT('Ctrl Pts',(26.5787270255406,-6.00596718811531,-18.0110920299747)) ;
#59010=CARTESIAN_POINT('Ctrl Pts',(26.5536899925335,-5.86007969985845,-17.9942953098607)) ;
#59011=CARTESIAN_POINT('Ctrl Pts',(26.5037756790954,-5.56926172242007,-17.9608186704879)) ;
#59012=CARTESIAN_POINT('Ctrl Pts',(26.4788983993272,-5.42433123323721,-17.9441387502522)) ;
#59013=CARTESIAN_POINT('Ctrl Pts',(26.4293210373901,-5.13553358586907,-17.9109091382572)) ;
#59014=CARTESIAN_POINT('Ctrl Pts',(26.4046209588946,-4.9916664276861,-17.894359441081)) ;
#59015=CARTESIAN_POINT('Ctrl Pts',(26.3554151654589,-4.70510177476713,-17.8614041146133)) ;
#59016=CARTESIAN_POINT('Ctrl Pts',(26.3309094580062,-4.56240428001608,-17.8449984742729)) ;
#59017=CARTESIAN_POINT('Ctrl Pts',(26.2821091285874,-4.27828528728337,-17.8123457560937)) ;
#59018=CARTESIAN_POINT('Ctrl Pts',(26.2578145217622,-4.13686379021172,-17.7960986562588)) ;
#59019=CARTESIAN_POINT('Ctrl Pts',(26.2094523539447,-3.85540312801667,-17.7637786376448)) ;
#59020=CARTESIAN_POINT('Ctrl Pts',(26.1853848265438,-3.71536396281382,-17.7477056692929)) ;
#59021=CARTESIAN_POINT('Ctrl Pts',(26.1494647130129,-3.50642171648299,-17.723740155438)) ;
#59022=CARTESIAN_POINT('Ctrl Pts',(26.1375215227776,-3.43696038478214,-17.7157756632548)) ;
#59023=CARTESIAN_POINT('Ctrl Pts',(26.1136970574172,-3.29842318143604,-17.6998973079537)) ;
#59024=CARTESIAN_POINT('Ctrl Pts',(26.1018157834405,-3.22934730978736,-17.6919834431423)) ;
#59025=CARTESIAN_POINT('Ctrl Pts',(26.0781163980241,-3.0915943199743,-17.6762093981207)) ;
#59026=CARTESIAN_POINT('Ctrl Pts',(26.0662982955211,-3.02291720182354,-17.668349204735)) ;
#59027=CARTESIAN_POINT('Ctrl Pts',(26.0427259888543,-2.88597501397047,-17.652686313256)) ;
#59028=CARTESIAN_POINT('Ctrl Pts',(26.0309718067178,-2.81770994419542,-17.6448835826481)) ;
#59029=CARTESIAN_POINT('Ctrl Pts',(26.0085513814615,-2.68755132608213,-17.6300198666284)) ;
#59030=CARTESIAN_POINT('Ctrl Pts',(25.9973144624006,-2.62233986336839,-17.6225787316105)) ;
#59031=CARTESIAN_POINT('Ctrl Pts',(25.9800473661399,-2.52219386753023,-17.6111666777666)) ;
#59032=CARTESIAN_POINT('Ctrl Pts',(25.974223031518,-2.48842373537836,-17.6073209586087)) ;
#59033=CARTESIAN_POINT('Ctrl Pts',(25.96250282621,-2.42049538204628,-17.5995921129432)) ;
#59034=CARTESIAN_POINT('Ctrl Pts',(25.9566069655597,-2.38633716082053,-17.5957089716173)) ;
#59035=CARTESIAN_POINT('Ctrl Pts',(25.9448089810994,-2.31802080948946,-17.5879519599898)) ;
#59036=CARTESIAN_POINT('Ctrl Pts',(25.9389068845097,-2.28386269304911,-17.5840780545739)) ;
#59037=CARTESIAN_POINT('Ctrl Pts',(25.9300972726076,-2.23291672727815,-17.5783102288032)) ;
#59038=CARTESIAN_POINT('Ctrl Pts',(25.9271679806095,-2.21598327357521,-17.5763948073344)) ;
#59039=CARTESIAN_POINT('Ctrl Pts',(25.9213317316417,-2.18226195696306,-17.572584637016)) ;
#59040=CARTESIAN_POINT('Ctrl Pts',(25.9184247759445,-2.16547409404589,-17.5706898862874)) ;
#59041=CARTESIAN_POINT('Ctrl Pts',(25.912640797489,-2.13209248154464,-17.5669277199662)) ;
#59042=CARTESIAN_POINT('Ctrl Pts',(25.909763785347,-2.11549873579995,-17.5650602901298)) ;
#59043=CARTESIAN_POINT('Ctrl Pts',(25.9040468317566,-2.08255388387165,-17.5613601081469)) ;
#59044=CARTESIAN_POINT('Ctrl Pts',(25.9012069173771,-2.06620277748319,-17.5595273160017)) ;
#59045=CARTESIAN_POINT('Ctrl Pts',(25.896979461996,-2.04189449196258,-17.5568107344993)) ;
#59046=CARTESIAN_POINT('Ctrl Pts',(25.8955756987359,-2.03382812666439,-17.5559106629946)) ;
#59047=CARTESIAN_POINT('Ctrl Pts',(25.8927795087419,-2.01777425534598,-17.5541228400657)) ;
#59048=CARTESIAN_POINT('Ctrl Pts',(25.8913870824749,-2.00978674932117,-17.5532350879521)) ;
#59049=CARTESIAN_POINT('Ctrl Pts',(25.8886138157077,-1.99389666570093,-17.55147377119)) ;
#59050=CARTESIAN_POINT('Ctrl Pts',(25.8872329913601,-1.98599408828015,-17.5506001827826)) ;
#59051=CARTESIAN_POINT('Ctrl Pts',(25.8851701644093,-1.97420847503537,-17.5493025313486)) ;
#59052=CARTESIAN_POINT('Ctrl Pts',(25.8844839503814,-1.9702913128718,-17.548872112564)) ;
#59053=CARTESIAN_POINT('Ctrl Pts',(25.8831141358671,-1.96248050053228,-17.5480160786815)) ;
#59054=CARTESIAN_POINT('Ctrl Pts',(25.8824305363957,-1.95858685034292,-17.5475904620819)) ;
#59055=CARTESIAN_POINT('Ctrl Pts',(25.8810647713827,-1.95081910920302,-17.5467443167528)) ;
#59056=CARTESIAN_POINT('Ctrl Pts',(25.8803463295568,-1.94673863589274,-17.5463012905094)) ;
#59057=CARTESIAN_POINT('Ctrl Pts',(25.8788717871484,-1.93838361094976,-17.5453993105077)) ;
#59058=CARTESIAN_POINT('Ctrl Pts',(25.8781157274861,-1.93410905863785,-17.5449402961466)) ;
#59059=CARTESIAN_POINT('Ctrl Pts',(25.8769770714627,-1.92769749310063,-17.5442586065577)) ;
#59060=CARTESIAN_POINT('Ctrl Pts',(25.8765967513452,-1.92556036167893,-17.5440325305957)) ;
#59061=CARTESIAN_POINT('Ctrl Pts',(25.8758381991075,-1.92131049884297,-17.5435862844946)) ;
#59062=CARTESIAN_POINT('Ctrl Pts',(25.8754599870247,-1.91919776697313,-17.5433660846349)) ;
#59063=CARTESIAN_POINT('Ctrl Pts',(25.8748965291957,-1.91606519318084,-17.543043541432)) ;
#59064=CARTESIAN_POINT('Ctrl Pts',(25.8747093474316,-1.91502709306561,-17.5429373298579)) ;
#59065=CARTESIAN_POINT('Ctrl Pts',(25.8743364959667,-1.9129661094791,-17.5427282801657)) ;
#59066=CARTESIAN_POINT('Ctrl Pts',(25.8741508277133,-1.9119432259641,-17.5426254398969)) ;
#59067=CARTESIAN_POINT('Ctrl Pts',(25.8737809973961,-1.90991571725549,-17.5424242615868)) ;
#59068=CARTESIAN_POINT('Ctrl Pts',(25.8735968577151,-1.9089110938889,-17.5423258912064)) ;
#59069=CARTESIAN_POINT('Ctrl Pts',(25.8733212879543,-1.90742014783921,-17.5421832800649)) ;
#59070=CARTESIAN_POINT('Ctrl Pts',(25.873229532523,-1.90692583116035,-17.5421365753442)) ;
#59071=CARTESIAN_POINT('Ctrl Pts',(25.8730459473443,-1.90594291749478,-17.5420453818077)) ;
#59072=CARTESIAN_POINT('Ctrl Pts',(25.8729541310736,-1.90545431985745,-17.5420008728757)) ;
#59073=CARTESIAN_POINT('Ctrl Pts',(25.8728145537844,-1.90471906780893,-17.5419359748206)) ;
#59074=CARTESIAN_POINT('Ctrl Pts',(25.8727645372593,-1.90445692120481,-17.5419132072665)) ;
#59075=CARTESIAN_POINT('Ctrl Pts',(25.872661292673,-1.90392034649367,-17.5418678861124)) ;
#59076=CARTESIAN_POINT('Ctrl Pts',(25.8726080673986,-1.90364591820329,-17.5418453283351)) ;
#59077=CARTESIAN_POINT('Ctrl Pts',(25.8725001468687,-1.90309737461164,-17.5418024960997)) ;
#59078=CARTESIAN_POINT('Ctrl Pts',(25.8724455122429,-1.90282329814739,-17.5417821465215)) ;
#59079=CARTESIAN_POINT('Ctrl Pts',(25.8721685331813,-1.90163370002429,-17.5417525863779)) ;
#59080=CARTESIAN_POINT('Ctrl Pts',(25.8721571980749,-1.90158501684508,-17.541751376657)) ;
#59081=CARTESIAN_POINT('Ctrl Pts',(25.8721458629685,-1.90153633366587,-17.541750166936)) ;
#59082=CARTESIAN_POINT('',(17.5021003261044,-15.0366437072153,-29.1174641239524)) ;
#59083=CARTESIAN_POINT('',(17.5274987345145,-15.0366437072153,-29.1021824086489)) ;
#59084=CARTESIAN_POINT('Origin',(-0.704216953074884,-21.6462763158693,1.17041768075435)) ;
#59085=CARTESIAN_POINT('',(16.1153339123929,-1.90153624029605,-26.7838933346086)) ;
#59086=CARTESIAN_POINT('Ctrl Pts',(16.1153339216337,-1.90153632902166,-26.7838933504477)) ;
#59087=CARTESIAN_POINT('Ctrl Pts',(16.1153335953233,-1.9015848891725,-26.7839052586496)) ;
#59088=CARTESIAN_POINT('Ctrl Pts',(16.1153279744952,-1.90242135746351,-26.784110382256)) ;
#59089=CARTESIAN_POINT('Ctrl Pts',(16.1153496048023,-1.90282255227177,-26.7841941289722)) ;
#59090=CARTESIAN_POINT('Ctrl Pts',(16.1153669531215,-1.90309646909155,-26.7842497548283)) ;
#59091=CARTESIAN_POINT('Ctrl Pts',(16.1154038521165,-1.903644693376,-26.7843597756432)) ;
#59092=CARTESIAN_POINT('Ctrl Pts',(16.1154234811304,-1.90391896201011,-26.7844141141024)) ;
#59093=CARTESIAN_POINT('Ctrl Pts',(16.1154631181323,-1.90445522464972,-26.7845196025717)) ;
#59094=CARTESIAN_POINT('Ctrl Pts',(16.1154831305781,-1.90471721884436,-26.7845707499452)) ;
#59095=CARTESIAN_POINT('Ctrl Pts',(16.115540337139,-1.90545203888158,-26.7847135557674)) ;
#59096=CARTESIAN_POINT('Ctrl Pts',(16.1155797829326,-1.90594034787055,-26.7848075936928)) ;
#59097=CARTESIAN_POINT('Ctrl Pts',(16.1156608488187,-1.90692268088041,-26.7849957396781)) ;
#59098=CARTESIAN_POINT('Ctrl Pts',(16.1157024897167,-1.90741670555177,-26.7850898353766)) ;
#59099=CARTESIAN_POINT('Ctrl Pts',(16.1158298881831,-1.9089067708687,-26.7853725602131)) ;
#59100=CARTESIAN_POINT('Ctrl Pts',(16.1159180875171,-1.90991080080438,-26.785561647068)) ;
#59101=CARTESIAN_POINT('Ctrl Pts',(16.1160988314327,-1.91193711189471,-26.7859416082069)) ;
#59102=CARTESIAN_POINT('Ctrl Pts',(16.1161914094641,-1.91295939122146,-26.7861324619241)) ;
#59103=CARTESIAN_POINT('Ctrl Pts',(16.1163798463095,-1.91501915746764,-26.786515863185)) ;
#59104=CARTESIAN_POINT('Ctrl Pts',(16.1164757072989,-1.91605664442983,-26.7867084094301)) ;
#59105=CARTESIAN_POINT('Ctrl Pts',(16.1167670878519,-1.91918736800688,-26.7872881678793)) ;
#59106=CARTESIAN_POINT('Ctrl Pts',(16.1169663635439,-1.92129885205805,-26.7876775210615)) ;
#59107=CARTESIAN_POINT('Ctrl Pts',(16.1173706348745,-1.92554620490979,-26.7884586670275)) ;
#59108=CARTESIAN_POINT('Ctrl Pts',(16.1175756613148,-1.92768207416669,-26.7888504413886)) ;
#59109=CARTESIAN_POINT('Ctrl Pts',(16.1181943210993,-1.93408985320923,-26.7900236514862)) ;
#59110=CARTESIAN_POINT('Ctrl Pts',(16.1186114723357,-1.93836188118933,-26.7908029990837)) ;
#59111=CARTESIAN_POINT('Ctrl Pts',(16.1194317942334,-1.94671197220809,-26.7923233251266)) ;
#59112=CARTESIAN_POINT('Ctrl Pts',(16.1198350276133,-1.95079003592607,-26.7930642659994)) ;
#59113=CARTESIAN_POINT('Ctrl Pts',(16.1206055169498,-1.95855316926191,-26.794473011271)) ;
#59114=CARTESIAN_POINT('Ctrl Pts',(16.1209932609039,-1.96244449927012,-26.795178234885)) ;
#59115=CARTESIAN_POINT('Ctrl Pts',(16.1217733986971,-1.97025065724297,-26.7965915516703)) ;
#59116=CARTESIAN_POINT('Ctrl Pts',(16.1221657940786,-1.97416548522092,-26.7972996439166)) ;
#59117=CARTESIAN_POINT('Ctrl Pts',(16.1233491364704,-1.98594407558046,-26.7994284424439)) ;
#59118=CARTESIAN_POINT('Ctrl Pts',(16.1241461989878,-1.99384194397278,-26.8008536949254)) ;
#59119=CARTESIAN_POINT('Ctrl Pts',(16.1257538074971,-2.00972255893998,-26.8037165582988)) ;
#59120=CARTESIAN_POINT('Ctrl Pts',(16.1265643780836,-2.01770530534027,-26.8051541543504)) ;
#59121=CARTESIAN_POINT('Ctrl Pts',(16.1281972001052,-2.03374961042777,-26.8080413264793)) ;
#59122=CARTESIAN_POINT('Ctrl Pts',(16.1290194522432,-2.04181116911945,-26.8094909021344)) ;
#59123=CARTESIAN_POINT('Ctrl Pts',(16.1315016683943,-2.06610496976883,-26.8138566462427)) ;
#59124=CARTESIAN_POINT('Ctrl Pts',(16.1331770043602,-2.08244633284062,-26.8167898838212)) ;
#59125=CARTESIAN_POINT('Ctrl Pts',(16.1365601959366,-2.11537155357574,-26.8226952780538)) ;
#59126=CARTESIAN_POINT('Ctrl Pts',(16.1382680929498,-2.13195541144395,-26.8256674098459)) ;
#59127=CARTESIAN_POINT('Ctrl Pts',(16.1417095180794,-2.16531713254428,-26.8316430424412)) ;
#59128=CARTESIAN_POINT('Ctrl Pts',(16.1434430610002,-2.18209499193708,-26.8346465334107)) ;
#59129=CARTESIAN_POINT('Ctrl Pts',(16.1469295656395,-2.21579621476455,-26.8406769245025)) ;
#59130=CARTESIAN_POINT('Ctrl Pts',(16.1486825293011,-2.23271957820714,-26.843703823457)) ;
#59131=CARTESIAN_POINT('Ctrl Pts',(16.1539617626142,-2.2836351864612,-26.852807377152)) ;
#59132=CARTESIAN_POINT('Ctrl Pts',(16.1575083122125,-2.31777294890895,-26.8589069261871)) ;
#59133=CARTESIAN_POINT('Ctrl Pts',(16.1646109320275,-2.38604859225412,-26.8711003244594)) ;
#59134=CARTESIAN_POINT('Ctrl Pts',(16.1681670387747,-2.42018645948669,-26.877194148421)) ;
#59135=CARTESIAN_POINT('Ctrl Pts',(16.1752457642938,-2.48807433612738,-26.8893084008)) ;
#59136=CARTESIAN_POINT('Ctrl Pts',(16.1787683984017,-2.52182434558099,-26.8953288200009)) ;
#59137=CARTESIAN_POINT('Ctrl Pts',(16.1892225990797,-2.62191066721012,-26.9131778237026)) ;
#59138=CARTESIAN_POINT('Ctrl Pts',(16.1960403645944,-2.68708327229862,-26.9247942140295)) ;
#59139=CARTESIAN_POINT('Ctrl Pts',(16.2096598584406,-2.81716036725213,-26.9479719791873)) ;
#59140=CARTESIAN_POINT('Ctrl Pts',(16.2168100717623,-2.88538078201676,-26.9601234212194)) ;
#59141=CARTESIAN_POINT('Ctrl Pts',(16.2311643500484,-3.02223339031803,-26.9844932177342)) ;
#59142=CARTESIAN_POINT('Ctrl Pts',(16.238368448649,-3.09086558392735,-26.9967115519961)) ;
#59143=CARTESIAN_POINT('Ctrl Pts',(16.2528267741834,-3.2285284638215,-27.0212141688352)) ;
#59144=CARTESIAN_POINT('Ctrl Pts',(16.2600810147522,-3.2975591500927,-27.0334984432048)) ;
#59145=CARTESIAN_POINT('Ctrl Pts',(16.2746366660444,-3.43600573054254,-27.0581315160813)) ;
#59146=CARTESIAN_POINT('Ctrl Pts',(16.2819380785228,-3.50542162472458,-27.0704803135319)) ;
#59147=CARTESIAN_POINT('Ctrl Pts',(16.3039093040814,-3.71422719332898,-27.1076209529245)) ;
#59148=CARTESIAN_POINT('Ctrl Pts',(16.3186460115184,-3.85417475315424,-27.1325070981648)) ;
#59149=CARTESIAN_POINT('Ctrl Pts',(16.3482808560405,-4.13545130036397,-27.1825154360538)) ;
#59150=CARTESIAN_POINT('Ctrl Pts',(16.3631790444222,-4.27678028782789,-27.2076375978574)) ;
#59151=CARTESIAN_POINT('Ctrl Pts',(16.3931221850076,-4.56071342667109,-27.2581011640566)) ;
#59152=CARTESIAN_POINT('Ctrl Pts',(16.408167159986,-4.70331757714046,-27.2834425545297)) ;
#59153=CARTESIAN_POINT('Ctrl Pts',(16.4383903366365,-4.98969477637851,-27.3343270936616)) ;
#59154=CARTESIAN_POINT('Ctrl Pts',(16.4535685497435,-5.13346782516221,-27.3598702354439)) ;
#59155=CARTESIAN_POINT('Ctrl Pts',(16.4840453325162,-5.4220765581703,-27.411140392136)) ;
#59156=CARTESIAN_POINT('Ctrl Pts',(16.4993439077866,-5.56691224239239,-27.4368674036729)) ;
#59157=CARTESIAN_POINT('Ctrl Pts',(16.5300489684253,-5.85753998390375,-27.4884871600178)) ;
#59158=CARTESIAN_POINT('Ctrl Pts',(16.5454554548018,-6.00333204119435,-27.5143799042186)) ;
#59159=CARTESIAN_POINT('Ctrl Pts',(16.591818523408,-6.4419833796166,-27.5922792779561)) ;
#59160=CARTESIAN_POINT('Ctrl Pts',(16.6229186490035,-6.73611782260147,-27.6445070872715)) ;
#59161=CARTESIAN_POINT('Ctrl Pts',(16.6854064677895,-7.32693704076666,-27.7494047781817)) ;
#59162=CARTESIAN_POINT('Ctrl Pts',(16.7167941940568,-7.62362181598063,-27.802074639883)) ;
#59163=CARTESIAN_POINT('Ctrl Pts',(16.779763714813,-8.21869159784999,-27.9077076626911)) ;
#59164=CARTESIAN_POINT('Ctrl Pts',(16.8113455256892,-8.51707660450211,-27.9606708139371)) ;
#59165=CARTESIAN_POINT('Ctrl Pts',(16.8746106604458,-9.11469674930695,-28.0667410750769)) ;
#59166=CARTESIAN_POINT('Ctrl Pts',(16.9062939919982,-9.41393188746664,-28.1198481803558)) ;
#59167=CARTESIAN_POINT('Ctrl Pts',(17.001358320318,-10.3116373501377,-28.2791608835402)) ;
#59168=CARTESIAN_POINT('Ctrl Pts',(17.0647535138763,-10.9101077074106,-28.3853579474179)) ;
#59169=CARTESIAN_POINT('Ctrl Pts',(17.1908503647206,-12.1002477005039,-28.5965291458614)) ;
#59170=CARTESIAN_POINT('Ctrl Pts',(17.2535520883831,-12.6919173363758,-28.7015032405009)) ;
#59171=CARTESIAN_POINT('Ctrl Pts',(17.3785914021686,-13.871632628226,-28.9107964804685)) ;
#59172=CARTESIAN_POINT('Ctrl Pts',(17.4409045653392,-14.4594442698531,-29.0150738827972)) ;
#59173=CARTESIAN_POINT('Ctrl Pts',(17.5021003260697,-15.0366437072153,-29.1174641239733)) ;
#59174=CARTESIAN_POINT('Ctrl Pts',(17.5274987345495,-15.0366437072153,-29.1021824086278)) ;
#59175=CARTESIAN_POINT('Ctrl Pts',(17.526462169319,-15.0269621479894,-29.1004710648072)) ;
#59176=CARTESIAN_POINT('Ctrl Pts',(17.5254252822432,-15.0172776030755,-29.0987591945383)) ;
#59177=CARTESIAN_POINT('Ctrl Pts',(17.4635886137329,-14.4397231681225,-28.9966689555074)) ;
#59178=CARTESIAN_POINT('Ctrl Pts',(17.4016894411209,-13.8616550702235,-28.8944924373392)) ;
#59179=CARTESIAN_POINT('Ctrl Pts',(17.2764143764457,-12.6919173364626,-28.687747458202)) ;
#59180=CARTESIAN_POINT('Ctrl Pts',(17.2130385160889,-12.1002477006036,-28.5831789781565)) ;
#59181=CARTESIAN_POINT('Ctrl Pts',(17.0855310481079,-10.9101077075362,-28.3728565198898)) ;
#59182=CARTESIAN_POINT('Ctrl Pts',(17.0213995068512,-10.3116373502763,-28.2671025017254)) ;
#59183=CARTESIAN_POINT('Ctrl Pts',(16.9251737485511,-9.41393188762483,-28.1084886077789)) ;
#59184=CARTESIAN_POINT('Ctrl Pts',(16.89309372132,-9.11469674947166,-28.0556201863721)) ;
#59185=CARTESIAN_POINT('Ctrl Pts',(16.8290132911686,-8.51707660467983,-27.9500404721984)) ;
#59186=CARTESIAN_POINT('Ctrl Pts',(16.7970128959182,-8.21869159803422,-27.8973291748155)) ;
#59187=CARTESIAN_POINT('Ctrl Pts',(16.7331803030063,-7.62362181617781,-27.7922154452969)) ;
#59188=CARTESIAN_POINT('Ctrl Pts',(16.7013481217343,-7.32693704097029,-27.7398130033007)) ;
#59189=CARTESIAN_POINT('Ctrl Pts',(16.6379395701423,-6.73611782281798,-27.6354692989421)) ;
#59190=CARTESIAN_POINT('Ctrl Pts',(16.6063632328931,-6.44198337983951,-27.5835280166735)) ;
#59191=CARTESIAN_POINT('Ctrl Pts',(16.5592550506141,-6.00333204142681,-27.5060769629603)) ;
#59192=CARTESIAN_POINT('Ctrl Pts',(16.5435950275102,-5.85753998413939,-27.4803367667477)) ;
#59193=CARTESIAN_POINT('Ctrl Pts',(16.5123708606242,-5.56691224263436,-27.4290293462702)) ;
#59194=CARTESIAN_POINT('Ctrl Pts',(16.4968067178516,-5.42207655841544,-27.4034621213986)) ;
#59195=CARTESIAN_POINT('Ctrl Pts',(16.4657844991903,-5.13346782541362,-27.3525201425934)) ;
#59196=CARTESIAN_POINT('Ctrl Pts',(16.4503264289016,-4.98969477663306,-27.3271453852913)) ;
#59197=CARTESIAN_POINT('Ctrl Pts',(16.4195261167511,-4.70331757740126,-27.2766080970697)) ;
#59198=CARTESIAN_POINT('Ctrl Pts',(16.4041838863201,-4.56071342693497,-27.2514455592689)) ;
#59199=CARTESIAN_POINT('Ctrl Pts',(16.3736243375693,-4.27678028809796,-27.2013528735587)) ;
#59200=CARTESIAN_POINT('Ctrl Pts',(16.3584070422223,-4.13545130063712,-27.1764227120465)) ;
#59201=CARTESIAN_POINT('Ctrl Pts',(16.3281052846885,-3.85417475343352,-27.1268156424043)) ;
#59202=CARTESIAN_POINT('Ctrl Pts',(16.3130208737795,-3.7142271936113,-27.1021387034025)) ;
#59203=CARTESIAN_POINT('Ctrl Pts',(16.2904981790424,-3.50542162501146,-27.0653298720066)) ;
#59204=CARTESIAN_POINT('Ctrl Pts',(16.2830079109946,-3.4360057308309,-27.0530947051822)) ;
#59205=CARTESIAN_POINT('Ctrl Pts',(16.2680622843419,-3.2975591503841,-27.0286962726957)) ;
#59206=CARTESIAN_POINT('Ctrl Pts',(16.2606069274919,-3.22852846411439,-27.0165330059779)) ;
#59207=CARTESIAN_POINT('Ctrl Pts',(16.2457309721133,-3.09086558422325,-26.9922816686795)) ;
#59208=CARTESIAN_POINT('Ctrl Pts',(16.2383103872221,-3.02223339061542,-26.9801935898972)) ;
#59209=CARTESIAN_POINT('Ctrl Pts',(16.2235030435901,-2.88538078231715,-26.9560963937571)) ;
#59210=CARTESIAN_POINT('Ctrl Pts',(16.2161163184728,-2.81716036755398,-26.9440872561512)) ;
#59211=CARTESIAN_POINT('Ctrl Pts',(16.2020179696739,-2.68708327265388,-26.9211976084717)) ;
#59212=CARTESIAN_POINT('Ctrl Pts',(16.194948247823,-2.6219106676199,-26.9097328152556)) ;
#59213=CARTESIAN_POINT('Ctrl Pts',(16.1840752739186,-2.52182434607447,-26.8921357790644)) ;
#59214=CARTESIAN_POINT('Ctrl Pts',(16.180406192602,-2.48807433664905,-26.8862034742322)) ;
#59215=CARTESIAN_POINT('Ctrl Pts',(16.1730188395042,-2.42018646006518,-26.8742749169197)) ;
#59216=CARTESIAN_POINT('Ctrl Pts',(16.1693005830549,-2.38604859286116,-26.8682786552036)) ;
#59217=CARTESIAN_POINT('Ctrl Pts',(16.1618544958971,-2.3177729495731,-26.8562919143886)) ;
#59218=CARTESIAN_POINT('Ctrl Pts',(16.1581267046257,-2.28363518715392,-26.8503014148569)) ;
#59219=CARTESIAN_POINT('Ctrl Pts',(16.1525564427381,-2.23271957894245,-26.8413729672555)) ;
#59220=CARTESIAN_POINT('Ctrl Pts',(16.1507032440341,-2.215796215514,-26.8384063777284)) ;
#59221=CARTESIAN_POINT('Ctrl Pts',(16.1470084290761,-2.18209499271471,-26.8325013228036)) ;
#59222=CARTESIAN_POINT('Ctrl Pts',(16.1451668147577,-2.165317133336,-26.82956285624)) ;
#59223=CARTESIAN_POINT('Ctrl Pts',(16.1414992639685,-2.13195541226357,-26.8237232789466)) ;
#59224=CARTESIAN_POINT('Ctrl Pts',(16.1396733431141,-2.1153715544092,-26.8208221597469)) ;
#59225=CARTESIAN_POINT('Ctrl Pts',(16.136040571677,-2.0824463337016,-26.8150669327407)) ;
#59226=CARTESIAN_POINT('Ctrl Pts',(16.1342337624648,-2.06610497064345,-26.8122127999931)) ;
#59227=CARTESIAN_POINT('Ctrl Pts',(16.1315392659603,-2.04181117001441,-26.8079747807405)) ;
#59228=CARTESIAN_POINT('Ctrl Pts',(16.130643698243,-2.03374961132952,-26.8065693176076)) ;
#59229=CARTESIAN_POINT('Ctrl Pts',(16.1288576745114,-2.01770530625544,-26.8037743238924)) ;
#59230=CARTESIAN_POINT('Ctrl Pts',(16.1279672191938,-2.00972255986181,-26.8023847928903)) ;
#59231=CARTESIAN_POINT('Ctrl Pts',(16.1261908623183,-1.99384194490789,-26.7996234620433)) ;
#59232=CARTESIAN_POINT('Ctrl Pts',(16.1253049854103,-1.98594407652206,-26.7982516474091)) ;
#59233=CARTESIAN_POINT('Ctrl Pts',(16.1239784538382,-1.97416548617237,-26.7962090029555)) ;
#59234=CARTESIAN_POINT('Ctrl Pts',(16.1235366471204,-1.97025065819767,-26.7955306405245)) ;
#59235=CARTESIAN_POINT('Ctrl Pts',(16.1226533878464,-1.96244450023135,-26.7941793698772)) ;
#59236=CARTESIAN_POINT('Ctrl Pts',(16.122211936814,-1.95855317022654,-26.7935064607409)) ;
#59237=CARTESIAN_POINT('Ctrl Pts',(16.1213281970955,-1.9507900367832,-26.7921658559373)) ;
#59238=CARTESIAN_POINT('Ctrl Pts',(16.1208624448328,-1.94671197294882,-26.7914625314001)) ;
#59239=CARTESIAN_POINT('Ctrl Pts',(16.1199034641384,-1.93836188169201,-26.7900256335297)) ;
#59240=CARTESIAN_POINT('Ctrl Pts',(16.1194102982851,-1.93408985359028,-26.7892920223804)) ;
#59241=CARTESIAN_POINT('Ctrl Pts',(16.1186635384765,-1.9276820743651,-26.7881958874659)) ;
#59242=CARTESIAN_POINT('Ctrl Pts',(16.1184134372312,-1.92554620504717,-26.7878312337004)) ;
#59243=CARTESIAN_POINT('Ctrl Pts',(16.1179126494524,-1.92129885207443,-26.7871081597253)) ;
#59244=CARTESIAN_POINT('Ctrl Pts',(16.1176619935634,-1.91918736796419,-26.7867497209677)) ;
#59245=CARTESIAN_POINT('Ctrl Pts',(16.1172862550928,-1.91605664429787,-26.7862207189719)) ;
#59246=CARTESIAN_POINT('Ctrl Pts',(16.1171610403001,-1.91501915730528,-26.7860458343169)) ;
#59247=CARTESIAN_POINT('Ctrl Pts',(16.1169105660688,-1.91295939100032,-26.7856997596984)) ;
#59248=CARTESIAN_POINT('Ctrl Pts',(16.1167853088843,-1.91193711164353,-26.7855285683681)) ;
#59249=CARTESIAN_POINT('Ctrl Pts',(16.1165342706096,-1.90991080049551,-26.7851909019278)) ;
#59250=CARTESIAN_POINT('Ctrl Pts',(16.1164085234018,-1.90890677053132,-26.7850244068722)) ;
#59251=CARTESIAN_POINT('Ctrl Pts',(16.116218407116,-1.90741670517188,-26.7847794180852)) ;
#59252=CARTESIAN_POINT('Ctrl Pts',(16.1161547773415,-1.9069226804876,-26.7846985526516)) ;
#59253=CARTESIAN_POINT('Ctrl Pts',(16.1160265200478,-1.90594034744944,-26.7845388007874)) ;
#59254=CARTESIAN_POINT('Ctrl Pts',(16.1159619131579,-1.90545203844624,-26.7844599017879)) ;
#59255=CARTESIAN_POINT('Ctrl Pts',(16.1158625385309,-1.90471721841522,-26.7843424676508)) ;
#59256=CARTESIAN_POINT('Ctrl Pts',(16.1158267232252,-1.90445522424116,-26.7843008285476)) ;
#59257=CARTESIAN_POINT('Ctrl Pts',(16.1157520891995,-1.90391896164507,-26.7842163970993)) ;
#59258=CARTESIAN_POINT('Ctrl Pts',(16.1157132748072,-1.90364469303768,-26.7841736021057)) ;
#59259=CARTESIAN_POINT('Ctrl Pts',(16.1156333538959,-1.9030964687972,-26.7840894667296)) ;
#59260=CARTESIAN_POINT('Ctrl Pts',(16.1155923338751,-1.90282255200049,-26.7840480836694)) ;
#59261=CARTESIAN_POINT('Ctrl Pts',(16.1153534832311,-1.90163369505953,-26.7839050636273)) ;
#59262=CARTESIAN_POINT('Ctrl Pts',(16.1153437024324,-1.9015850120406,-26.7838992070375)) ;
#59263=CARTESIAN_POINT('Ctrl Pts',(16.1153339216337,-1.90153632902166,-26.7838933504477)) ;
#59264=CARTESIAN_POINT('',(3.65837019749608,-15.0366437072151,-33.7752359034359)) ;
#59265=CARTESIAN_POINT('',(3.68783779512015,-15.0366437072151,-33.7720311090636)) ;
#59266=CARTESIAN_POINT('Origin',(-0.147684368304155,-21.6462763158694,1.35793534153108)) ;
#59267=CARTESIAN_POINT('',(3.37961603007408,-1.90153624332578,-31.075056312033)) ;
#59268=CARTESIAN_POINT('Ctrl Pts',(3.37961603187484,-1.90153633508113,-31.0750563309111)) ;
#59269=CARTESIAN_POINT('Ctrl Pts',(3.37961070599222,-1.90158489145841,-31.0750670039238)) ;
#59270=CARTESIAN_POINT('Ctrl Pts',(3.37951986530706,-1.90241309119405,-31.0752490477001)) ;
#59271=CARTESIAN_POINT('Ctrl Pts',(3.37950436522705,-1.90281047539216,-31.0753333407487)) ;
#59272=CARTESIAN_POINT('Ctrl Pts',(3.37949676124729,-1.9030817925977,-31.0753905685281)) ;
#59273=CARTESIAN_POINT('Ctrl Pts',(3.37948405658615,-1.90362481732619,-31.0755048329751)) ;
#59274=CARTESIAN_POINT('Ctrl Pts',(3.37947905017671,-1.90389648606574,-31.0755618513277)) ;
#59275=CARTESIAN_POINT('Ctrl Pts',(3.37947071353972,-1.90442766694489,-31.0756731786513)) ;
#59276=CARTESIAN_POINT('Ctrl Pts',(3.37946738820882,-1.9046871792651,-31.0757274871272)) ;
#59277=CARTESIAN_POINT('Ctrl Pts',(3.37945930658739,-1.90541496833161,-31.075879657174)) ;
#59278=CARTESIAN_POINT('Ctrl Pts',(3.37945558758785,-1.90589858091376,-31.0759805939111)) ;
#59279=CARTESIAN_POINT('Ctrl Pts',(3.37945008307113,-1.90687146640829,-31.0761834337627)) ;
#59280=CARTESIAN_POINT('Ctrl Pts',(3.37944832151258,-1.90736073997115,-31.0762853344068)) ;
#59281=CARTESIAN_POINT('Ctrl Pts',(3.37944508902581,-1.90883647538957,-31.0765924584461)) ;
#59282=CARTESIAN_POINT('Ctrl Pts',(3.37944563120107,-1.90983084996186,-31.0767991077804)) ;
#59283=CARTESIAN_POINT('Ctrl Pts',(3.37944989084143,-1.91183767529128,-31.0772158187512)) ;
#59284=CARTESIAN_POINT('Ctrl Pts',(3.37945364719749,-1.91285012422377,-31.0774258757787)) ;
#59285=CARTESIAN_POINT('Ctrl Pts',(3.37946341359751,-1.91489008382497,-31.0778488757296)) ;
#59286=CARTESIAN_POINT('Ctrl Pts',(3.3794694261378,-1.91591759453621,-31.0780618183902)) ;
#59287=CARTESIAN_POINT('Ctrl Pts',(3.37949000589426,-1.9190182143266,-31.0787041299186)) ;
#59288=CARTESIAN_POINT('Ctrl Pts',(3.37950706889375,-1.92110939581349,-31.0791369842042)) ;
#59289=CARTESIAN_POINT('Ctrl Pts',(3.37954533910382,-1.92531591015439,-31.0800072625959)) ;
#59290=CARTESIAN_POINT('Ctrl Pts',(3.37956658180458,-1.92743124346434,-31.080444682937)) ;
#59291=CARTESIAN_POINT('Ctrl Pts',(3.37963442654588,-1.93377741462869,-31.0817565318447)) ;
#59292=CARTESIAN_POINT('Ctrl Pts',(3.37968507843149,-1.93800837065686,-31.0826305445298)) ;
#59293=CARTESIAN_POINT('Ctrl Pts',(3.37978980881172,-1.94627818463165,-31.0843382643264)) ;
#59294=CARTESIAN_POINT('Ctrl Pts',(3.37984395962429,-1.95031704325728,-31.0851719637139)) ;
#59295=CARTESIAN_POINT('Ctrl Pts',(3.3799503650075,-1.95800520795894,-31.0867585894296)) ;
#59296=CARTESIAN_POINT('Ctrl Pts',(3.3800054657301,-1.96185878993651,-31.0875536706246)) ;
#59297=CARTESIAN_POINT('Ctrl Pts',(3.38011866494425,-1.96958922400625,-31.0891483443258)) ;
#59298=CARTESIAN_POINT('Ctrl Pts',(3.3801767652232,-1.97346607611177,-31.0899479366401)) ;
#59299=CARTESIAN_POINT('Ctrl Pts',(3.38035473269316,-1.98513040811581,-31.092353336025)) ;
#59300=CARTESIAN_POINT('Ctrl Pts',(3.38047821962445,-1.99295166328761,-31.0939657705512)) ;
#59301=CARTESIAN_POINT('Ctrl Pts',(3.38073219781414,-2.00867822864612,-31.0972073510004)) ;
#59302=CARTESIAN_POINT('Ctrl Pts',(3.38086271750251,-2.01658353865841,-31.0988364937951)) ;
#59303=CARTESIAN_POINT('Ctrl Pts',(3.38112929199853,-2.03247220660011,-31.1021104018258)) ;
#59304=CARTESIAN_POINT('Ctrl Pts',(3.38126534761985,-2.04045556453403,-31.1037551669739)) ;
#59305=CARTESIAN_POINT('Ctrl Pts',(3.3816803546736,-2.0645137045524,-31.10871118306)) ;
#59306=CARTESIAN_POINT('Ctrl Pts',(3.38196604522678,-2.08069654939365,-31.1120441649112)) ;
#59307=CARTESIAN_POINT('Ctrl Pts',(3.38255050826333,-2.11330238176182,-31.1187586261777)) ;
#59308=CARTESIAN_POINT('Ctrl Pts',(3.38284932852915,-2.12972536949358,-31.1221401004387)) ;
#59309=CARTESIAN_POINT('Ctrl Pts',(3.38345698968157,-2.16276346879482,-31.128941897414)) ;
#59310=CARTESIAN_POINT('Ctrl Pts',(3.38376584804614,-2.17937857652572,-31.1323622174295)) ;
#59311=CARTESIAN_POINT('Ctrl Pts',(3.38439130595124,-2.21275288488517,-31.1392319692574)) ;
#59312=CARTESIAN_POINT('Ctrl Pts',(3.3847079077424,-2.22951208552169,-31.1426814008264)) ;
#59313=CARTESIAN_POINT('Ctrl Pts',(3.38566651923717,-2.27993379421205,-31.1530586943963)) ;
#59314=CARTESIAN_POINT('Ctrl Pts',(3.38631726306848,-2.31374040875672,-31.1600155630294)) ;
#59315=CARTESIAN_POINT('Ctrl Pts',(3.38762973138084,-2.38135375628433,-31.1739281306989)) ;
#59316=CARTESIAN_POINT('Ctrl Pts',(3.38829149941384,-2.41516047560426,-31.1808838221583)) ;
#59317=CARTESIAN_POINT('Ctrl Pts',(3.38961550071907,-2.48238981945739,-31.1947153097383)) ;
#59318=CARTESIAN_POINT('Ctrl Pts',(3.39027775169458,-2.51581244403611,-31.201591103943)) ;
#59319=CARTESIAN_POINT('Ctrl Pts',(3.39225062944442,-2.61492790016553,-31.2219804336516)) ;
#59320=CARTESIAN_POINT('Ctrl Pts',(3.39354726626446,-2.67946831375413,-31.2352559286588)) ;
#59321=CARTESIAN_POINT('Ctrl Pts',(3.39614778446036,-2.80821979180197,-31.2617376664407)) ;
#59322=CARTESIAN_POINT('Ctrl Pts',(3.3975194687046,-2.87571441576423,-31.2756191140077)) ;
#59323=CARTESIAN_POINT('Ctrl Pts',(3.40028344398628,-3.01111106169542,-31.3034644569785)) ;
#59324=CARTESIAN_POINT('Ctrl Pts',(3.4016757737032,-3.07901308373674,-31.3174283481908)) ;
#59325=CARTESIAN_POINT('Ctrl Pts',(3.40447808763379,-3.21521138105106,-31.3454361670284)) ;
#59326=CARTESIAN_POINT('Ctrl Pts',(3.40588808753438,-3.2835076563105,-31.3594800929445)) ;
#59327=CARTESIAN_POINT('Ctrl Pts',(3.40872367041719,-3.4204813166111,-31.3876454742405)) ;
#59328=CARTESIAN_POINT('Ctrl Pts',(3.41014925541447,-3.4891587016557,-31.4017669294009)) ;
#59329=CARTESIAN_POINT('Ctrl Pts',(3.41444704959774,-3.69574280763306,-31.4442437450053)) ;
#59330=CARTESIAN_POINT('Ctrl Pts',(3.41734019001168,-3.83420147875592,-31.4727115671767)) ;
#59331=CARTESIAN_POINT('Ctrl Pts',(3.42317344443391,-4.11248555184698,-31.5299262156988)) ;
#59332=CARTESIAN_POINT('Ctrl Pts',(3.42611361752539,-4.25231095389446,-31.55867303564)) ;
#59333=CARTESIAN_POINT('Ctrl Pts',(3.43203473233886,-4.53322335570595,-31.6164244996989)) ;
#59334=CARTESIAN_POINT('Ctrl Pts',(3.4350157003956,-4.67431035456218,-31.6454291407638)) ;
#59335=CARTESIAN_POINT('Ctrl Pts',(3.44101350143713,-4.95764081489597,-31.7036749251378)) ;
#59336=CARTESIAN_POINT('Ctrl Pts',(3.44403034759642,-5.09988427638858,-31.7329160670173)) ;
#59337=CARTESIAN_POINT('Ctrl Pts',(3.45009576986787,-5.38542252965196,-31.7916134480566)) ;
#59338=CARTESIAN_POINT('Ctrl Pts',(3.45314435244133,-5.52871732142045,-31.8210696865129)) ;
#59339=CARTESIAN_POINT('Ctrl Pts',(3.45926960099568,-5.81625310337682,-31.8801758027233)) ;
#59340=CARTESIAN_POINT('Ctrl Pts',(3.46234626814327,-5.96049409356606,-31.90982568035)) ;
#59341=CARTESIAN_POINT('Ctrl Pts',(3.47161340231309,-6.39447866448406,-31.9990335333828)) ;
#59342=CARTESIAN_POINT('Ctrl Pts',(3.47784092628434,-6.68548384087354,-32.0588497362073)) ;
#59343=CARTESIAN_POINT('Ctrl Pts',(3.49037064512373,-7.27001739345534,-32.1789985378797)) ;
#59344=CARTESIAN_POINT('Ctrl Pts',(3.49667287813247,-7.56354576968126,-32.2393311325864)) ;
#59345=CARTESIAN_POINT('Ctrl Pts',(3.50932984594644,-8.15228466530568,-32.3603402921398)) ;
#59346=CARTESIAN_POINT('Ctrl Pts',(3.5156845996516,-8.44749518470088,-32.4210168549303)) ;
#59347=CARTESIAN_POINT('Ctrl Pts',(3.52842552872783,-9.03875731084587,-32.5425414065042)) ;
#59348=CARTESIAN_POINT('Ctrl Pts',(3.53481171294786,-9.33480891760259,-32.6033893943262)) ;
#59349=CARTESIAN_POINT('Ctrl Pts',(3.55398681249754,-10.222963786029,-32.785931568223)) ;
#59350=CARTESIAN_POINT('Ctrl Pts',(3.56679211841551,-10.8150670804398,-32.9076239785171)) ;
#59351=CARTESIAN_POINT('Ctrl Pts',(3.59228823476391,-11.9925453007398,-33.1496225734659)) ;
#59352=CARTESIAN_POINT('Ctrl Pts',(3.60497912176864,-12.5779202266805,-33.2699287498025)) ;
#59353=CARTESIAN_POINT('Ctrl Pts',(3.63009196367396,-13.7352132465282,-33.5077729753066)) ;
#59354=CARTESIAN_POINT('Ctrl Pts',(3.64251395514895,-14.3071313404322,-33.6253110204958)) ;
#59355=CARTESIAN_POINT('Ctrl Pts',(3.65594235487389,-14.9249537984812,-33.7522821058483)) ;
#59356=CARTESIAN_POINT('Ctrl Pts',(3.65715735966845,-14.9808505488474,-33.7637696540393)) ;
#59357=CARTESIAN_POINT('Ctrl Pts',(3.65837019675597,-15.0366437072147,-33.775235903516)) ;
#59358=CARTESIAN_POINT('Ctrl Pts',(3.68783779586043,-15.0366437072147,-33.7720311089827)) ;
#59359=CARTESIAN_POINT('Ctrl Pts',(3.68655737279354,-14.9808505488608,-33.7605722099269)) ;
#59360=CARTESIAN_POINT('Ctrl Pts',(3.6852744881599,-14.924953798508,-33.7490920441161)) ;
#59361=CARTESIAN_POINT('Ctrl Pts',(3.67109390924987,-14.3071313404863,-33.6222027631854)) ;
#59362=CARTESIAN_POINT('Ctrl Pts',(3.65795827615197,-13.7352132465962,-33.5047423312028)) ;
#59363=CARTESIAN_POINT('Ctrl Pts',(3.63135451591116,-12.5779202267768,-33.2670602528451)) ;
#59364=CARTESIAN_POINT('Ctrl Pts',(3.61788642534454,-11.9925453008504,-33.1468386024926)) ;
#59365=CARTESIAN_POINT('Ctrl Pts',(3.59076391217546,-10.8150670805791,-32.9050168888634)) ;
#59366=CARTESIAN_POINT('Ctrl Pts',(3.57710956614513,-10.2229637861827,-32.7834168172492)) ;
#59367=CARTESIAN_POINT('Ctrl Pts',(3.55659519104407,-9.33480891777804,-32.6010202983507)) ;
#59368=CARTESIAN_POINT('Ctrl Pts',(3.54975155110104,-9.03875731102854,-32.5402220618383)) ;
#59369=CARTESIAN_POINT('Ctrl Pts',(3.53607041798801,-8.44749518489797,-32.4187997636185)) ;
#59370=CARTESIAN_POINT('Ctrl Pts',(3.52923293366762,-8.15228466551,-32.3581757009477)) ;
#59371=CARTESIAN_POINT('Ctrl Pts',(3.51558059630923,-7.56354576989996,-32.2372747943589)) ;
#59372=CARTESIAN_POINT('Ctrl Pts',(3.50876576216914,-7.2700173936812,-32.1769979483863)) ;
#59373=CARTESIAN_POINT('Ctrl Pts',(3.49517410235908,-6.68548384111368,-32.0569646397574)) ;
#59374=CARTESIAN_POINT('Ctrl Pts',(3.48839731482568,-6.39447866473132,-31.9972081729466)) ;
#59375=CARTESIAN_POINT('Ctrl Pts',(3.47827073711185,-5.96049409382388,-31.9080937900342)) ;
#59376=CARTESIAN_POINT('Ctrl Pts',(3.47490162625046,-5.81625310363817,-31.8784757175788)) ;
#59377=CARTESIAN_POINT('Ctrl Pts',(3.46817760207663,-5.52871732168881,-31.8194347221429)) ;
#59378=CARTESIAN_POINT('Ctrl Pts',(3.46482268993128,-5.38542252992385,-31.7900117990359)) ;
#59379=CARTESIAN_POINT('Ctrl Pts',(3.45812810415939,-5.09988427666742,-31.7313828436523)) ;
#59380=CARTESIAN_POINT('Ctrl Pts',(3.45478843699215,-4.95764081517829,-31.7021768106739)) ;
#59381=CARTESIAN_POINT('Ctrl Pts',(3.44812489087114,-4.6743103548514,-31.644003430442)) ;
#59382=CARTESIAN_POINT('Ctrl Pts',(3.44480102509296,-4.53322335599863,-31.6150360817525)) ;
#59383=CARTESIAN_POINT('Ctrl Pts',(3.4381688498808,-4.25231095419401,-31.5573619501736)) ;
#59384=CARTESIAN_POINT('Ctrl Pts',(3.4348605668216,-4.11248555214992,-31.5286551646046)) ;
#59385=CARTESIAN_POINT('Ctrl Pts',(3.42825798481763,-3.83420147906566,-31.4715241855007)) ;
#59386=CARTESIAN_POINT('Ctrl Pts',(3.42496374495564,-3.69574280794619,-31.4430999855238)) ;
#59387=CARTESIAN_POINT('Ctrl Pts',(3.42002979935007,-3.48915870197386,-31.4006923555569)) ;
#59388=CARTESIAN_POINT('Ctrl Pts',(3.41838635952705,-3.42048131693095,-31.386594593537)) ;
#59389=CARTESIAN_POINT('Ctrl Pts',(3.41510092364216,-3.28350765663369,-31.358478136704)) ;
#59390=CARTESIAN_POINT('Ctrl Pts',(3.41345892959589,-3.21521138137592,-31.3444594416721)) ;
#59391=CARTESIAN_POINT('Ctrl Pts',(3.41017487383933,-3.07901308406493,-31.3165040154161)) ;
#59392=CARTESIAN_POINT('Ctrl Pts',(3.40853282782131,-3.01111106202524,-31.3025672824885)) ;
#59393=CARTESIAN_POINT('Ctrl Pts',(3.40524625726093,-2.87571441609737,-31.27477877518)) ;
#59394=CARTESIAN_POINT('Ctrl Pts',(3.40360177139038,-2.80821979213676,-31.2609269965782)) ;
#59395=CARTESIAN_POINT('Ctrl Pts',(3.40044870008814,-2.67946831411711,-31.234505352574)) ;
#59396=CARTESIAN_POINT('Ctrl Pts',(3.39886118325269,-2.61492790055638,-31.2212614926806)) ;
#59397=CARTESIAN_POINT('Ctrl Pts',(3.39640483303503,-2.51581244446976,-31.2009247437805)) ;
#59398=CARTESIAN_POINT('Ctrl Pts',(3.39557350845141,-2.48238981990544,-31.1940673374417)) ;
#59399=CARTESIAN_POINT('Ctrl Pts',(3.39389319436904,-2.41516047608134,-31.1802746012175)) ;
#59400=CARTESIAN_POINT('Ctrl Pts',(3.39304422256571,-2.38135375677605,-31.1733392693982)) ;
#59401=CARTESIAN_POINT('Ctrl Pts',(3.3913352153028,-2.31374040927761,-31.1594698279445)) ;
#59402=CARTESIAN_POINT('Ctrl Pts',(3.39047522401304,-2.2799337947475,-31.1525357163469)) ;
#59403=CARTESIAN_POINT('Ctrl Pts',(3.38918061233769,-2.2295120860789,-31.1421949650033)) ;
#59404=CARTESIAN_POINT('Ctrl Pts',(3.38874828632986,-2.21275288544962,-31.1387581192029)) ;
#59405=CARTESIAN_POINT('Ctrl Pts',(3.38788232780283,-2.17937857710456,-31.1319145233968)) ;
#59406=CARTESIAN_POINT('Ctrl Pts',(3.38744869751914,-2.16276346938089,-31.1285077731469)) ;
#59407=CARTESIAN_POINT('Ctrl Pts',(3.38657996660205,-2.12972537009392,-31.1217343692224)) ;
#59408=CARTESIAN_POINT('Ctrl Pts',(3.38614488362664,-2.11330238236914,-31.1183677144256)) ;
#59409=CARTESIAN_POINT('Ctrl Pts',(3.38527227154898,-2.08069655001507,-31.1116845912588)) ;
#59410=CARTESIAN_POINT('Ctrl Pts',(3.3848347902236,-2.06451370518087,-31.1083681176504)) ;
#59411=CARTESIAN_POINT('Ctrl Pts',(3.38417469768363,-2.04045556517289,-31.1034387562193)) ;
#59412=CARTESIAN_POINT('Ctrl Pts',(3.38395399652491,-2.03247220724235,-31.101803196829)) ;
#59413=CARTESIAN_POINT('Ctrl Pts',(3.38351054520699,-2.01658353930749,-31.0985485253133)) ;
#59414=CARTESIAN_POINT('Ctrl Pts',(3.38328779585336,-2.00867822929873,-31.0969294130999)) ;
#59415=CARTESIAN_POINT('Ctrl Pts',(3.38283899220078,-1.992951663947,-31.0937090211981)) ;
#59416=CARTESIAN_POINT('Ctrl Pts',(3.38261296631749,-1.98513040877856,-31.0921077384556)) ;
#59417=CARTESIAN_POINT('Ctrl Pts',(3.3822696832439,-1.97346607677957,-31.0897203182271)) ;
#59418=CARTESIAN_POINT('Ctrl Pts',(3.38215453645563,-1.96958922467574,-31.0889269300949)) ;
#59419=CARTESIAN_POINT('Ctrl Pts',(3.38192228142768,-1.96185879060935,-31.0873452044946)) ;
#59420=CARTESIAN_POINT('Ctrl Pts',(3.38180517497239,-1.9580052086334,-31.0865568668297)) ;
#59421=CARTESIAN_POINT('Ctrl Pts',(3.38156801502377,-1.95031704378451,-31.0849844614994)) ;
#59422=CARTESIAN_POINT('Ctrl Pts',(3.38144167908556,-1.94627818500258,-31.0841586126848)) ;
#59423=CARTESIAN_POINT('Ctrl Pts',(3.38117685164134,-1.93800837070766,-31.0824683044267)) ;
#59424=CARTESIAN_POINT('Ctrl Pts',(3.38103843247478,-1.93377741451519,-31.0816038369745)) ;
#59425=CARTESIAN_POINT('Ctrl Pts',(3.3808226822932,-1.92743124310526,-31.0803080737017)) ;
#59426=CARTESIAN_POINT('Ctrl Pts',(3.38074939587864,-1.92531590971377,-31.0798763134386)) ;
#59427=CARTESIAN_POINT('Ctrl Pts',(3.3805996872188,-1.92110939521005,-31.0790181546749)) ;
#59428=CARTESIAN_POINT('Ctrl Pts',(3.38052330043609,-1.91901821364194,-31.0785917522226)) ;
#59429=CARTESIAN_POINT('Ctrl Pts',(3.38040532104915,-1.91591759373161,-31.0779600335174)) ;
#59430=CARTESIAN_POINT('Ctrl Pts',(3.38036541656933,-1.91489008298177,-31.0777507768194)) ;
#59431=CARTESIAN_POINT('Ctrl Pts',(3.38028402215018,-1.91285012330151,-31.0773355668686)) ;
#59432=CARTESIAN_POINT('Ctrl Pts',(3.38024253472088,-1.91183767432828,-31.0771296133342)) ;
#59433=CARTESIAN_POINT('Ctrl Pts',(3.38015711422549,-1.90983084892124,-31.0767217291221)) ;
#59434=CARTESIAN_POINT('Ctrl Pts',(3.38011322012409,-1.90883647431282,-31.0765197945864)) ;
#59435=CARTESIAN_POINT('Ctrl Pts',(3.38004404061596,-1.90736073883729,-31.0762205458143)) ;
#59436=CARTESIAN_POINT('Ctrl Pts',(3.38002041465609,-1.90687146525441,-31.076121406225)) ;
#59437=CARTESIAN_POINT('Ctrl Pts',(3.37997143425657,-1.90589857972234,-31.0759244919573)) ;
#59438=CARTESIAN_POINT('Ctrl Pts',(3.37994610382241,-1.90541496712062,-31.0758267145325)) ;
#59439=CARTESIAN_POINT('Ctrl Pts',(3.37990549909382,-1.90468717824974,-31.075679839486)) ;
#59440=CARTESIAN_POINT('Ctrl Pts',(3.37989057675563,-1.90442766615567,-31.0756275156108)) ;
#59441=CARTESIAN_POINT('Ctrl Pts',(3.37985850297489,-1.90389648573531,-31.0755205832803)) ;
#59442=CARTESIAN_POINT('Ctrl Pts',(3.37984135648545,-1.90362481722601,-31.0754659742485)) ;
#59443=CARTESIAN_POINT('Ctrl Pts',(3.37980438540426,-1.90308179296695,-31.0753571124616)) ;
#59444=CARTESIAN_POINT('Ctrl Pts',(3.37978465703699,-1.90281047598829,-31.0753028573013)) ;
#59445=CARTESIAN_POINT('Ctrl Pts',(3.37962891700279,-1.90163369580955,-31.0750751686933)) ;
#59446=CARTESIAN_POINT('Ctrl Pts',(3.37962247443882,-1.90158501544534,-31.0750657498022)) ;
#59447=CARTESIAN_POINT('Ctrl Pts',(3.37961603187484,-1.90153633508113,-31.0750563309111)) ;
#59448=CARTESIAN_POINT('',(10.8335168660175,-15.0366437072153,-32.1991482053236)) ;
#59449=CARTESIAN_POINT('',(10.8616065908236,-15.0366437072153,-32.1896836750667)) ;
#59450=CARTESIAN_POINT('Origin',(-0.436147547989925,-21.6462763158694,1.29443979419782)) ;
#59451=CARTESIAN_POINT('',(9.98082102021339,-1.90153624263669,-29.622021218349)) ;
#59452=CARTESIAN_POINT('Ctrl Pts',(9.98082102598227,-1.90153633370295,-29.6220212362645)) ;
#59453=CARTESIAN_POINT('Ctrl Pts',(9.98081813631591,-1.90158489238407,-29.6220327993228)) ;
#59454=CARTESIAN_POINT('Ctrl Pts',(9.98076855213416,-1.90241811745866,-29.6222312114266)) ;
#59455=CARTESIAN_POINT('Ctrl Pts',(9.98077161916715,-1.90281781836607,-29.6223173426495)) ;
#59456=CARTESIAN_POINT('Ctrl Pts',(9.98077656137303,-1.9030907160465,-29.6223751894864)) ;
#59457=CARTESIAN_POINT('Ctrl Pts',(9.98078885651281,-1.90363690191882,-29.6224901560522)) ;
#59458=CARTESIAN_POINT('Ctrl Pts',(9.98079629783591,-1.90391015129655,-29.6225472375348)) ;
#59459=CARTESIAN_POINT('Ctrl Pts',(9.98081223588766,-1.90444442170522,-29.6226583782004)) ;
#59460=CARTESIAN_POINT('Ctrl Pts',(9.98082073741189,-1.90470544292088,-29.6227124358077)) ;
#59461=CARTESIAN_POINT('Ctrl Pts',(9.98084576989917,-1.90543750589486,-29.6228636457412)) ;
#59462=CARTESIAN_POINT('Ctrl Pts',(9.98086398323431,-1.9059239730479,-29.6229635950973)) ;
#59463=CARTESIAN_POINT('Ctrl Pts',(9.98090251341636,-1.9069026009321,-29.6231640266788)) ;
#59464=CARTESIAN_POINT('Ctrl Pts',(9.98092285312758,-1.90739476231177,-29.6232645013418)) ;
#59465=CARTESIAN_POINT('Ctrl Pts',(9.98098619086646,-1.90887920773021,-29.6235668802546)) ;
#59466=CARTESIAN_POINT('Ctrl Pts',(9.98103146973062,-1.90987945102643,-29.6237697517133)) ;
#59467=CARTESIAN_POINT('Ctrl Pts',(9.98112587712619,-1.91189812019236,-29.6241781626848)) ;
#59468=CARTESIAN_POINT('Ctrl Pts',(9.98117504274455,-1.91291654423624,-29.6243836893032)) ;
#59469=CARTESIAN_POINT('Ctrl Pts',(9.98127620660854,-1.91496854271383,-29.6247970920327)) ;
#59470=CARTESIAN_POINT('Ctrl Pts',(9.98132820728659,-1.91600211719088,-29.6250049673334)) ;
#59471=CARTESIAN_POINT('Ctrl Pts',(9.98148745395848,-1.91912103466703,-29.6256314676495)) ;
#59472=CARTESIAN_POINT('Ctrl Pts',(9.98159789961051,-1.92122455645945,-29.6260529789081)) ;
#59473=CARTESIAN_POINT('Ctrl Pts',(9.98182384020141,-1.9254558932669,-29.6268995978579)) ;
#59474=CARTESIAN_POINT('Ctrl Pts',(9.98193936909476,-1.92758370873797,-29.627324694208)) ;
#59475=CARTESIAN_POINT('Ctrl Pts',(9.98228989915498,-1.93396732640727,-29.6285986919253)) ;
#59476=CARTESIAN_POINT('Ctrl Pts',(9.9825287775567,-1.93822324679246,-29.6294463126736)) ;
#59477=CARTESIAN_POINT('Ctrl Pts',(9.98300116316303,-1.94654185476612,-29.6311012247671)) ;
#59478=CARTESIAN_POINT('Ctrl Pts',(9.98323473955941,-1.95060454303379,-29.631908492947)) ;
#59479=CARTESIAN_POINT('Ctrl Pts',(9.98368255605493,-1.95833827461836,-29.633444136637)) ;
#59480=CARTESIAN_POINT('Ctrl Pts',(9.98390871275382,-1.96221480004706,-29.6342133074122)) ;
#59481=CARTESIAN_POINT('Ctrl Pts',(9.98436493992941,-1.96999125950243,-29.6357554350788)) ;
#59482=CARTESIAN_POINT('Ctrl Pts',(9.98459501211632,-1.97389119354246,-29.6365283913966)) ;
#59483=CARTESIAN_POINT('Ctrl Pts',(9.98529025494379,-1.98562497237449,-29.6388529762627)) ;
#59484=CARTESIAN_POINT('Ctrl Pts',(9.98576040690957,-1.99349279346355,-29.6404103357754)) ;
#59485=CARTESIAN_POINT('Ctrl Pts',(9.98671119165241,-2.00931299098254,-29.6435399627786)) ;
#59486=CARTESIAN_POINT('Ctrl Pts',(9.98719185157983,-2.01726536723783,-29.645112221083)) ;
#59487=CARTESIAN_POINT('Ctrl Pts',(9.98816197703178,-2.03324863225337,-29.6482708923264)) ;
#59488=CARTESIAN_POINT('Ctrl Pts',(9.98865144333217,-2.04127952101813,-29.6498573050044)) ;
#59489=CARTESIAN_POINT('Ctrl Pts',(9.99013124687624,-2.06548089680454,-29.6546364071499)) ;
#59490=CARTESIAN_POINT('Ctrl Pts',(9.99113289198428,-2.08176008985808,-29.6578489925809)) ;
#59491=CARTESIAN_POINT('Ctrl Pts',(9.99315950009389,-2.11456004815152,-29.6643189874948)) ;
#59492=CARTESIAN_POINT('Ctrl Pts',(9.99418450879868,-2.13108081359634,-29.667576381623)) ;
#59493=CARTESIAN_POINT('Ctrl Pts',(9.99625275550711,-2.16431561192512,-29.6741271744382)) ;
#59494=CARTESIAN_POINT('Ctrl Pts',(9.9972960100553,-2.18102964097007,-29.6774205667135)) ;
#59495=CARTESIAN_POINT('Ctrl Pts',(9.9993964069154,-2.21460264965853,-29.6840342819798)) ;
#59496=CARTESIAN_POINT('Ctrl Pts',(10.0004535513673,-2.23146162930993,-29.6873546042511)) ;
#59497=CARTESIAN_POINT('Ctrl Pts',(10.0036398912599,-2.28218353274662,-29.6973421615439)) ;
#59498=CARTESIAN_POINT('Ctrl Pts',(10.0057839243653,-2.31619142072435,-29.7040360101861)) ;
#59499=CARTESIAN_POINT('Ctrl Pts',(10.0100824939905,-2.38420731512499,-29.7174201942883)) ;
#59500=CARTESIAN_POINT('Ctrl Pts',(10.0122370715424,-2.4182153078838,-29.7241105129429)) ;
#59501=CARTESIAN_POINT('Ctrl Pts',(10.0165293804464,-2.48584491142059,-29.7374125662913)) ;
#59502=CARTESIAN_POINT('Ctrl Pts',(10.0186671287307,-2.51946652224412,-29.7440242952898)) ;
#59503=CARTESIAN_POINT('Ctrl Pts',(10.0250152291373,-2.61917207551851,-29.7636286226259)) ;
#59504=CARTESIAN_POINT('Ctrl Pts',(10.0291603271039,-2.68409673841795,-29.776390398192)) ;
#59505=CARTESIAN_POINT('Ctrl Pts',(10.0374451175131,-2.81365377182546,-29.8018520291029)) ;
#59506=CARTESIAN_POINT('Ctrl Pts',(10.0417974675238,-2.88158937318959,-29.8152005826093)) ;
#59507=CARTESIAN_POINT('Ctrl Pts',(10.0505402348891,-3.01787063559852,-29.8419742868526)) ;
#59508=CARTESIAN_POINT('Ctrl Pts',(10.0549306893133,-3.0862162967159,-29.8553994251151)) ;
#59509=CARTESIAN_POINT('Ctrl Pts',(10.063746247243,-3.22330444799194,-29.8823245653509)) ;
#59510=CARTESIAN_POINT('Ctrl Pts',(10.0681713657794,-3.29204693813702,-29.8958245622563)) ;
#59511=CARTESIAN_POINT('Ctrl Pts',(10.0770536772797,-3.42991551815616,-29.9228974023034)) ;
#59512=CARTESIAN_POINT('Ctrl Pts',(10.0815108721742,-3.49904160803363,-29.9364702447942)) ;
#59513=CARTESIAN_POINT('Ctrl Pts',(10.0949274455347,-3.70697543463906,-29.9772947666975)) ;
#59514=CARTESIAN_POINT('Ctrl Pts',(10.1039317092748,-3.84633872768537,-30.0046524752369)) ;
#59515=CARTESIAN_POINT('Ctrl Pts',(10.122046733416,-4.12644097408161,-30.0596320060214)) ;
#59516=CARTESIAN_POINT('Ctrl Pts',(10.1311575503894,-4.26717992751092,-30.0872538092222)) ;
#59517=CARTESIAN_POINT('Ctrl Pts',(10.1494750088276,-4.54992767466381,-30.1427420485428)) ;
#59518=CARTESIAN_POINT('Ctrl Pts',(10.1586816754589,-4.69193646747835,-30.1706084759848)) ;
#59519=CARTESIAN_POINT('Ctrl Pts',(10.1771814062645,-4.97711807142237,-30.2265660630076)) ;
#59520=CARTESIAN_POINT('Ctrl Pts',(10.186474483048,-5.12029088256691,-30.2546572183432)) ;
#59521=CARTESIAN_POINT('Ctrl Pts',(10.2051383429346,-5.40769470394702,-30.3110441130795)) ;
#59522=CARTESIAN_POINT('Ctrl Pts',(10.214509132221,-5.5519257141803,-30.3393398503962)) ;
#59523=CARTESIAN_POINT('Ctrl Pts',(10.2333201932668,-5.84134011499873,-30.39611560365)) ;
#59524=CARTESIAN_POINT('Ctrl Pts',(10.2427604661428,-5.98652350558523,-30.4245956192103)) ;
#59525=CARTESIAN_POINT('Ctrl Pts',(10.2711736295317,-6.4233435202736,-30.5102814718431)) ;
#59526=CARTESIAN_POINT('Ctrl Pts',(10.2902387921012,-6.71624998261006,-30.5677331383397)) ;
#59527=CARTESIAN_POINT('Ctrl Pts',(10.3285541927133,-7.30460259223824,-30.6831279529963)) ;
#59528=CARTESIAN_POINT('Ctrl Pts',(10.3478044672482,-7.6000487395636,-30.741071088868)) ;
#59529=CARTESIAN_POINT('Ctrl Pts',(10.3864310012383,-8.19263416749283,-30.8572841407583)) ;
#59530=CARTESIAN_POINT('Ctrl Pts',(10.4058072787758,-8.48977344809338,-30.9155540506836)) ;
#59531=CARTESIAN_POINT('Ctrl Pts',(10.4446277699812,-9.08489859170915,-31.0322555983316)) ;
#59532=CARTESIAN_POINT('Ctrl Pts',(10.4640719921157,-9.38288445473128,-31.0906872332025)) ;
#59533=CARTESIAN_POINT('Ctrl Pts',(10.5224204792962,-10.2768420919756,-31.2659768176842)) ;
#59534=CARTESIAN_POINT('Ctrl Pts',(10.5613404148874,-10.8728138989514,-31.3828294944131)) ;
#59535=CARTESIAN_POINT('Ctrl Pts',(10.6387676678931,-12.0579851840454,-31.6151970020299)) ;
#59536=CARTESIAN_POINT('Ctrl Pts',(10.6772750585538,-12.6471846622151,-31.7307118082486)) ;
#59537=CARTESIAN_POINT('Ctrl Pts',(10.7534264185142,-13.8120388658114,-31.959078574304)) ;
#59538=CARTESIAN_POINT('Ctrl Pts',(10.7929238620596,-14.4160365129575,-32.0774868980543)) ;
#59539=CARTESIAN_POINT('Ctrl Pts',(10.8316989411202,-15.0088506101495,-32.1936997662465)) ;
#59540=CARTESIAN_POINT('Ctrl Pts',(10.8335168657289,-15.0366437072151,-32.1991482054207)) ;
#59541=CARTESIAN_POINT('Ctrl Pts',(10.8616065911119,-15.0366437072151,-32.1896836749694)) ;
#59542=CARTESIAN_POINT('Ctrl Pts',(10.8597565733843,-15.0088506101318,-32.1842460492222)) ;
#59543=CARTESIAN_POINT('Ctrl Pts',(10.857904869647,-14.9810324826228,-32.1788035330569)) ;
#59544=CARTESIAN_POINT('Ctrl Pts',(10.8184090484746,-14.3876935911638,-32.0627190668428)) ;
#59545=CARTESIAN_POINT('Ctrl Pts',(10.7800820901594,-13.8120388657218,-31.9500972327959)) ;
#59546=CARTESIAN_POINT('Ctrl Pts',(10.7025039813416,-12.6471846620883,-31.7222111943943)) ;
#59547=CARTESIAN_POINT('Ctrl Pts',(10.6632528658263,-12.0579851838998,-31.6069469782516)) ;
#59548=CARTESIAN_POINT('Ctrl Pts',(10.5842693409797,-10.8728138987679,-31.3751038396628)) ;
#59549=CARTESIAN_POINT('Ctrl Pts',(10.5445370048881,-10.2768420917731,-31.2585248925291)) ;
#59550=CARTESIAN_POINT('Ctrl Pts',(10.4849070942047,-9.38288445450015,-31.08366706989)) ;
#59551=CARTESIAN_POINT('Ctrl Pts',(10.4650251858398,-9.08489859146851,-31.0253829086787)) ;
#59552=CARTESIAN_POINT('Ctrl Pts',(10.4253051421847,-8.48977344783374,-30.9089844555366)) ;
#59553=CARTESIAN_POINT('Ctrl Pts',(10.40546701536,-8.19263416722367,-30.8508701607525)) ;
#59554=CARTESIAN_POINT('Ctrl Pts',(10.3658881887475,-7.60004873927551,-30.7349779736013)) ;
#59555=CARTESIAN_POINT('Ctrl Pts',(10.3461475070413,-7.30460259194072,-30.6772000751425)) ;
#59556=CARTESIAN_POINT('Ctrl Pts',(10.3068161653798,-6.71624998229373,-30.562147570877)) ;
#59557=CARTESIAN_POINT('Ctrl Pts',(10.2872255419149,-6.42334351994791,-30.5048729527681)) ;
#59558=CARTESIAN_POINT('Ctrl Pts',(10.2579901956425,-5.98652350524559,-30.4194641258002)) ;
#59559=CARTESIAN_POINT('Ctrl Pts',(10.2482701603494,-5.84134011465445,-30.3910783731724)) ;
#59560=CARTESIAN_POINT('Ctrl Pts',(10.2288862936885,-5.55192571382677,-30.3344956205997)) ;
#59561=CARTESIAN_POINT('Ctrl Pts',(10.2192224634346,-5.40769470358889,-30.30629862028)) ;
#59562=CARTESIAN_POINT('Ctrl Pts',(10.1999567380997,-5.12029088219959,-30.2501145176226)) ;
#59563=CARTESIAN_POINT('Ctrl Pts',(10.1903548491999,-4.97711807105047,-30.2221274132028)) ;
#59564=CARTESIAN_POINT('Ctrl Pts',(10.1712182678004,-4.69193646709734,-30.1663844061269)) ;
#59565=CARTESIAN_POINT('Ctrl Pts',(10.1616835879102,-4.54992767427827,-30.138628499219)) ;
#59566=CARTESIAN_POINT('Ctrl Pts',(10.1426859378703,-4.26717992711634,-30.0833694431312)) ;
#59567=CARTESIAN_POINT('Ctrl Pts',(10.1332229930092,-4.12644097368253,-30.0558662856289)) ;
#59568=CARTESIAN_POINT('Ctrl Pts',(10.1143720437184,-3.84633872727734,-30.0011347168959)) ;
#59569=CARTESIAN_POINT('Ctrl Pts',(10.104984095847,-3.70697543422659,-29.9739062865914)) ;
#59570=CARTESIAN_POINT('Ctrl Pts',(10.0909589888611,-3.49904160761451,-29.9332868035381)) ;
#59571=CARTESIAN_POINT('Ctrl Pts',(10.0862933965109,-3.42991551773483,-29.9197841783251)) ;
#59572=CARTESIAN_POINT('Ctrl Pts',(10.0769807583747,-3.2920469377113,-29.8928563322026)) ;
#59573=CARTESIAN_POINT('Ctrl Pts',(10.0723337145218,-3.22330444756401,-29.879431110642)) ;
#59574=CARTESIAN_POINT('Ctrl Pts',(10.0630573184486,-3.08621629628361,-29.8526612448547)) ;
#59575=CARTESIAN_POINT('Ctrl Pts',(10.0584279812629,-3.01787063516402,-29.8393165955654)) ;
#59576=CARTESIAN_POINT('Ctrl Pts',(10.0491852822835,-2.88158937275076,-29.8127113378945)) ;
#59577=CARTESIAN_POINT('Ctrl Pts',(10.0445719575502,-2.81365377138444,-29.7994507170098)) ;
#59578=CARTESIAN_POINT('Ctrl Pts',(10.0357586992447,-2.68409673802282,-29.7741671476752)) ;
#59579=CARTESIAN_POINT('Ctrl Pts',(10.0313354854857,-2.61917207517383,-29.7614990802411)) ;
#59580=CARTESIAN_POINT('Ctrl Pts',(10.0245251307954,-2.51946652197692,-29.7420505045245)) ;
#59581=CARTESIAN_POINT('Ctrl Pts',(10.0222257294742,-2.48584491117954,-29.7354932427815)) ;
#59582=CARTESIAN_POINT('Ctrl Pts',(10.0175927471364,-2.41821530769531,-29.7223059756892)) ;
#59583=CARTESIAN_POINT('Ctrl Pts',(10.01525918304,-2.38420731496295,-29.7156759646289)) ;
#59584=CARTESIAN_POINT('Ctrl Pts',(10.0105814814048,-2.31619142061517,-29.7024195249859)) ;
#59585=CARTESIAN_POINT('Ctrl Pts',(10.0082373866956,-2.28218353266388,-29.6957930849522)) ;
#59586=CARTESIAN_POINT('Ctrl Pts',(10.0047297976448,-2.2314616292666,-29.6859137691122)) ;
#59587=CARTESIAN_POINT('Ctrl Pts',(10.0035620095976,-2.21460264962826,-29.6826307270115)) ;
#59588=CARTESIAN_POINT('Ctrl Pts',(10.0012316710292,-2.18102964096591,-29.6760944881331)) ;
#59589=CARTESIAN_POINT('Ctrl Pts',(10.0000691226531,-2.16431561193394,-29.6728412906312)) ;
#59590=CARTESIAN_POINT('Ctrl Pts',(9.99775126861663,-2.13108081363099,-29.6663746003226)) ;
#59591=CARTESIAN_POINT('Ctrl Pts',(9.99659597999818,-2.11456004819905,-29.6631611026111)) ;
#59592=CARTESIAN_POINT('Ctrl Pts',(9.99429387456847,-2.0817600899311,-29.6567839335578)) ;
#59593=CARTESIAN_POINT('Ctrl Pts',(9.99314710341809,-2.06548089689024,-29.6536202467865)) ;
#59594=CARTESIAN_POINT('Ctrl Pts',(9.99143297536932,-2.04127952112266,-29.6489200977634)) ;
#59595=CARTESIAN_POINT('Ctrl Pts',(9.99086258006168,-2.03324863236408,-29.6473609532442)) ;
#59596=CARTESIAN_POINT('Ctrl Pts',(9.98972334381673,-2.01726536736095,-29.6442592620639)) ;
#59597=CARTESIAN_POINT('Ctrl Pts',(9.98915450367532,-2.0093129911118,-29.6427167151343)) ;
#59598=CARTESIAN_POINT('Ctrl Pts',(9.98801744725042,-1.99349279360512,-29.6396498503709)) ;
#59599=CARTESIAN_POINT('Ctrl Pts',(9.98744925815376,-1.98562497252213,-29.638125523415)) ;
#59600=CARTESIAN_POINT('Ctrl Pts',(9.98659595732529,-1.97389119369923,-29.6358541944921)) ;
#59601=CARTESIAN_POINT('Ctrl Pts',(9.98631134296961,-1.96999125966218,-29.6350996155713)) ;
#59602=CARTESIAN_POINT('Ctrl Pts',(9.98574128636084,-1.96221480021287,-29.6335958415077)) ;
#59603=CARTESIAN_POINT('Ctrl Pts',(9.98545584580647,-1.95833827478728,-29.6328466457898)) ;
#59604=CARTESIAN_POINT('Ctrl Pts',(9.98488301744925,-1.95060454321582,-29.6313531235031)) ;
#59605=CARTESIAN_POINT('Ctrl Pts',(9.98458042814821,-1.94654185495839,-29.6305691084804)) ;
#59606=CARTESIAN_POINT('Ctrl Pts',(9.98395498092834,-1.93822324700642,-29.6289657688539)) ;
#59607=CARTESIAN_POINT('Ctrl Pts',(9.98363219212854,-1.9339673266325,-29.628146420813)) ;
#59608=CARTESIAN_POINT('Ctrl Pts',(9.98314025611079,-1.9275837089799,-29.6269200683138)) ;
#59609=CARTESIAN_POINT('Ctrl Pts',(9.98297497049299,-1.92545589351462,-29.6265117369574)) ;
#59610=CARTESIAN_POINT('Ctrl Pts',(9.98264248827336,-1.9212245567182,-29.6257010160644)) ;
#59611=CARTESIAN_POINT('Ctrl Pts',(9.9824753255637,-1.91912103493106,-29.6252986150088)) ;
#59612=CARTESIAN_POINT('Ctrl Pts',(9.98222295889623,-1.91600211746307,-29.6247034904741)) ;
#59613=CARTESIAN_POINT('Ctrl Pts',(9.98213855545869,-1.91496854298954,-29.624506532935)) ;
#59614=CARTESIAN_POINT('Ctrl Pts',(9.98196891063809,-1.91291654451728,-29.6241162041275)) ;
#59615=CARTESIAN_POINT('Ctrl Pts',(9.98188367167153,-1.91189812047543,-29.6239228320356)) ;
#59616=CARTESIAN_POINT('Ctrl Pts',(9.98171166896053,-1.90987945131465,-29.6235405659712)) ;
#59617=CARTESIAN_POINT('Ctrl Pts',(9.98162494256724,-1.90887920802121,-29.6233516598116)) ;
#59618=CARTESIAN_POINT('Ctrl Pts',(9.98149237338653,-1.90739476260648,-29.6230726076883)) ;
#59619=CARTESIAN_POINT('Ctrl Pts',(9.9814477610636,-1.90690260122667,-29.6229803114205)) ;
#59620=CARTESIAN_POINT('Ctrl Pts',(9.98135713865687,-1.90592397334478,-29.6227974317535)) ;
#59621=CARTESIAN_POINT('Ctrl Pts',(9.98131115132827,-1.90543750619486,-29.6227068405461)) ;
#59622=CARTESIAN_POINT('Ctrl Pts',(9.98123957118407,-1.90470544341716,-29.6225713143871)) ;
#59623=CARTESIAN_POINT('Ctrl Pts',(9.98121362489977,-1.90444442240732,-29.6225231346487)) ;
#59624=CARTESIAN_POINT('Ctrl Pts',(9.98115905365425,-1.90391015241643,-29.6224250111128)) ;
#59625=CARTESIAN_POINT('Ctrl Pts',(9.981130433504,-1.90363690324913,-29.6223750656538)) ;
#59626=CARTESIAN_POINT('Ctrl Pts',(9.98107064682837,-1.90309071780404,-29.6222761009427)) ;
#59627=CARTESIAN_POINT('Ctrl Pts',(9.9810395738566,-1.90281782033889,-29.6222270586329)) ;
#59628=CARTESIAN_POINT('Ctrl Pts',(9.98083763067218,-1.90163369767085,-29.6220368741041)) ;
#59629=CARTESIAN_POINT('Ctrl Pts',(9.98082932832723,-1.9015850156869,-29.6220290551843)) ;
#59630=CARTESIAN_POINT('Ctrl Pts',(9.98082102598227,-1.90153633370295,-29.6220212362645)) ;
#59631=CARTESIAN_POINT('',(23.3523050271291,-15.0366437072153,-24.6742797818822)) ;
#59632=CARTESIAN_POINT('',(23.3738245177983,-15.0366437072153,-24.6538954375541)) ;
#59633=CARTESIAN_POINT('Origin',(-0.939357956114975,-21.6462763158693,0.991668137384664)) ;
#59634=CARTESIAN_POINT('',(21.496311701647,-1.90153623936716,-22.6933803669979)) ;
#59635=CARTESIAN_POINT('Ctrl Pts',(21.4963117139471,-1.90153632716387,-22.6933803803385)) ;
#59636=CARTESIAN_POINT('Ctrl Pts',(21.4963139585538,-1.90158488788986,-22.6933920772455)) ;
#59637=CARTESIAN_POINT('Ctrl Pts',(21.4963526813015,-1.90242263142415,-22.6935938659951)) ;
#59638=CARTESIAN_POINT('Ctrl Pts',(21.4963918791992,-1.90282441372072,-22.6936711055929)) ;
#59639=CARTESIAN_POINT('Ctrl Pts',(21.4964208293853,-1.90309873132532,-22.6937217687247)) ;
#59640=CARTESIAN_POINT('Ctrl Pts',(21.4964806174594,-1.9036477572329,-22.693821418077)) ;
#59641=CARTESIAN_POINT('Ctrl Pts',(21.4965115196631,-1.90392242669208,-22.6938703323172)) ;
#59642=CARTESIAN_POINT('Ctrl Pts',(21.4965730073544,-1.90445947279204,-22.6939649615802)) ;
#59643=CARTESIAN_POINT('Ctrl Pts',(21.4966035966074,-1.90472184962075,-22.6940106730897)) ;
#59644=CARTESIAN_POINT('Ctrl Pts',(21.4966903054876,-1.90545775387604,-22.6941380177788)) ;
#59645=CARTESIAN_POINT('Ctrl Pts',(21.4967491393391,-1.90594678716221,-22.6942214937476)) ;
#59646=CARTESIAN_POINT('Ctrl Pts',(21.4968689478468,-1.90693057720395,-22.6943880470282)) ;
#59647=CARTESIAN_POINT('Ctrl Pts',(21.4969299401569,-1.90742533460924,-22.6944711078024)) ;
#59648=CARTESIAN_POINT('Ctrl Pts',(21.4971154317997,-1.90891760993743,-22.6947201861981)) ;
#59649=CARTESIAN_POINT('Ctrl Pts',(21.4972424168975,-1.90992312895963,-22.6948861267403)) ;
#59650=CARTESIAN_POINT('Ctrl Pts',(21.4975010204046,-1.91195244521774,-22.6952188219258)) ;
#59651=CARTESIAN_POINT('Ctrl Pts',(21.4976326671314,-1.91297624062658,-22.6953855492251)) ;
#59652=CARTESIAN_POINT('Ctrl Pts',(21.4978995329129,-1.91503906152865,-22.695719955273)) ;
#59653=CARTESIAN_POINT('Ctrl Pts',(21.4980347538706,-1.91607808706589,-22.6958876322313)) ;
#59654=CARTESIAN_POINT('Ctrl Pts',(21.4984445862641,-1.91921345336299,-22.696391919799)) ;
#59655=CARTESIAN_POINT('Ctrl Pts',(21.4987233311854,-1.92132806855155,-22.6967298168923)) ;
#59656=CARTESIAN_POINT('Ctrl Pts',(21.4992869388782,-1.92558171967302,-22.6974067674593)) ;
#59657=CARTESIAN_POINT('Ctrl Pts',(21.4995718277727,-1.927720756062,-22.6977457963179)) ;
#59658=CARTESIAN_POINT('Ctrl Pts',(21.500429539133,-1.93413803650467,-22.6987600475774)) ;
#59659=CARTESIAN_POINT('Ctrl Pts',(21.5010053506063,-1.93841639875659,-22.6994324722858)) ;
#59660=CARTESIAN_POINT('Ctrl Pts',(21.5021350348965,-1.94677887040481,-22.7007428078236)) ;
#59661=CARTESIAN_POINT('Ctrl Pts',(21.502688960902,-1.95086298048004,-22.7013806684633)) ;
#59662=CARTESIAN_POINT('Ctrl Pts',(21.5037458825198,-1.95863767629825,-22.7025926144358)) ;
#59663=CARTESIAN_POINT('Ctrl Pts',(21.5042769737302,-1.96253482848826,-22.7031988866226)) ;
#59664=CARTESIAN_POINT('Ctrl Pts',(21.505344320571,-1.97035266596653,-22.70441323784)) ;
#59665=CARTESIAN_POINT('Ctrl Pts',(21.5058805775187,-1.9742733512682,-22.7050213156265)) ;
#59666=CARTESIAN_POINT('Ctrl Pts',(21.5074963416005,-1.98606956461108,-22.7068486477647)) ;
#59667=CARTESIAN_POINT('Ctrl Pts',(21.5085828074178,-1.99397924967536,-22.7080710335096)) ;
#59668=CARTESIAN_POINT('Ctrl Pts',(21.5107715848834,-2.00988362495031,-22.7105249922724)) ;
#59669=CARTESIAN_POINT('Ctrl Pts',(21.5118739173825,-2.01787831498638,-22.7117565454895)) ;
#59670=CARTESIAN_POINT('Ctrl Pts',(21.5140925843333,-2.03394662524021,-22.7142288565352)) ;
#59671=CARTESIAN_POINT('Ctrl Pts',(21.5152089193814,-2.04202024546243,-22.7154696137994)) ;
#59672=CARTESIAN_POINT('Ctrl Pts',(21.5185767066728,-2.06635039394262,-22.7192052036515)) ;
#59673=CARTESIAN_POINT('Ctrl Pts',(21.5208468664255,-2.08271620655358,-22.7217134240119)) ;
#59674=CARTESIAN_POINT('Ctrl Pts',(21.5254273675335,-2.11569068912034,-22.7267609335447)) ;
#59675=CARTESIAN_POINT('Ctrl Pts',(21.5277377440152,-2.13229935928107,-22.7293001895015)) ;
#59676=CARTESIAN_POINT('Ctrl Pts',(21.5323903166247,-2.16571099516926,-22.7344038676818)) ;
#59677=CARTESIAN_POINT('Ctrl Pts',(21.5347325251025,-2.18251395705726,-22.7369682771135)) ;
#59678=CARTESIAN_POINT('Ctrl Pts',(21.5394409725641,-2.21626560252734,-22.7421158136557)) ;
#59679=CARTESIAN_POINT('Ctrl Pts',(21.5418072131894,-2.23321428611731,-22.7446989392129)) ;
#59680=CARTESIAN_POINT('Ctrl Pts',(21.5489307493174,-2.28420607246569,-22.7524662951117)) ;
#59681=CARTESIAN_POINT('Ctrl Pts',(21.553712806182,-2.31839491051271,-22.7576685546976)) ;
#59682=CARTESIAN_POINT('Ctrl Pts',(21.5632849986474,-2.38677270505818,-22.7680654550021)) ;
#59683=CARTESIAN_POINT('Ctrl Pts',(21.5680751645116,-2.4209616478915,-22.7732600631636)) ;
#59684=CARTESIAN_POINT('Ctrl Pts',(21.5776069357775,-2.48895109533015,-22.7835847070533)) ;
#59685=CARTESIAN_POINT('Ctrl Pts',(21.5823485541794,-2.52275159998098,-22.7887147304799)) ;
#59686=CARTESIAN_POINT('Ctrl Pts',(21.5964164967376,-2.6229876659894,-22.8039216843402)) ;
#59687=CARTESIAN_POINT('Ctrl Pts',(21.6055858239275,-2.68825777904764,-22.8138155781247)) ;
#59688=CARTESIAN_POINT('Ctrl Pts',(21.6238983410685,-2.81853945525282,-22.8335545263681)) ;
#59689=CARTESIAN_POINT('Ctrl Pts',(21.6335094237685,-2.88687193565162,-22.843901688933)) ;
#59690=CARTESIAN_POINT('Ctrl Pts',(21.6527986704329,-3.02394935163266,-22.8646498792361)) ;
#59691=CARTESIAN_POINT('Ctrl Pts',(21.6624768629465,-3.09269428728769,-22.8750508799517)) ;
#59692=CARTESIAN_POINT('Ctrl Pts',(21.681896480493,-3.23058330586397,-22.8959066041)) ;
#59693=CARTESIAN_POINT('Ctrl Pts',(21.6916379170892,-3.29972738877161,-22.9063613165752)) ;
#59694=CARTESIAN_POINT('Ctrl Pts',(21.7111808231678,-3.43840139526491,-22.9273237072948)) ;
#59695=CARTESIAN_POINT('Ctrl Pts',(21.7209822941359,-3.50793131885397,-22.9378313841313)) ;
#59696=CARTESIAN_POINT('Ctrl Pts',(21.7504725253938,-3.71707989210545,-22.9694321897675)) ;
#59697=CARTESIAN_POINT('Ctrl Pts',(21.7702470244795,-3.85725734359656,-22.9906031688657)) ;
#59698=CARTESIAN_POINT('Ctrl Pts',(21.8100047544406,-4.13899594338214,-23.0331412836721)) ;
#59699=CARTESIAN_POINT('Ctrl Pts',(21.8299880288275,-4.2805570917561,-23.0545083781865)) ;
#59700=CARTESIAN_POINT('Ctrl Pts',(21.870145346404,-4.56495664710652,-23.0974254409772)) ;
#59701=CARTESIAN_POINT('Ctrl Pts',(21.890319408865,-4.70779505317279,-23.1189753907396)) ;
#59702=CARTESIAN_POINT('Ctrl Pts',(21.9308412967585,-4.99464268373381,-23.1622439739505)) ;
#59703=CARTESIAN_POINT('Ctrl Pts',(21.9511891318898,-5.13865190824363,-23.1839625982162)) ;
#59704=CARTESIAN_POINT('Ctrl Pts',(21.992042125138,-5.42773473827606,-23.2275538051461)) ;
#59705=CARTESIAN_POINT('Ctrl Pts',(22.0125472880069,-5.57280834379641,-23.2494263833081)) ;
#59706=CARTESIAN_POINT('Ctrl Pts',(22.0536988560531,-5.8639134989194,-23.2933104325269)) ;
#59707=CARTESIAN_POINT('Ctrl Pts',(22.0743452620874,-6.00994504852342,-23.3153219027712)) ;
#59708=CARTESIAN_POINT('Ctrl Pts',(22.1364725738118,-6.44931695857324,-23.3815417220833)) ;
#59709=CARTESIAN_POINT('Ctrl Pts',(22.1781415168096,-6.74393457555848,-23.4259355317348)) ;
#59710=CARTESIAN_POINT('Ctrl Pts',(22.2618558852985,-7.33572433109793,-23.5150936882605)) ;
#59711=CARTESIAN_POINT('Ctrl Pts',(22.303901338843,-7.63289646968583,-23.5598580085705)) ;
#59712=CARTESIAN_POINT('Ctrl Pts',(22.388245232698,-8.22894377121979,-23.6496317838259)) ;
#59713=CARTESIAN_POINT('Ctrl Pts',(22.4305436869088,-8.52781893416259,-23.6946412256033)) ;
#59714=CARTESIAN_POINT('Ctrl Pts',(22.5152708871044,-9.12642078800902,-23.784779082941)) ;
#59715=CARTESIAN_POINT('Ctrl Pts',(22.5576996395945,-9.42614747891959,-23.8299074923405)) ;
#59716=CARTESIAN_POINT('Ctrl Pts',(22.6849980529511,-10.3253275998488,-23.9652812195954)) ;
#59717=CARTESIAN_POINT('Ctrl Pts',(22.7698797528227,-10.9247810626322,-24.0555151428219)) ;
#59718=CARTESIAN_POINT('Ctrl Pts',(22.9387013685547,-12.1168760951015,-24.2349360469274)) ;
#59719=CARTESIAN_POINT('Ctrl Pts',(23.0226413407052,-12.7095176648389,-24.3241229744988)) ;
#59720=CARTESIAN_POINT('Ctrl Pts',(23.1889804045827,-13.8838032555933,-24.5008259087648)) ;
#59721=CARTESIAN_POINT('Ctrl Pts',(23.2713709284772,-14.465386062484,-24.5883326063611)) ;
#59722=CARTESIAN_POINT('Ctrl Pts',(23.3523050271262,-15.0366437072153,-24.6742797818849)) ;
#59723=CARTESIAN_POINT('Ctrl Pts',(23.3738245178012,-15.0366437072153,-24.6538954375513)) ;
#59724=CARTESIAN_POINT('Ctrl Pts',(23.3734610461599,-15.0340941323794,-24.6535139839134)) ;
#59725=CARTESIAN_POINT('Ctrl Pts',(23.37309754507,-15.0315443518747,-24.6531324996256)) ;
#59726=CARTESIAN_POINT('Ctrl Pts',(23.2916449156809,-14.4601946117196,-24.5676502869763)) ;
#59727=CARTESIAN_POINT('Ctrl Pts',(23.2090927645543,-13.8811769232892,-24.4810268676804)) ;
#59728=CARTESIAN_POINT('Ctrl Pts',(23.0420288777678,-12.7095176651673,-24.3057581239909)) ;
#59729=CARTESIAN_POINT('Ctrl Pts',(22.957517168995,-12.1168760954787,-24.2171127741293)) ;
#59730=CARTESIAN_POINT('Ctrl Pts',(22.7874992191376,-10.9247810631074,-24.0388250979295)) ;
#59731=CARTESIAN_POINT('Ctrl Pts',(22.7019930343313,-10.3253276003733,-23.9491827182685)) ;
#59732=CARTESIAN_POINT('Ctrl Pts',(22.5737096414841,-9.4261474795181,-23.814742013168)) ;
#59733=CARTESIAN_POINT('Ctrl Pts',(22.5309444631412,-9.12642078863219,-23.7699322832708)) ;
#59734=CARTESIAN_POINT('Ctrl Pts',(22.4455258388896,-8.52781893483503,-23.6804493776025)) ;
#59735=CARTESIAN_POINT('Ctrl Pts',(22.4028723994856,-8.2289437719168,-23.6357761956683)) ;
#59736=CARTESIAN_POINT('Ctrl Pts',(22.3177965715717,-7.63289647043186,-23.5466957451952)) ;
#59737=CARTESIAN_POINT('Ctrl Pts',(22.2753741969594,-7.33572433186842,-23.5022884634925)) ;
#59738=CARTESIAN_POINT('Ctrl Pts',(22.1908790031011,-6.74393457637766,-23.4138699440584)) ;
#59739=CARTESIAN_POINT('Ctrl Pts',(22.1488062118971,-6.44931695941667,-23.3698586797545)) ;
#59740=CARTESIAN_POINT('Ctrl Pts',(22.0860470145102,-6.00994504940297,-23.3042374143459)) ;
#59741=CARTESIAN_POINT('Ctrl Pts',(22.0651855998762,-5.86391349981098,-23.282429611069)) ;
#59742=CARTESIAN_POINT('Ctrl Pts',(22.0235938113801,-5.57280834471192,-23.2389625608171)) ;
#59743=CARTESIAN_POINT('Ctrl Pts',(22.0028634383754,-5.42773473920353,-23.2173033130307)) ;
#59744=CARTESIAN_POINT('Ctrl Pts',(21.9615478981759,-5.13865190919487,-23.1741502538532)) ;
#59745=CARTESIAN_POINT('Ctrl Pts',(21.9409627357323,-4.9946426846969,-23.1526564379623)) ;
#59746=CARTESIAN_POINT('Ctrl Pts',(21.899951420414,-4.70779505415949,-23.1098514650408)) ;
#59747=CARTESIAN_POINT('Ctrl Pts',(21.8795252772345,-4.56495664810496,-23.0885402988219)) ;
#59748=CARTESIAN_POINT('Ctrl Pts',(21.8388452293624,-4.28055709277793,-23.0461183924753)) ;
#59749=CARTESIAN_POINT('Ctrl Pts',(21.8185913441993,-4.13899594441561,-23.0250076341073)) ;
#59750=CARTESIAN_POINT('Ctrl Pts',(21.7782680553142,-3.85725734465321,-22.9830052451768)) ;
#59751=CARTESIAN_POINT('Ctrl Pts',(21.7581986950839,-3.71707989317363,-22.9621135733942)) ;
#59752=CARTESIAN_POINT('Ctrl Pts',(21.7282408036885,-3.50793131993937,-22.9309557589758)) ;
#59753=CARTESIAN_POINT('Ctrl Pts',(21.7182791782025,-3.43840139635602,-22.9205997885584)) ;
#59754=CARTESIAN_POINT('Ctrl Pts',(21.6984055622423,-3.29972738987415,-22.8999506628818)) ;
#59755=CARTESIAN_POINT('Ctrl Pts',(21.6884935732522,-3.23058330697217,-22.8896575062172)) ;
#59756=CARTESIAN_POINT('Ctrl Pts',(21.6687197927208,-3.09269428840723,-22.8691372630713)) ;
#59757=CARTESIAN_POINT('Ctrl Pts',(21.6588580127507,-3.02394935275785,-22.8589101656336)) ;
#59758=CARTESIAN_POINT('Ctrl Pts',(21.6391845502197,-2.88687193678811,-22.8385259239346)) ;
#59759=CARTESIAN_POINT('Ctrl Pts',(21.6293728961843,-2.81853945639494,-22.828368752632)) ;
#59760=CARTESIAN_POINT('Ctrl Pts',(21.6106543164916,-2.68825778012938,-22.8090144472516)) ;
#59761=CARTESIAN_POINT('Ctrl Pts',(21.6012713503163,-2.62298766700186,-22.7993229230439)) ;
#59762=CARTESIAN_POINT('Ctrl Pts',(21.5868483218045,-2.52275160088707,-22.7844523244347)) ;
#59763=CARTESIAN_POINT('Ctrl Pts',(21.5819825280398,-2.48895109620037,-22.7794399261495)) ;
#59764=CARTESIAN_POINT('Ctrl Pts',(21.5721890658123,-2.42096164868958,-22.7693631690854)) ;
#59765=CARTESIAN_POINT('Ctrl Pts',(21.5672614103372,-2.38677270581997,-22.7642987979908)) ;
#59766=CARTESIAN_POINT('Ctrl Pts',(21.5573979860251,-2.31839491120195,-22.7541777671244)) ;
#59767=CARTESIAN_POINT('Ctrl Pts',(21.5524622513411,-2.28420607311861,-22.749121078891)) ;
#59768=CARTESIAN_POINT('Ctrl Pts',(21.5450919474027,-2.23321428671612,-22.7415874738631)) ;
#59769=CARTESIAN_POINT('Ctrl Pts',(21.5426407158965,-2.2162656031082,-22.7390848559396)) ;
#59770=CARTESIAN_POINT('Ctrl Pts',(21.5377556388623,-2.18251395760228,-22.7341046318056)) ;
#59771=CARTESIAN_POINT('Ctrl Pts',(21.5353217949764,-2.16571099569641,-22.731627024038)) ;
#59772=CARTESIAN_POINT('Ctrl Pts',(21.5304774869785,-2.13229935977276,-22.7267049672548)) ;
#59773=CARTESIAN_POINT('Ctrl Pts',(21.5280670363083,-2.11569068959445,-22.7242605065996)) ;
#59774=CARTESIAN_POINT('Ctrl Pts',(21.5232749127087,-2.0827162069927,-22.7194134565288)) ;
#59775=CARTESIAN_POINT('Ctrl Pts',(21.520893274851,-2.06635039436428,-22.7170108338336)) ;
#59776=CARTESIAN_POINT('Ctrl Pts',(21.5173454918877,-2.04202024585826,-22.7134457449312)) ;
#59777=CARTESIAN_POINT('Ctrl Pts',(21.516166991437,-2.03394662562764,-22.7122638738618)) ;
#59778=CARTESIAN_POINT('Ctrl Pts',(21.5138184224543,-2.01787831535676,-22.7099146125519)) ;
#59779=CARTESIAN_POINT('Ctrl Pts',(21.5126483545181,-2.00988362531201,-22.7087472217466)) ;
#59780=CARTESIAN_POINT('Ctrl Pts',(21.5103164927178,-1.99397925002019,-22.7064287996602)) ;
#59781=CARTESIAN_POINT('Ctrl Pts',(21.5091547197619,-1.98606956494765,-22.7052777486237)) ;
#59782=CARTESIAN_POINT('Ctrl Pts',(21.5074175432658,-1.97427335159223,-22.7035654244297)) ;
#59783=CARTESIAN_POINT('Ctrl Pts',(21.5068393896569,-1.97035266628625,-22.7029970332676)) ;
#59784=CARTESIAN_POINT('Ctrl Pts',(21.505684604382,-1.96253482879969,-22.701865508132)) ;
#59785=CARTESIAN_POINT('Ctrl Pts',(21.5051079740316,-1.95863767660568,-22.7013023729089)) ;
#59786=CARTESIAN_POINT('Ctrl Pts',(21.5039550260575,-1.95086298073556,-22.7001813879179)) ;
#59787=CARTESIAN_POINT('Ctrl Pts',(21.5033480898594,-1.94677887060986,-22.6995937411855)) ;
#59788=CARTESIAN_POINT('Ctrl Pts',(21.5021008358999,-1.93841639885889,-22.6983947735248)) ;
#59789=CARTESIAN_POINT('Ctrl Pts',(21.5014605711589,-1.93413803655436,-22.6977834021797)) ;
#59790=CARTESIAN_POINT('Ctrl Pts',(21.500494242935,-1.92772075603282,-22.696872038256)) ;
#59791=CARTESIAN_POINT('Ctrl Pts',(21.500171134863,-1.92558171961753,-22.6965692125178)) ;
#59792=CARTESIAN_POINT('Ctrl Pts',(21.4995256901997,-1.92132806844377,-22.695969782032)) ;
#59793=CARTESIAN_POINT('Ctrl Pts',(21.4992033795886,-1.91921345322948,-22.695673152545)) ;
#59794=CARTESIAN_POINT('Ctrl Pts',(21.4987220194729,-1.91607808689387,-22.6952366196236)) ;
#59795=CARTESIAN_POINT('Ctrl Pts',(21.4985619091592,-1.91503906134344,-22.6950925191119)) ;
#59796=CARTESIAN_POINT('Ctrl Pts',(21.4982424413642,-1.91297624041611,-22.6948079403308)) ;
#59797=CARTESIAN_POINT('Ctrl Pts',(21.4980830857427,-1.91195244499585,-22.6946674602874)) ;
#59798=CARTESIAN_POINT('Ctrl Pts',(21.4977648789956,-1.90992312871267,-22.6943912242827)) ;
#59799=CARTESIAN_POINT('Ctrl Pts',(21.4976060566755,-1.90891760967738,-22.6942554415556)) ;
#59800=CARTESIAN_POINT('Ctrl Pts',(21.4973673858906,-1.90742533433075,-22.6940567371139)) ;
#59801=CARTESIAN_POINT('Ctrl Pts',(21.497287749008,-1.90693057691868,-22.6939913374149)) ;
#59802=CARTESIAN_POINT('Ctrl Pts',(21.4971279262894,-1.90594678686493,-22.6938626876047)) ;
#59803=CARTESIAN_POINT('Ctrl Pts',(21.4970477579221,-1.90545775357358,-22.6937994207613)) ;
#59804=CARTESIAN_POINT('Ctrl Pts',(21.4969252943185,-1.90472184931356,-22.6937059447438)) ;
#59805=CARTESIAN_POINT('Ctrl Pts',(21.4968813058637,-1.9044594724889,-22.6936729256337)) ;
#59806=CARTESIAN_POINT('Ctrl Pts',(21.4967901442597,-1.90392242639159,-22.6936064049946)) ;
#59807=CARTESIAN_POINT('Ctrl Pts',(21.4967429748205,-1.90364775693111,-22.693572899898)) ;
#59808=CARTESIAN_POINT('Ctrl Pts',(21.4966467084668,-1.90309873102656,-22.6935078046084)) ;
#59809=CARTESIAN_POINT('Ctrl Pts',(21.4965976870603,-1.90282441341568,-22.6934761539446)) ;
#59810=CARTESIAN_POINT('Ctrl Pts',(21.4963333307451,-1.90163369401068,-22.6933876198957)) ;
#59811=CARTESIAN_POINT('Ctrl Pts',(21.4963225223461,-1.90158501058727,-22.6933840001171)) ;
#59812=CARTESIAN_POINT('Ctrl Pts',(21.4963117139471,-1.90153632716387,-22.6933803803385)) ;
#59813=CARTESIAN_POINT('',(31.5544392045414,-15.0366437072153,-12.5883914509194)) ;
#59814=CARTESIAN_POINT('',(31.565410601292,-15.0366437072153,-12.5608553214549)) ;
#59815=CARTESIAN_POINT('Origin',(-1.2689288344947,-21.6462763158693,0.505587457724587)) ;
#59816=CARTESIAN_POINT('',(29.0382272079201,-1.90153624090668,-11.5698872032838)) ;
#59817=CARTESIAN_POINT('Ctrl Pts',(29.0382272249795,-1.90153633024293,-11.569887210347)) ;
#59818=CARTESIAN_POINT('Ctrl Pts',(29.0382341685625,-1.90158488937111,-11.5698968952696)) ;
#59819=CARTESIAN_POINT('Ctrl Pts',(29.0383534545912,-1.90241910213499,-11.5700632756462)) ;
#59820=CARTESIAN_POINT('Ctrl Pts',(29.0384211680538,-1.9028192570987,-11.5701167460572)) ;
#59821=CARTESIAN_POINT('Ctrl Pts',(29.0384685127817,-1.90309246453481,-11.5701504595666)) ;
#59822=CARTESIAN_POINT('Ctrl Pts',(29.0385642093004,-1.90363926995708,-11.5702155771039)) ;
#59823=CARTESIAN_POINT('Ctrl Pts',(29.0386125891881,-1.90391282912392,-11.5702468889399)) ;
#59824=CARTESIAN_POINT('Ctrl Pts',(29.0387077264248,-1.90444770504447,-11.5703067495747)) ;
#59825=CARTESIAN_POINT('Ctrl Pts',(29.0387544856515,-1.90470902198025,-11.5703352937625)) ;
#59826=CARTESIAN_POINT('Ctrl Pts',(29.038886093546,-1.90544192358575,-11.5704141835626)) ;
#59827=CARTESIAN_POINT('Ctrl Pts',(29.0389741666542,-1.90592895120476,-11.5704650586967)) ;
#59828=CARTESIAN_POINT('Ctrl Pts',(29.0391520824275,-1.9069087065474,-11.5705655502498)) ;
#59829=CARTESIAN_POINT('Ctrl Pts',(29.039241934173,-1.90740143492223,-11.5706151442418)) ;
#59830=CARTESIAN_POINT('Ctrl Pts',(29.0395137203389,-1.90888759045901,-11.5707627771257)) ;
#59831=CARTESIAN_POINT('Ctrl Pts',(29.0396978706761,-1.90988898601723,-11.5708597034774)) ;
#59832=CARTESIAN_POINT('Ctrl Pts',(29.0400707017281,-1.91190998059807,-11.5710523493246)) ;
#59833=CARTESIAN_POINT('Ctrl Pts',(29.0402593966093,-1.91292957779318,-11.5711480322448)) ;
#59834=CARTESIAN_POINT('Ctrl Pts',(29.0406404146295,-1.91498393997969,-11.5713387604754)) ;
#59835=CARTESIAN_POINT('Ctrl Pts',(29.0408327387316,-1.91601870501465,-11.571433803393)) ;
#59836=CARTESIAN_POINT('Ctrl Pts',(29.0414140068024,-1.9191412150523,-11.571718320527)) ;
#59837=CARTESIAN_POINT('Ctrl Pts',(29.0418072264422,-1.92124715973623,-11.57190722504)) ;
#59838=CARTESIAN_POINT('Ctrl Pts',(29.0425996817526,-1.92548337017848,-11.5722835141449)) ;
#59839=CARTESIAN_POINT('Ctrl Pts',(29.0429989307614,-1.92761363639261,-11.5724708655146)) ;
#59840=CARTESIAN_POINT('Ctrl Pts',(29.044198247386,-1.93400460629616,-11.5730290758498)) ;
#59841=CARTESIAN_POINT('Ctrl Pts',(29.0449998498987,-1.93826542817482,-11.5733961485032)) ;
#59842=CARTESIAN_POINT('Ctrl Pts',(29.0465687990394,-1.94659361634588,-11.5741082576043)) ;
#59843=CARTESIAN_POINT('Ctrl Pts',(29.0473361728228,-1.95066098331758,-11.5744532262768)) ;
#59844=CARTESIAN_POINT('Ctrl Pts',(29.0487981958263,-1.95840366162645,-11.5751067922209)) ;
#59845=CARTESIAN_POINT('Ctrl Pts',(29.0495316973985,-1.96228469190273,-11.575432736428)) ;
#59846=CARTESIAN_POINT('Ctrl Pts',(29.0510041256863,-1.97007018824413,-11.5760840936556)) ;
#59847=CARTESIAN_POINT('Ctrl Pts',(29.0517430530695,-1.9739746543226,-11.5764095050075)) ;
#59848=CARTESIAN_POINT('Ctrl Pts',(29.0539674538176,-1.98572206873987,-11.577385610067)) ;
#59849=CARTESIAN_POINT('Ctrl Pts',(29.0554605281726,-1.99359903284624,-11.5780362187396)) ;
#59850=CARTESIAN_POINT('Ctrl Pts',(29.0584648442791,-2.00943761463625,-11.5793391039616)) ;
#59851=CARTESIAN_POINT('Ctrl Pts',(29.0599760966161,-2.01739923214533,-11.5799913538457)) ;
#59852=CARTESIAN_POINT('Ctrl Pts',(29.0630151083938,-2.03340107088851,-11.5812983106997)) ;
#59853=CARTESIAN_POINT('Ctrl Pts',(29.0645428681356,-2.04144129212701,-11.5819530169154)) ;
#59854=CARTESIAN_POINT('Ctrl Pts',(29.0691486954484,-2.06567079163896,-11.5839213103865)) ;
#59855=CARTESIAN_POINT('Ctrl Pts',(29.0722492727184,-2.08196890224857,-11.5852391668774)) ;
#59856=CARTESIAN_POINT('Ctrl Pts',(29.0784997417023,-2.11480697633052,-11.587886143567)) ;
#59857=CARTESIAN_POINT('Ctrl Pts',(29.0816496513105,-2.13134694000775,-11.5892152189681)) ;
#59858=CARTESIAN_POINT('Ctrl Pts',(29.0879887575836,-2.16462035934258,-11.5918827990063)) ;
#59859=CARTESIAN_POINT('Ctrl Pts',(29.0911779600734,-2.18135381116105,-11.5932212868798)) ;
#59860=CARTESIAN_POINT('Ctrl Pts',(29.097585914687,-2.21496583380245,-11.5959051228844)) ;
#59861=CARTESIAN_POINT('Ctrl Pts',(29.1008046676486,-2.2318444046333,-11.597250468916)) ;
#59862=CARTESIAN_POINT('Ctrl Pts',(29.1104908766021,-2.2826252500142,-11.6012923700042)) ;
#59863=CARTESIAN_POINT('Ctrl Pts',(29.1169882557135,-2.31667265716275,-11.6039948555289)) ;
#59864=CARTESIAN_POINT('Ctrl Pts',(29.1299871384566,-2.38476758990642,-11.6093895409454)) ;
#59865=CARTESIAN_POINT('Ctrl Pts',(29.1364886558516,-2.4188151018372,-11.6120816986642)) ;
#59866=CARTESIAN_POINT('Ctrl Pts',(29.1494208066684,-2.48652329463723,-11.617427940203)) ;
#59867=CARTESIAN_POINT('Ctrl Pts',(29.1558514467138,-2.52018397555204,-11.620082007424)) ;
#59868=CARTESIAN_POINT('Ctrl Pts',(29.1749249846731,-2.62000539185675,-11.6279442948498)) ;
#59869=CARTESIAN_POINT('Ctrl Pts',(29.1873494574745,-2.68500550045174,-11.633052708379)) ;
#59870=CARTESIAN_POINT('Ctrl Pts',(29.2121491155211,-2.81472076007776,-11.6432341376143)) ;
#59871=CARTESIAN_POINT('Ctrl Pts',(29.2251571264759,-2.88274300453423,-11.6485653289196)) ;
#59872=CARTESIAN_POINT('Ctrl Pts',(29.2512562758467,-3.01919807609263,-11.6592483178059)) ;
#59873=CARTESIAN_POINT('Ctrl Pts',(29.2643474287702,-3.08763090326719,-11.6646000790163)) ;
#59874=CARTESIAN_POINT('Ctrl Pts',(29.2906093238418,-3.22489389275181,-11.6753256915392)) ;
#59875=CARTESIAN_POINT('Ctrl Pts',(29.3037800718641,-3.29372405504827,-11.6806995281003)) ;
#59876=CARTESIAN_POINT('Ctrl Pts',(29.3301979489162,-3.43176846859418,-11.6914699476084)) ;
#59877=CARTESIAN_POINT('Ctrl Pts',(29.3434450787023,-3.50098271984707,-11.6968665286563)) ;
#59878=CARTESIAN_POINT('Ctrl Pts',(29.3832965163599,-3.70918173910975,-11.7130906509313)) ;
#59879=CARTESIAN_POINT('Ctrl Pts',(29.4100108320053,-3.84872277196881,-11.7239526726309)) ;
#59880=CARTESIAN_POINT('Ctrl Pts',(29.463710046215,-4.12918225244752,-11.7457666556354)) ;
#59881=CARTESIAN_POINT('Ctrl Pts',(29.4906949669058,-4.27010070014659,-11.7567185614512)) ;
#59882=CARTESIAN_POINT('Ctrl Pts',(29.5449136076951,-4.5532090553379,-11.7787078273763)) ;
#59883=CARTESIAN_POINT('Ctrl Pts',(29.5721473374809,-4.69539896192083,-11.7897451626647)) ;
#59884=CARTESIAN_POINT('Ctrl Pts',(29.6268422993657,-4.98094427794184,-11.8118995803103)) ;
#59885=CARTESIAN_POINT('Ctrl Pts',(29.6543035363965,-5.12429968739496,-11.823016650298)) ;
#59886=CARTESIAN_POINT('Ctrl Pts',(29.7094325037144,-5.41207005497427,-11.8453241087356)) ;
#59887=CARTESIAN_POINT('Ctrl Pts',(29.7371002364177,-5.55648501309814,-11.8565144911195)) ;
#59888=CARTESIAN_POINT('Ctrl Pts',(29.7926213687897,-5.84626852432184,-11.8789616873085)) ;
#59889=CARTESIAN_POINT('Ctrl Pts',(29.8204747688937,-5.991637077423,-11.8902185000195)) ;
#59890=CARTESIAN_POINT('Ctrl Pts',(29.9042824088571,-6.42901419915437,-11.92407780665)) ;
#59891=CARTESIAN_POINT('Ctrl Pts',(29.9604840591669,-6.72229422551734,-11.9467692397323)) ;
#59892=CARTESIAN_POINT('Ctrl Pts',(30.073382389645,-7.31139720219581,-11.9923294645172)) ;
#59893=CARTESIAN_POINT('Ctrl Pts',(30.1300790840833,-7.60722015254495,-12.0151982204241)) ;
#59894=CARTESIAN_POINT('Ctrl Pts',(30.2438035110593,-8.200561345854,-12.0610514214145)) ;
#59895=CARTESIAN_POINT('Ctrl Pts',(30.3008312506642,-8.49807958881067,-12.0840358487589)) ;
#59896=CARTESIAN_POINT('Ctrl Pts',(30.4150541835392,-9.09396373680619,-12.1300577013257)) ;
#59897=CARTESIAN_POINT('Ctrl Pts',(30.4722493801187,-9.39232964185194,-12.1530951182446)) ;
#59898=CARTESIAN_POINT('Ctrl Pts',(30.6438411606855,-10.2874274051715,-12.2221918581039)) ;
#59899=CARTESIAN_POINT('Ctrl Pts',(30.7582438742163,-10.8841592962013,-12.2682358153304)) ;
#59900=CARTESIAN_POINT('Ctrl Pts',(30.9857608719517,-12.0708421120912,-12.3597714289845)) ;
#59901=CARTESIAN_POINT('Ctrl Pts',(31.0988751847915,-12.6607930370028,-12.4052630135689)) ;
#59902=CARTESIAN_POINT('Ctrl Pts',(31.3225120133624,-13.8271328594513,-12.4951790207671)) ;
#59903=CARTESIAN_POINT('Ctrl Pts',(31.4373907777609,-14.4262400706049,-12.5413543921016)) ;
#59904=CARTESIAN_POINT('Ctrl Pts',(31.5501658085507,-15.0143581153283,-12.5866741590384)) ;
#59905=CARTESIAN_POINT('Ctrl Pts',(31.554439204467,-15.0366437072152,-12.5883914511059)) ;
#59906=CARTESIAN_POINT('Ctrl Pts',(31.565410601367,-15.0366437072152,-12.5608553212663)) ;
#59907=CARTESIAN_POINT('Ctrl Pts',(31.561127154397,-15.0143581154633,-12.5591632555168)) ;
#59908=CARTESIAN_POINT('Ctrl Pts',(31.5568406253047,-14.9920565142548,-12.5574699867564)) ;
#59909=CARTESIAN_POINT('Ctrl Pts',(31.4437198542653,-14.403521757529,-12.5127852997407)) ;
#59910=CARTESIAN_POINT('Ctrl Pts',(31.3329303683987,-13.8271328601355,-12.4690309217221)) ;
#59911=CARTESIAN_POINT('Ctrl Pts',(31.1087358495905,-12.6607930379712,-12.3805146116334)) ;
#59912=CARTESIAN_POINT('Ctrl Pts',(30.9953308303239,-12.0708421132033,-12.335752645243)) ;
#59913=CARTESIAN_POINT('Ctrl Pts',(30.767205523712,-10.8841592976026,-12.2457437719057)) ;
#59914=CARTESIAN_POINT('Ctrl Pts',(30.6524852649845,-10.2874274067182,-12.2004967931075)) ;
#59915=CARTESIAN_POINT('Ctrl Pts',(30.4803926152741,-9.39232964361678,-12.1326571401289)) ;
#59916=CARTESIAN_POINT('Ctrl Pts',(30.4230263412627,-9.09396373864371,-12.1100490952274)) ;
#59917=CARTESIAN_POINT('Ctrl Pts',(30.3084518038435,-8.49807959079342,-12.064909703605)) ;
#59918=CARTESIAN_POINT('Ctrl Pts',(30.2512435437427,-8.20056134790925,-12.0423783485818)) ;
#59919=CARTESIAN_POINT('Ctrl Pts',(30.1371469009566,-7.60722015474479,-11.9974593389122)) ;
#59920=CARTESIAN_POINT('Ctrl Pts',(30.0802585253396,-7.31139720446773,-11.9750716665277)) ;
#59921=CARTESIAN_POINT('Ctrl Pts',(29.9669631044646,-6.72229422793283,-11.9305080635682)) ;
#59922=CARTESIAN_POINT('Ctrl Pts',(29.9105560734644,-6.42901420164131,-11.9083320971897)) ;
#59923=CARTESIAN_POINT('Ctrl Pts',(29.8264270778358,-5.99163708001652,-11.8752793325204)) ;
#59924=CARTESIAN_POINT('Ctrl Pts',(29.7984643309233,-5.84626852695081,-11.8642969596244)) ;
#59925=CARTESIAN_POINT('Ctrl Pts',(29.7427193144565,-5.55648501579772,-11.842411670182)) ;
#59926=CARTESIAN_POINT('Ctrl Pts',(29.714937045338,-5.41207005770904,-11.8315087525432)) ;
#59927=CARTESIAN_POINT('Ctrl Pts',(29.6595728365084,-5.12429969019985,-11.8097917058187)) ;
#59928=CARTESIAN_POINT('Ctrl Pts',(29.6319908992134,-4.98094428078168,-11.7989775706709)) ;
#59929=CARTESIAN_POINT('Ctrl Pts',(29.5770470224415,-4.69539896483025,-11.7774478823226)) ;
#59930=CARTESIAN_POINT('Ctrl Pts',(29.549685087891,-4.55320905828197,-11.7667323167496)) ;
#59931=CARTESIAN_POINT('Ctrl Pts',(29.4952005928358,-4.27010070315964,-11.7454102947565)) ;
#59932=CARTESIAN_POINT('Ctrl Pts',(29.468078042368,-4.12918225549492,-11.7348038136532)) ;
#59933=CARTESIAN_POINT('Ctrl Pts',(29.4140911906375,-3.84872277508455,-11.7137117464274)) ;
#59934=CARTESIAN_POINT('Ctrl Pts',(29.3872269114725,-3.70918174225949,-11.7032261047998)) ;
#59935=CARTESIAN_POINT('Ctrl Pts',(29.3471376272874,-3.50098272304754,-11.6875989323238)) ;
#59936=CARTESIAN_POINT('Ctrl Pts',(29.3338090449177,-3.43176847181153,-11.6824067818549)) ;
#59937=CARTESIAN_POINT('Ctrl Pts',(29.307222973611,-3.29372405829925,-11.6720584981133)) ;
#59938=CARTESIAN_POINT('Ctrl Pts',(29.2939654854284,-3.22489389601956,-11.6669023629481)) ;
#59939=CARTESIAN_POINT('Ctrl Pts',(29.2675234700757,-3.08763090656839,-11.6566288182608)) ;
#59940=CARTESIAN_POINT('Ctrl Pts',(29.2543389487858,-3.01919807941051,-11.6515113939891)) ;
#59941=CARTESIAN_POINT('Ctrl Pts',(29.2280443983299,-2.88274300788535,-11.6413188248645)) ;
#59942=CARTESIAN_POINT('Ctrl Pts',(29.2149343836421,-2.81472076344547,-11.6362436436338)) ;
#59943=CARTESIAN_POINT('Ctrl Pts',(29.1899281802654,-2.68500550351773,-11.626580603919)) ;
#59944=CARTESIAN_POINT('Ctrl Pts',(29.1773950157388,-2.62000539458853,-11.621744985863)) ;
#59945=CARTESIAN_POINT('Ctrl Pts',(29.1581408222584,-2.52018397777059,-11.614336109319)) ;
#59946=CARTESIAN_POINT('Ctrl Pts',(29.1516470059532,-2.48652329668272,-11.611840602457)) ;
#59947=CARTESIAN_POINT('Ctrl Pts',(29.1385817152791,-2.41881510353456,-11.6068285165685)) ;
#59948=CARTESIAN_POINT('Ctrl Pts',(29.132010247518,-2.38476759142876,-11.6043119209325)) ;
#59949=CARTESIAN_POINT('Ctrl Pts',(29.1188631949375,-2.31667265833498,-11.5992891135706)) ;
#59950=CARTESIAN_POINT('Ctrl Pts',(29.1122876291262,-2.2826252510114,-11.5967828617679)) ;
#59951=CARTESIAN_POINT('Ctrl Pts',(29.1024758718508,-2.2318444053694,-11.5930560630614)) ;
#59952=CARTESIAN_POINT('Ctrl Pts',(29.0992138779589,-2.21496583445174,-11.591819243533)) ;
#59953=CARTESIAN_POINT('Ctrl Pts',(29.0927160591955,-2.18135381163753,-11.5893609494406)) ;
#59954=CARTESIAN_POINT('Ctrl Pts',(29.0894802351616,-2.16462035973303,-11.5881394727713)) ;
#59955=CARTESIAN_POINT('Ctrl Pts',(29.0830435792027,-2.13134694022715,-11.5857167238876)) ;
#59956=CARTESIAN_POINT('Ctrl Pts',(29.0798427545775,-2.11480697646486,-11.5845154354957)) ;
#59957=CARTESIAN_POINT('Ctrl Pts',(29.0734846178031,-2.08196890221408,-11.5821386844894)) ;
#59958=CARTESIAN_POINT('Ctrl Pts',(29.0703273234694,-2.0656707915207,-11.5809631770477)) ;
#59959=CARTESIAN_POINT('Ctrl Pts',(29.0656299192246,-2.0414412918842,-11.579224724275)) ;
#59960=CARTESIAN_POINT('Ctrl Pts',(29.0640705314266,-2.03340107060426,-11.5786493984716)) ;
#59961=CARTESIAN_POINT('Ctrl Pts',(29.060965429039,-2.01739923177882,-11.5775083164946)) ;
#59962=CARTESIAN_POINT('Ctrl Pts',(29.059419714753,-2.00943761422882,-11.5769425595576)) ;
#59963=CARTESIAN_POINT('Ctrl Pts',(29.0563426013253,-1.99359903235739,-11.5758223817893)) ;
#59964=CARTESIAN_POINT('Ctrl Pts',(29.0548112128256,-1.98572206821069,-11.575267934346)) ;
#59965=CARTESIAN_POINT('Ctrl Pts',(29.0525250409775,-1.97397465373301,-11.5744468630235)) ;
#59966=CARTESIAN_POINT('Ctrl Pts',(29.0517647978228,-1.9700701876343,-11.5741749502126)) ;
#59967=CARTESIAN_POINT('Ctrl Pts',(29.0502478835027,-1.96228469125286,-11.5736352444845)) ;
#59968=CARTESIAN_POINT('Ctrl Pts',(29.049491213007,-1.95840366095669,-11.5733674498795)) ;
#59969=CARTESIAN_POINT('Ctrl Pts',(29.0479803339922,-1.9506609828574,-11.5728365033947)) ;
#59970=CARTESIAN_POINT('Ctrl Pts',(29.0471859893661,-1.94659361612655,-11.5725592265675)) ;
#59971=CARTESIAN_POINT('Ctrl Pts',(29.0455572224161,-1.93826542844876,-11.5719972491222)) ;
#59972=CARTESIAN_POINT('Ctrl Pts',(29.0447228269808,-1.93400460682272,-11.5717124806397)) ;
#59973=CARTESIAN_POINT('Ctrl Pts',(29.0434682476483,-1.92761363729763,-11.5712929694538)) ;
#59974=CARTESIAN_POINT('Ctrl Pts',(29.0430495532631,-1.92548337120945,-11.5711544223689)) ;
#59975=CARTESIAN_POINT('Ctrl Pts',(29.0422154605149,-1.9212471610181,-11.5708826354932)) ;
#59976=CARTESIAN_POINT('Ctrl Pts',(29.041800075323,-1.91914121645887,-11.5707493623905)) ;
#59977=CARTESIAN_POINT('Ctrl Pts',(29.0411824150817,-1.91601870660613,-11.5705561828204)) ;
#59978=CARTESIAN_POINT('Ctrl Pts',(29.04097742769,-1.91498394163286,-11.5704929223976)) ;
#59979=CARTESIAN_POINT('Ctrl Pts',(29.0405696466495,-1.91292957956788,-11.5703693643508)) ;
#59980=CARTESIAN_POINT('Ctrl Pts',(29.0403668539521,-1.91190998243237,-11.5703090643144)) ;
#59981=CARTESIAN_POINT('Ctrl Pts',(29.0399636978678,-1.90988898797118,-11.5701925286259)) ;
#59982=CARTESIAN_POINT('Ctrl Pts',(29.0397633493576,-1.90888759247266,-11.5701362566561)) ;
#59983=CARTESIAN_POINT('Ctrl Pts',(29.0394645067919,-1.90740143702365,-11.5700565302644)) ;
#59984=CARTESIAN_POINT('Ctrl Pts',(29.039365169076,-1.9069087086778,-11.5700307442789)) ;
#59985=CARTESIAN_POINT('Ctrl Pts',(29.0391668950545,-1.90592895339284,-11.5699813481084)) ;
#59986=CARTESIAN_POINT('Ctrl Pts',(29.0390679675556,-1.90544192580431,-11.5699577154576)) ;
#59987=CARTESIAN_POINT('Ctrl Pts',(29.03891816831,-1.9047090240292,-11.5699244824112)) ;
#59988=CARTESIAN_POINT('Ctrl Pts',(29.0388645915097,-1.90444770688011,-11.569913048924)) ;
#59989=CARTESIAN_POINT('Ctrl Pts',(29.0387543560926,-1.90391283053387,-11.5698910816268)) ;
#59990=CARTESIAN_POINT('Ctrl Pts',(29.0386976993307,-1.90363927114993,-11.5698805430576)) ;
#59991=CARTESIAN_POINT('Ctrl Pts',(29.0385834427038,-1.90309246529325,-11.5698620076366)) ;
#59992=CARTESIAN_POINT('Ctrl Pts',(29.0385258858671,-1.90281925763486,-11.5698539244633)) ;
#59993=CARTESIAN_POINT('Ctrl Pts',(29.0382498911084,-1.90163369484209,-11.5698846841972)) ;
#59994=CARTESIAN_POINT('Ctrl Pts',(29.038238558044,-1.90158501254251,-11.5698859472721)) ;
#59995=CARTESIAN_POINT('Ctrl Pts',(29.0382272249795,-1.90153633024293,-11.569887210347)) ;
#59996=CARTESIAN_POINT('',(33.9237617799844,-15.0366437072151,1.82445047330668)) ;
#59997=CARTESIAN_POINT('',(33.9221570292818,-15.0366437072151,1.85404835843738)) ;
#59998=CARTESIAN_POINT('Origin',(-1.36393928288321,-21.6462763158694,-0.073950639135127)) ;
#59999=CARTESIAN_POINT('',(31.2124507878034,-1.90153624155895,1.69228989918397)) ;
#60000=CARTESIAN_POINT('Ctrl Pts',(31.2124508063865,-1.90153633154746,1.69228989994415)) ;
#60001=CARTESIAN_POINT('Ctrl Pts',(31.212461175561,-1.90158488722844,1.69228399858286)) ;
#60002=CARTESIAN_POINT('Ctrl Pts',(31.2126377175942,-1.90241157971636,1.6921835240153)) ;
#60003=CARTESIAN_POINT('Ctrl Pts',(31.2127209037029,-1.90280827097885,1.69216349692496)) ;
#60004=CARTESIAN_POINT('Ctrl Pts',(31.2127775376793,-1.90307911546552,1.69215281262026)) ;
#60005=CARTESIAN_POINT('Ctrl Pts',(31.2128907504375,-1.90362119469672,1.69213395170716)) ;
#60006=CARTESIAN_POINT('Ctrl Pts',(31.2129473160421,-1.90389239066645,1.69212587012815)) ;
#60007=CARTESIAN_POINT('Ctrl Pts',(31.2130578371091,-1.90442264746974,1.69211152595285)) ;
#60008=CARTESIAN_POINT('Ctrl Pts',(31.2131117923418,-1.90468170848452,1.69210526828505)) ;
#60009=CARTESIAN_POINT('Ctrl Pts',(31.213263036536,-1.90540821834563,1.69208896765253)) ;
#60010=CARTESIAN_POINT('Ctrl Pts',(31.2133634468165,-1.90589097623944,1.69207979306088)) ;
#60011=CARTESIAN_POINT('Ctrl Pts',(31.2135653350542,-1.90686214240077,1.69206332035544)) ;
#60012=CARTESIAN_POINT('Ctrl Pts',(31.2136668118428,-1.90735055131874,1.69205604627652)) ;
#60013=CARTESIAN_POINT('Ctrl Pts',(31.2139727705461,-1.90882367886906,1.6920361944457)) ;
#60014=CARTESIAN_POINT('Ctrl Pts',(31.2141787825174,-1.90981629627927,1.69202554768393)) ;
#60015=CARTESIAN_POINT('Ctrl Pts',(31.2145943792177,-1.91181957543587,1.69200723738784)) ;
#60016=CARTESIAN_POINT('Ctrl Pts',(31.2148039614514,-1.91283023535738,1.69199961290675)) ;
#60017=CARTESIAN_POINT('Ctrl Pts',(31.215226124221,-1.91486659038896,1.69198645586192)) ;
#60018=CARTESIAN_POINT('Ctrl Pts',(31.2154387046288,-1.91589228554187,1.69198092582033)) ;
#60019=CARTESIAN_POINT('Ctrl Pts',(31.2160800554371,-1.91898742680707,1.69196668346609)) ;
#60020=CARTESIAN_POINT('Ctrl Pts',(31.2165124347933,-1.92107491347353,1.69196027231138)) ;
#60021=CARTESIAN_POINT('Ctrl Pts',(31.2173819724023,-1.92527399569929,1.6919513369368)) ;
#60022=CARTESIAN_POINT('Ctrl Pts',(31.2178191288148,-1.92738559171555,1.69194884840311)) ;
#60023=CARTESIAN_POINT('Ctrl Pts',(31.2191304096143,-1.93372055099077,1.6919455119432)) ;
#60024=CARTESIAN_POINT('Ctrl Pts',(31.2200043381773,-1.93794403242011,1.69194872685841)) ;
#60025=CARTESIAN_POINT('Ctrl Pts',(31.2217122048351,-1.94619923694316,1.69196075730605)) ;
#60026=CARTESIAN_POINT('Ctrl Pts',(31.222546139137,-1.95023096071567,1.6919696453857)) ;
#60027=CARTESIAN_POINT('Ctrl Pts',(31.2241333801421,-1.95790548260028,1.69198990256225)) ;
#60028=CARTESIAN_POINT('Ctrl Pts',(31.2249288593706,-1.96175219546279,1.69200182885001)) ;
#60029=CARTESIAN_POINT('Ctrl Pts',(31.226524476387,-1.96946884984108,1.69202842779924)) ;
#60030=CARTESIAN_POINT('Ctrl Pts',(31.2273246140806,-1.97333879137023,1.69204310224879)) ;
#60031=CARTESIAN_POINT('Ctrl Pts',(31.2297318261205,-1.98498233146023,1.69209042504112)) ;
#60032=CARTESIAN_POINT('Ctrl Pts',(31.2313457018942,-1.99278964510905,1.6921263257119)) ;
#60033=CARTESIAN_POINT('Ctrl Pts',(31.2345904888783,-2.0084881776274,1.69220421002999)) ;
#60034=CARTESIAN_POINT('Ctrl Pts',(31.2362213985065,-2.01637939632246,1.69224622219019)) ;
#60035=CARTESIAN_POINT('Ctrl Pts',(31.2394990884388,-2.03223974253541,1.69233492278662)) ;
#60036=CARTESIAN_POINT('Ctrl Pts',(31.2411458686997,-2.04020887005775,1.69238161202648)) ;
#60037=CARTESIAN_POINT('Ctrl Pts',(31.2461082290652,-2.06422412624885,1.69252732779402)) ;
#60038=CARTESIAN_POINT('Ctrl Pts',(31.2494458335295,-2.08037812508227,1.69263190102892)) ;
#60039=CARTESIAN_POINT('Ctrl Pts',(31.2561700891972,-2.11292583745181,1.69285147290656)) ;
#60040=CARTESIAN_POINT('Ctrl Pts',(31.2595567378426,-2.12931955119283,1.69296651950916)) ;
#60041=CARTESIAN_POINT('Ctrl Pts',(31.2663692987432,-2.16229876012589,1.69320450644542)) ;
#60042=CARTESIAN_POINT('Ctrl Pts',(31.2697952092503,-2.17888425147949,1.6933274643675)) ;
#60043=CARTESIAN_POINT('Ctrl Pts',(31.2766764656943,-2.21219907029455,1.69357952704175)) ;
#60044=CARTESIAN_POINT('Ctrl Pts',(31.2801318115104,-2.22892839776393,1.69370863404421)) ;
#60045=CARTESIAN_POINT('Ctrl Pts',(31.2905272293254,-2.27926023016279,1.69410317044972)) ;
#60046=CARTESIAN_POINT('Ctrl Pts',(31.2974966855476,-2.31300658479306,1.69437574300689)) ;
#60047=CARTESIAN_POINT('Ctrl Pts',(31.3114350251233,-2.38049941248962,1.69493190615983)) ;
#60048=CARTESIAN_POINT('Ctrl Pts',(31.3184039032708,-2.41424587189324,1.69521554061887)) ;
#60049=CARTESIAN_POINT('Ctrl Pts',(31.332262048329,-2.48135538068444,1.69578759918834)) ;
#60050=CARTESIAN_POINT('Ctrl Pts',(31.3391513142871,-2.51471843011748,1.69607604104233)) ;
#60051=CARTESIAN_POINT('Ctrl Pts',(31.3595810816876,-2.61365721512364,1.69694041210369)) ;
#60052=CARTESIAN_POINT('Ctrl Pts',(31.3728835588276,-2.67808258704843,1.69751527163408)) ;
#60053=CARTESIAN_POINT('Ctrl Pts',(31.3994174846424,-2.80659298449379,1.69867586291107)) ;
#60054=CARTESIAN_POINT('Ctrl Pts',(31.4133256032471,-2.87395568035031,1.69929267964525)) ;
#60055=CARTESIAN_POINT('Ctrl Pts',(31.4412251194173,-3.00908767377159,1.70054240363067)) ;
#60056=CARTESIAN_POINT('Ctrl Pts',(31.455216514895,-3.07685697140873,1.70117534966788)) ;
#60057=CARTESIAN_POINT('Ctrl Pts',(31.4832800222044,-3.21278904930444,1.70245451856394)) ;
#60058=CARTESIAN_POINT('Ctrl Pts',(31.4973521331798,-3.28095182954947,1.70310075716268)) ;
#60059=CARTESIAN_POINT('Ctrl Pts',(31.5255744612477,-3.41765775489871,1.70440458104699)) ;
#60060=CARTESIAN_POINT('Ctrl Pts',(31.5397246782305,-3.4862009000063,1.70506216835304)) ;
#60061=CARTESIAN_POINT('Ctrl Pts',(31.5822885313072,-3.69238120731966,1.70704982916459)) ;
#60062=CARTESIAN_POINT('Ctrl Pts',(31.6108153752653,-3.83056924086275,1.70839469325321)) ;
#60063=CARTESIAN_POINT('Ctrl Pts',(31.668149650939,-4.10830936735011,1.71111617408425)) ;
#60064=CARTESIAN_POINT('Ctrl Pts',(31.6969570794573,-4.24786146037364,1.71249285009703)) ;
#60065=CARTESIAN_POINT('Ctrl Pts',(31.7548310815494,-4.52822477818846,1.7152729122382)) ;
#60066=CARTESIAN_POINT('Ctrl Pts',(31.7838976535024,-4.66903600207234,1.7166763247973)) ;
#60067=CARTESIAN_POINT('Ctrl Pts',(31.8422684285719,-4.95181265200927,1.71950612302232)) ;
#60068=CARTESIAN_POINT('Ctrl Pts',(31.8715726309751,-5.09377807807733,1.72093252190176)) ;
#60069=CARTESIAN_POINT('Ctrl Pts',(31.9303971118103,-5.37875820553491,1.72380532693214)) ;
#60070=CARTESIAN_POINT('Ctrl Pts',(31.9599173898905,-5.52177290692212,1.72525173956014)) ;
#60071=CARTESIAN_POINT('Ctrl Pts',(32.0191524404763,-5.80874665865466,1.72816209630444)) ;
#60072=CARTESIAN_POINT('Ctrl Pts',(32.048867212918,-5.95270570900133,1.72962604159107)) ;
#60073=CARTESIAN_POINT('Ctrl Pts',(32.138270873612,-6.38584199444269,1.73404093995574)) ;
#60074=CARTESIAN_POINT('Ctrl Pts',(32.1982191083803,-6.67627835925047,1.73701487958215)) ;
#60075=CARTESIAN_POINT('Ctrl Pts',(32.3186342423773,-7.25966935677229,1.74300929128555)) ;
#60076=CARTESIAN_POINT('Ctrl Pts',(32.3791011395381,-7.55262398951995,1.74602980162912)) ;
#60077=CARTESIAN_POINT('Ctrl Pts',(32.5003805641629,-8.14021211025548,1.75210457488547)) ;
#60078=CARTESIAN_POINT('Ctrl Pts',(32.5611930905981,-8.43484559824006,1.75515885676166)) ;
#60079=CARTESIAN_POINT('Ctrl Pts',(32.6829906805412,-9.02495201759556,1.76128948583913)) ;
#60080=CARTESIAN_POINT('Ctrl Pts',(32.7439757435688,-9.3204249489734,1.76436584192077)) ;
#60081=CARTESIAN_POINT('Ctrl Pts',(32.9269300423157,-10.2068437912566,1.77361151529095)) ;
#60082=CARTESIAN_POINT('Ctrl Pts',(33.0488983929961,-10.7977897348994,1.77979728107415)) ;
#60083=CARTESIAN_POINT('Ctrl Pts',(33.2914474187023,-11.9729664053665,1.79212964973308)) ;
#60084=CARTESIAN_POINT('Ctrl Pts',(33.4120280895723,-12.5571971322423,1.79827632943994)) ;
#60085=CARTESIAN_POINT('Ctrl Pts',(33.650416233567,-13.7122280573775,1.81045128027227)) ;
#60086=CARTESIAN_POINT('Ctrl Pts',(33.7682237047013,-14.2830282556339,1.81647958809695)) ;
#60087=CARTESIAN_POINT('Ctrl Pts',(33.8972495735035,-14.9081862858531,1.82309151287019)) ;
#60088=CARTESIAN_POINT('Ctrl Pts',(33.9105199299277,-14.9724840415154,1.82377166717193)) ;
#60089=CARTESIAN_POINT('Ctrl Pts',(33.9237617800355,-15.0366437072146,1.82445047235355)) ;
#60090=CARTESIAN_POINT('Ctrl Pts',(33.9221570292296,-15.0366437072146,1.85404835939107)) ;
#60091=CARTESIAN_POINT('Ctrl Pts',(33.908919411658,-14.972484041484,1.8532914895515)) ;
#60092=CARTESIAN_POINT('Ctrl Pts',(33.8956533090097,-14.9081862857901,1.85253287884846)) ;
#60093=CARTESIAN_POINT('Ctrl Pts',(33.7666689205491,-14.2830282555071,1.84515589394836)) ;
#60094=CARTESIAN_POINT('Ctrl Pts',(33.6489002671268,-13.7122280572179,1.83841163542848)) ;
#60095=CARTESIAN_POINT('Ctrl Pts',(33.4105932208991,-12.5571971320165,1.82474092404397)) ;
#60096=CARTESIAN_POINT('Ctrl Pts',(33.2900548261047,-11.9729664051072,1.81781450787719)) ;
#60097=CARTESIAN_POINT('Ctrl Pts',(33.0475942695711,-10.7977897345726,1.8038504210827)) ;
#60098=CARTESIAN_POINT('Ctrl Pts',(32.9256721036565,-10.2068437908959,1.7968128272885)) ;
#60099=CARTESIAN_POINT('Ctrl Pts',(32.7427906577076,-9.32042494856183,1.78622346292756)) ;
#60100=CARTESIAN_POINT('Ctrl Pts',(32.6818304791294,-9.02495201716702,1.78268814012078)) ;
#60101=CARTESIAN_POINT('Ctrl Pts',(32.5600840342718,-8.43484559777765,1.77561419531639)) ;
#60102=CARTESIAN_POINT('Ctrl Pts',(32.49929776751,-8.14021210977616,1.77207558219994)) ;
#60103=CARTESIAN_POINT('Ctrl Pts',(32.37807248954,-7.55262398900691,1.76500213252937)) ;
#60104=CARTESIAN_POINT('Ctrl Pts',(32.3176334773044,-7.25966935624243,1.76146731493739)) ;
#60105=CARTESIAN_POINT('Ctrl Pts',(32.1972761120659,-6.67627835868714,1.75440742105084)) ;
#60106=CARTESIAN_POINT('Ctrl Pts',(32.1373577569814,-6.38584199386269,1.75088238301948)) ;
#60107=CARTESIAN_POINT('Ctrl Pts',(32.0480008498943,-5.95270570839647,1.7456051650227)) ;
#60108=CARTESIAN_POINT('Ctrl Pts',(32.0183019863929,-5.80874665804157,1.74384779656639)) ;
#60109=CARTESIAN_POINT('Ctrl Pts',(31.9590995092937,-5.52177290629252,1.74033665714888)) ;
#60110=CARTESIAN_POINT('Ctrl Pts',(31.9295958956328,-5.37875820489711,1.73858288736032)) ;
#60111=CARTESIAN_POINT('Ctrl Pts',(31.8708056415613,-5.09377807742317,1.73507880675721)) ;
#60112=CARTESIAN_POINT('Ctrl Pts',(31.8415190008,-4.95181265134699,1.73332850242113)) ;
#60113=CARTESIAN_POINT('Ctrl Pts',(31.7831844427051,-4.66903600139383,1.72983072134243)) ;
#60114=CARTESIAN_POINT('Ctrl Pts',(31.7541365246517,-4.52822477750184,1.72808325781884)) ;
#60115=CARTESIAN_POINT('Ctrl Pts',(31.6963012048463,-4.24786145967095,1.72458974281748)) ;
#60116=CARTESIAN_POINT('Ctrl Pts',(31.6675138018479,-4.10830936663942,1.72284371779161)) ;
#60117=CARTESIAN_POINT('Ctrl Pts',(31.6102213783154,-3.83056924013612,1.71935031957733)) ;
#60118=CARTESIAN_POINT('Ctrl Pts',(31.5817163545517,-3.69238120658509,1.71760300565428)) ;
#60119=CARTESIAN_POINT('Ctrl Pts',(31.5391871086669,-3.48620089925991,1.71497705269782)) ;
#60120=CARTESIAN_POINT('Ctrl Pts',(31.5250487431677,-3.41765775414836,1.71410087762607)) ;
#60121=CARTESIAN_POINT('Ctrl Pts',(31.4968508874359,-3.28095182879129,1.71234568803049)) ;
#60122=CARTESIAN_POINT('Ctrl Pts',(31.4827913970942,-3.21278904854235,1.71146667552467)) ;
#60123=CARTESIAN_POINT('Ctrl Pts',(31.45475409678,-3.07685697063884,1.70970414701375)) ;
#60124=CARTESIAN_POINT('Ctrl Pts',(31.4407762859572,-3.00908767299782,1.70882064674741)) ;
#60125=CARTESIAN_POINT('Ctrl Pts',(31.4129051990138,-2.87395567956879,1.70704657649424)) ;
#60126=CARTESIAN_POINT('Ctrl Pts',(31.3990119207755,-2.8065929837084,1.70615604529268)) ;
#60127=CARTESIAN_POINT('Ctrl Pts',(31.3725080560023,-2.67808258636586,1.70444101112125)) ;
#60128=CARTESIAN_POINT('Ctrl Pts',(31.3592214053287,-2.61365721455308,1.70357425002237)) ;
#60129=CARTESIAN_POINT('Ctrl Pts',(31.3388179431848,-2.51471842971896,1.70222470770763)) ;
#60130=CARTESIAN_POINT('Ctrl Pts',(31.3319378763602,-2.48135538034391,1.70176659804155)) ;
#60131=CARTESIAN_POINT('Ctrl Pts',(31.3180991179551,-2.41424587166938,1.7008369741399)) ;
#60132=CARTESIAN_POINT('Ctrl Pts',(31.3111404254024,-2.3804994123244,1.70036547766291)) ;
#60133=CARTESIAN_POINT('Ctrl Pts',(31.2972236611806,-2.31300658474519,1.69941138097162)) ;
#60134=CARTESIAN_POINT('Ctrl Pts',(31.290265589944,-2.27926023017359,1.69892882493465)) ;
#60135=CARTESIAN_POINT('Ctrl Pts',(31.2798884536427,-2.22892839786223,1.69819710618152)) ;
#60136=CARTESIAN_POINT('Ctrl Pts',(31.276439404296,-2.21219907042198,1.69795186774684)) ;
#60137=CARTESIAN_POINT('Ctrl Pts',(31.2695712333151,-2.17888425166482,1.69745845812796)) ;
#60138=CARTESIAN_POINT('Ctrl Pts',(31.2661521115581,-2.16229876034004,1.697210289186)) ;
#60139=CARTESIAN_POINT('Ctrl Pts',(31.2593537552793,-2.12931955146433,1.69671031363605)) ;
#60140=CARTESIAN_POINT('Ctrl Pts',(31.255974520594,-2.11292583775185,1.69645852469451)) ;
#60141=CARTESIAN_POINT('Ctrl Pts',(31.2492659429168,-2.08037812543891,1.69594978951167)) ;
#60142=CARTESIAN_POINT('Ctrl Pts',(31.2459365972835,-2.06422412663359,1.69569289121035)) ;
#60143=CARTESIAN_POINT('Ctrl Pts',(31.2409875718499,-2.04020887048424,1.69530122725515)) ;
#60144=CARTESIAN_POINT('Ctrl Pts',(31.2393453970935,-2.03223974297573,1.69516959453648)) ;
#60145=CARTESIAN_POINT('Ctrl Pts',(31.2360773309043,-2.01637939679035,1.69490339454841)) ;
#60146=CARTESIAN_POINT('Ctrl Pts',(31.2344514394269,-2.00848817810898,1.69476882809305)) ;
#60147=CARTESIAN_POINT('Ctrl Pts',(31.2312172527528,-1.99278964561794,1.69449543266551)) ;
#60148=CARTESIAN_POINT('Ctrl Pts',(31.2296089560453,-1.98498233198264,1.69435663222621)) ;
#60149=CARTESIAN_POINT('Ctrl Pts',(31.2272107386957,-1.97333879191288,1.69414341220993)) ;
#60150=CARTESIAN_POINT('Ctrl Pts',(31.2264137048588,-1.96946885039057,1.69407149051786)) ;
#60151=CARTESIAN_POINT('Ctrl Pts',(31.2248245655682,-1.96175219602569,1.69392541699786)) ;
#60152=CARTESIAN_POINT('Ctrl Pts',(31.2240324600155,-1.95790548316983,1.69385126694658)) ;
#60153=CARTESIAN_POINT('Ctrl Pts',(31.2224523333459,-1.95023096151237,1.69369979443971)) ;
#60154=CARTESIAN_POINT('Ctrl Pts',(31.2216223266799,-1.94619923797133,1.69361846626251)) ;
#60155=CARTESIAN_POINT('Ctrl Pts',(31.219923170987,-1.93794403392222,1.69344577332982)) ;
#60156=CARTESIAN_POINT('Ctrl Pts',(31.2190540178856,-1.93372055273508,1.69335448113254)) ;
#60157=CARTESIAN_POINT('Ctrl Pts',(31.2177507846797,-1.9273855938235,1.69320938984938)) ;
#60158=CARTESIAN_POINT('Ctrl Pts',(31.2173164599791,-1.92527399792839,1.69315965099183)) ;
#60159=CARTESIAN_POINT('Ctrl Pts',(31.2164529857702,-1.92107491594367,1.69305675445358)) ;
#60160=CARTESIAN_POINT('Ctrl Pts',(31.2160238342365,-1.91898742939789,1.69300363238707)) ;
#60161=CARTESIAN_POINT('Ctrl Pts',(31.2153877829594,-1.9158922883102,1.69292013131494)) ;
#60162=CARTESIAN_POINT('Ctrl Pts',(31.2151770466207,-1.9148665932158,1.69289164972855)) ;
#60163=CARTESIAN_POINT('Ctrl Pts',(31.214758781138,-1.912830238301,1.69283292599244)) ;
#60164=CARTESIAN_POINT('Ctrl Pts',(31.2145512518463,-1.91181957843706,1.6928026864043)) ;
#60165=CARTESIAN_POINT('Ctrl Pts',(31.2141400711059,-1.90981629939523,1.69273954955086)) ;
#60166=CARTESIAN_POINT('Ctrl Pts',(31.2139364179195,-1.90882368204382,1.69270669130966)) ;
#60167=CARTESIAN_POINT('Ctrl Pts',(31.2136343991363,-1.90735055457764,1.69265387591175)) ;
#60168=CARTESIAN_POINT('Ctrl Pts',(31.2135343036764,-1.90686214568561,1.69263567297964)) ;
#60169=CARTESIAN_POINT('Ctrl Pts',(31.2133353799399,-1.90589097957973,1.69259746889062)) ;
#60170=CARTESIAN_POINT('Ctrl Pts',(31.2132365502277,-1.90540822171605,1.69257749172998)) ;
#60171=CARTESIAN_POINT('Ctrl Pts',(31.2130879550431,-1.90468171186102,1.69254493427891)) ;
#60172=CARTESIAN_POINT('Ctrl Pts',(31.2130349926572,-1.90442265081812,1.69253287985787)) ;
#60173=CARTESIAN_POINT('Ctrl Pts',(31.212926670338,-1.90389239396861,1.69250667033966)) ;
#60174=CARTESIAN_POINT('Ctrl Pts',(31.2128713100969,-1.90362119797884,1.6924925202205)) ;
#60175=CARTESIAN_POINT('Ctrl Pts',(31.2127608002093,-1.90307911869992,1.69246152943509)) ;
#60176=CARTESIAN_POINT('Ctrl Pts',(31.2127056533896,-1.90280827418462,1.69244478463953)) ;
#60177=CARTESIAN_POINT('Ctrl Pts',(31.2124703134312,-1.90163369130276,1.69230175545996)) ;
#60178=CARTESIAN_POINT('Ctrl Pts',(31.2124605599088,-1.90158501142511,1.69229582770205)) ;
#60179=CARTESIAN_POINT('Ctrl Pts',(31.2124508063865,-1.90153633154746,1.69228989994415)) ;
#60180=CARTESIAN_POINT('',(30.0223054639863,-15.0366437072153,15.9000442597426)) ;
#60181=CARTESIAN_POINT('',(30.008421202744,-15.0366437072153,15.9262327545903)) ;
#60182=CARTESIAN_POINT('Origin',(-1.20682669964218,-21.6462763158694,-0.639819022420589)) ;
#60183=CARTESIAN_POINT('',(27.6170790376327,-1.90153624262371,14.6416486341816)) ;
#60184=CARTESIAN_POINT('Ctrl Pts',(27.6170790543757,-1.90153633367698,14.6416486427733)) ;
#60185=CARTESIAN_POINT('Ctrl Pts',(27.6170909284475,-1.90158489354294,14.6416476702318)) ;
#60186=CARTESIAN_POINT('Ctrl Pts',(27.6172953105488,-1.90242072876526,14.6416309303902)) ;
#60187=CARTESIAN_POINT('Ctrl Pts',(27.6173800480628,-1.90282163236688,14.6416479748488)) ;
#60188=CARTESIAN_POINT('Ctrl Pts',(27.6174364929341,-1.90309535052159,14.6416622714043)) ;
#60189=CARTESIAN_POINT('Ctrl Pts',(27.6175482732284,-1.90364317745633,14.6416931294984)) ;
#60190=CARTESIAN_POINT('Ctrl Pts',(27.617603556575,-1.90391724740132,14.6417097721296)) ;
#60191=CARTESIAN_POINT('Ctrl Pts',(27.6177109618581,-1.9044531216928,14.6417436089329)) ;
#60192=CARTESIAN_POINT('Ctrl Pts',(27.6177630814776,-1.90471492622262,14.6417608075557)) ;
#60193=CARTESIAN_POINT('Ctrl Pts',(27.6179086726074,-1.90544920904616,14.6418101549156)) ;
#60194=CARTESIAN_POINT('Ctrl Pts',(27.6180046400594,-1.90593715923105,14.6418444219163)) ;
#60195=CARTESIAN_POINT('Ctrl Pts',(27.6181967623408,-1.9069187704498,14.6419151220803)) ;
#60196=CARTESIAN_POINT('Ctrl Pts',(27.6182929059663,-1.90741243213361,14.6419515766631)) ;
#60197=CARTESIAN_POINT('Ctrl Pts',(27.6185819071216,-1.90890140264463,14.6420633878904)) ;
#60198=CARTESIAN_POINT('Ctrl Pts',(27.6187753531983,-1.90990469490898,14.6421411566644)) ;
#60199=CARTESIAN_POINT('Ctrl Pts',(27.6191642634503,-1.91192951728473,14.6423009341078)) ;
#60200=CARTESIAN_POINT('Ctrl Pts',(27.6193597088623,-1.91295104556991,14.6423829773627)) ;
#60201=CARTESIAN_POINT('Ctrl Pts',(27.6197524670421,-1.91500929858626,14.6425502462511)) ;
#60202=CARTESIAN_POINT('Ctrl Pts',(27.6199497785913,-1.91604602336157,14.642635474202)) ;
#60203=CARTESIAN_POINT('Ctrl Pts',(27.6205440333576,-1.91917444700591,14.6428948333414)) ;
#60204=CARTESIAN_POINT('Ctrl Pts',(27.6209433157231,-1.92128437993827,14.6430725971919)) ;
#60205=CARTESIAN_POINT('Ctrl Pts',(27.6217446234793,-1.92552861272312,14.6434337015435)) ;
#60206=CARTESIAN_POINT('Ctrl Pts',(27.6221466321499,-1.92766291303188,14.6436170737834)) ;
#60207=CARTESIAN_POINT('Ctrl Pts',(27.6233507429032,-1.93406598522556,14.6441708786263)) ;
#60208=CARTESIAN_POINT('Ctrl Pts',(27.6241509510669,-1.93833487530353,14.6445449356854)) ;
#60209=CARTESIAN_POINT('Ctrl Pts',(27.6257123249711,-1.94667883314713,14.6452811783355)) ;
#60210=CARTESIAN_POINT('Ctrl Pts',(27.6264734566239,-1.95075390159159,14.6456434285222)) ;
#60211=CARTESIAN_POINT('Ctrl Pts',(27.6279207920016,-1.95851130719468,14.6463359871736)) ;
#60212=CARTESIAN_POINT('Ctrl Pts',(27.6286454412933,-1.96239975312801,14.6466847136137)) ;
#60213=CARTESIAN_POINT('Ctrl Pts',(27.6300978542299,-1.97020012554322,14.6473866516838)) ;
#60214=CARTESIAN_POINT('Ctrl Pts',(27.6308256170244,-1.9741120520386,14.6477398649235)) ;
#60215=CARTESIAN_POINT('Ctrl Pts',(27.6330137497998,-1.98588191268041,14.6488054035607)) ;
#60216=CARTESIAN_POINT('Ctrl Pts',(27.6344789863001,-1.99377392756813,14.6495235859559)) ;
#60217=CARTESIAN_POINT('Ctrl Pts',(27.6374225189715,-2.00964277263372,14.6509727376127)) ;
#60218=CARTESIAN_POINT('Ctrl Pts',(27.6389008016604,-2.01761960263699,14.651703732227)) ;
#60219=CARTESIAN_POINT('Ctrl Pts',(27.6418699519166,-2.03365201652979,14.65317672962)) ;
#60220=CARTESIAN_POINT('Ctrl Pts',(27.6433608190934,-2.0417076004239,14.6539187331361)) ;
#60221=CARTESIAN_POINT('Ctrl Pts',(27.6478512357866,-2.06598339581858,14.6561592501836)) ;
#60222=CARTESIAN_POINT('Ctrl Pts',(27.6508686476163,-2.08231264757128,14.6576721797494)) ;
#60223=CARTESIAN_POINT('Ctrl Pts',(27.6569440624088,-2.1152134659747,14.6607283838232)) ;
#60224=CARTESIAN_POINT('Ctrl Pts',(27.6600020427949,-2.13178503283035,14.6622717010056)) ;
#60225=CARTESIAN_POINT('Ctrl Pts',(27.6661506889654,-2.16512202815071,14.6653822147967)) ;
#60226=CARTESIAN_POINT('Ctrl Pts',(27.6692413457347,-2.18188745277619,14.6669494267159)) ;
#60227=CARTESIAN_POINT('Ctrl Pts',(27.6754470665202,-2.21556369825287,14.670101961583)) ;
#60228=CARTESIAN_POINT('Ctrl Pts',(27.6785621294787,-2.23247451911198,14.6716872865286)) ;
#60229=CARTESIAN_POINT('Ctrl Pts',(27.687931224249,-2.28335239179949,14.67646232417)) ;
#60230=CARTESIAN_POINT('Ctrl Pts',(27.6942091959947,-2.31746485344798,14.6796710353371)) ;
#60231=CARTESIAN_POINT('Ctrl Pts',(27.7067599654047,-2.38568989519371,14.6860982692832)) ;
#60232=CARTESIAN_POINT('Ctrl Pts',(27.7130327398153,-2.41980246162625,14.6893168298943)) ;
#60233=CARTESIAN_POINT('Ctrl Pts',(27.7255032417993,-2.48764002417549,14.6957245106718)) ;
#60234=CARTESIAN_POINT('Ctrl Pts',(27.7317009610019,-2.52136502033768,14.6989136466471)) ;
#60235=CARTESIAN_POINT('Ctrl Pts',(27.7500761798837,-2.62137716461915,14.7083790904372)) ;
#60236=CARTESIAN_POINT('Ctrl Pts',(27.7620357950646,-2.68650146817802,14.714553331675)) ;
#60237=CARTESIAN_POINT('Ctrl Pts',(27.7858983569804,-2.81647723388609,14.7268883261163)) ;
#60238=CARTESIAN_POINT('Ctrl Pts',(27.7984089201602,-2.88464214796207,14.7333648690751)) ;
#60239=CARTESIAN_POINT('Ctrl Pts',(27.8234997178078,-3.02138341989203,14.7463680676332)) ;
#60240=CARTESIAN_POINT('Ctrl Pts',(27.8360799339147,-3.08995977781875,14.752894757897)) ;
#60241=CARTESIAN_POINT('Ctrl Pts',(27.8613088744068,-3.22751066216052,14.7659945877528)) ;
#60242=CARTESIAN_POINT('Ctrl Pts',(27.8739575913392,-3.29648518856197,14.7725677413957)) ;
#60243=CARTESIAN_POINT('Ctrl Pts',(27.899321952774,-3.43481913589162,14.7857576231482)) ;
#60244=CARTESIAN_POINT('Ctrl Pts',(27.9120375963184,-3.50417855682328,14.7923743530643)) ;
#60245=CARTESIAN_POINT('Ctrl Pts',(27.9502821814213,-3.71281425181492,14.8122862828268)) ;
#60246=CARTESIAN_POINT('Ctrl Pts',(27.9759088285234,-3.8526479574165,14.8256431260594)) ;
#60247=CARTESIAN_POINT('Ctrl Pts',(28.0274063617563,-4.13369567233197,14.8525051109128)) ;
#60248=CARTESIAN_POINT('Ctrl Pts',(28.0532772198779,-4.27490968172529,14.8660103053992)) ;
#60249=CARTESIAN_POINT('Ctrl Pts',(28.1052456159083,-4.55861182703004,14.8931552682346)) ;
#60250=CARTESIAN_POINT('Ctrl Pts',(28.1313431411544,-4.70109996203175,14.9067950600667)) ;
#60251=CARTESIAN_POINT('Ctrl Pts',(28.1837466950101,-4.98724417938732,14.9341966563273)) ;
#60252=CARTESIAN_POINT('Ctrl Pts',(28.210052717377,-5.1309002617562,14.9479584725376)) ;
#60253=CARTESIAN_POINT('Ctrl Pts',(28.2628547252717,-5.41927419743718,14.9755922436653)) ;
#60254=CARTESIAN_POINT('Ctrl Pts',(28.2893507077362,-5.563992050747,14.9894642043592)) ;
#60255=CARTESIAN_POINT('Ctrl Pts',(28.3425138642521,-5.85438335238595,15.0173068271929)) ;
#60256=CARTESIAN_POINT('Ctrl Pts',(28.3691810377508,-6.00005680071646,15.0312774903742)) ;
#60257=CARTESIAN_POINT('Ctrl Pts',(28.4494109621522,-6.43835127486106,15.0733208029126)) ;
#60258=CARTESIAN_POINT('Ctrl Pts',(28.503202151952,-6.7322464251316,15.1015247071888)) ;
#60259=CARTESIAN_POINT('Ctrl Pts',(28.6112411485239,-7.32258498307404,15.1581955212879)) ;
#60260=CARTESIAN_POINT('Ctrl Pts',(28.6654889372312,-7.61902839077961,15.1866624651996)) ;
#60261=CARTESIAN_POINT('Ctrl Pts',(28.7742876405899,-8.21361405443553,15.2437741189221)) ;
#60262=CARTESIAN_POINT('Ctrl Pts',(28.8288385462861,-8.51175631038259,15.2724188456229)) ;
#60263=CARTESIAN_POINT('Ctrl Pts',(28.9380894768923,-9.10889026217819,15.3298017983529)) ;
#60264=CARTESIAN_POINT('Ctrl Pts',(28.9927894976113,-9.40788195803363,15.3585400322891)) ;
#60265=CARTESIAN_POINT('Ctrl Pts',(29.1568817385665,-10.3048570937892,15.4447695077162)) ;
#60266=CARTESIAN_POINT('Ctrl Pts',(29.2662662086701,-10.9028405664495,15.5022753819552)) ;
#60267=CARTESIAN_POINT('Ctrl Pts',(29.4837774821227,-12.0920123230926,15.6166613433893)) ;
#60268=CARTESIAN_POINT('Ctrl Pts',(29.5919042492133,-12.6832006071272,15.6735414989958)) ;
#60269=CARTESIAN_POINT('Ctrl Pts',(29.8081521853442,-13.8656062554755,15.7873251993035)) ;
#60270=CARTESIAN_POINT('Ctrl Pts',(29.9162144772883,-14.4565031966882,15.8441984291581)) ;
#60271=CARTESIAN_POINT('Ctrl Pts',(30.0223054640206,-15.0366437072152,15.9000442596779)) ;
#60272=CARTESIAN_POINT('Ctrl Pts',(30.0084212027096,-15.0366437072153,15.926232754655)) ;
#60273=CARTESIAN_POINT('Ctrl Pts',(30.0060125542796,-15.0234311859071,15.9249466590702)) ;
#60274=CARTESIAN_POINT('Ctrl Pts',(30.0036028909758,-15.0102130853827,15.9236600162224)) ;
#60275=CARTESIAN_POINT('Ctrl Pts',(29.8977542434076,-14.4295845145506,15.8671417561465)) ;
#60276=CARTESIAN_POINT('Ctrl Pts',(29.7924622066071,-13.8519867029534,15.8109107703475)) ;
#60277=CARTESIAN_POINT('Ctrl Pts',(29.5794117650166,-12.6832006073523,15.6971048239497)) ;
#60278=CARTESIAN_POINT('Ctrl Pts',(29.4716533429022,-12.0920123233512,15.6395298960295)) ;
#60279=CARTESIAN_POINT('Ctrl Pts',(29.2549128278598,-10.9028405667752,15.52369013004)) ;
#60280=CARTESIAN_POINT('Ctrl Pts',(29.145930698655,-10.3048570941488,15.4654253603752)) ;
#60281=CARTESIAN_POINT('Ctrl Pts',(28.982473067386,-9.40788195844391,15.3779988841212)) ;
#60282=CARTESIAN_POINT('Ctrl Pts',(28.9279898032311,-9.10889026260538,15.3488518039411)) ;
#60283=CARTESIAN_POINT('Ctrl Pts',(28.819184355446,-8.51175631084354,15.2906285814875)) ;
#60284=CARTESIAN_POINT('Ctrl Pts',(28.7648621676244,-8.21361405491334,15.2615524471178)) ;
#60285=CARTESIAN_POINT('Ctrl Pts',(28.6565350551247,-7.61902839129104,15.2035512786878)) ;
#60286=CARTESIAN_POINT('Ctrl Pts',(28.6025301214926,-7.32258498360224,15.1746262615182)) ;
#60287=CARTESIAN_POINT('Ctrl Pts',(28.4949942247213,-6.73224642569316,15.117006500543)) ;
#60288=CARTESIAN_POINT('Ctrl Pts',(28.4414632435045,-6.43835127543923,15.0883117908206)) ;
#60289=CARTESIAN_POINT('Ctrl Pts',(28.3616404604458,-6.00005680131941,15.0455005282547)) ;
#60290=CARTESIAN_POINT('Ctrl Pts',(28.3351118233974,-5.85438335299716,15.0312685576118)) ;
#60291=CARTESIAN_POINT('Ctrl Pts',(28.2822323150105,-5.5639920513746,15.0028909176579)) ;
#60292=CARTESIAN_POINT('Ctrl Pts',(28.2558814431192,-5.41927419807298,14.9887452493908)) ;
#60293=CARTESIAN_POINT('Ctrl Pts',(28.2033774709265,-5.13090026240829,14.9605493233015)) ;
#60294=CARTESIAN_POINT('Ctrl Pts',(28.1772243675642,-4.98724418004753,14.9464990712542)) ;
#60295=CARTESIAN_POINT('Ctrl Pts',(28.1251361712074,-4.70109996270815,14.9185026476569)) ;
#60296=CARTESIAN_POINT('Ctrl Pts',(28.0992010719645,-4.55861182771449,14.9045564878861)) ;
#60297=CARTESIAN_POINT('Ctrl Pts',(28.0475694932131,-4.27490968242578,14.8767762202746)) ;
#60298=CARTESIAN_POINT('Ctrl Pts',(28.0218730013745,-4.13369567304044,14.8629421360925)) ;
#60299=CARTESIAN_POINT('Ctrl Pts',(27.9707398824971,-3.85264795814086,14.8353927928548)) ;
#60300=CARTESIAN_POINT('Ctrl Pts',(27.9453032274214,-3.71281425254719,14.8216775866479)) ;
#60301=CARTESIAN_POINT('Ctrl Pts',(27.9073599757471,-3.50417855756733,14.8011972817496)) ;
#60302=CARTESIAN_POINT('Ctrl Pts',(27.8947475265083,-3.43481913663961,14.7943859067264)) ;
#60303=CARTESIAN_POINT('Ctrl Pts',(27.8695962549378,-3.29648518931778,14.7807940948554)) ;
#60304=CARTESIAN_POINT('Ctrl Pts',(27.8570574316513,-3.22751066292022,14.7740136598092)) ;
#60305=CARTESIAN_POINT('Ctrl Pts',(27.8320566915263,-3.08995977858624,14.7604833984031)) ;
#60306=CARTESIAN_POINT('Ctrl Pts',(27.8195947672391,-3.0213834206634,14.7537335860997)) ;
#60307=CARTESIAN_POINT('Ctrl Pts',(27.7947515317538,-2.88464214874115,14.7402634357714)) ;
#60308=CARTESIAN_POINT('Ctrl Pts',(27.7823702021659,-2.81647723466904,14.7335431324013)) ;
#60309=CARTESIAN_POINT('Ctrl Pts',(27.7587693018651,-2.68650146887413,14.7207145917589)) ;
#60310=CARTESIAN_POINT('Ctrl Pts',(27.7469473689554,-2.62137716522004,14.7142806541665)) ;
#60311=CARTESIAN_POINT('Ctrl Pts',(27.7288009900815,-2.52136502079237,14.7043835722678)) ;
#60312=CARTESIAN_POINT('Ctrl Pts',(27.7226832974612,-2.48764002458085,14.7010434901236)) ;
#60313=CARTESIAN_POINT('Ctrl Pts',(27.7103814461481,-2.41980246193246,14.6943177003912)) ;
#60314=CARTESIAN_POINT('Ctrl Pts',(27.7041972790692,-2.38568989545004,14.6909320086009)) ;
#60315=CARTESIAN_POINT('Ctrl Pts',(27.6918341987723,-2.31746485360458,14.6841507553881)) ;
#60316=CARTESIAN_POINT('Ctrl Pts',(27.685655267294,-2.28335239190624,14.6807552344374)) ;
#60317=CARTESIAN_POINT('Ctrl Pts',(27.6764452063594,-2.23247451914435,14.6756802271275)) ;
#60318=CARTESIAN_POINT('Ctrl Pts',(27.6733849172902,-2.21556369826045,14.6739915876559)) ;
#60319=CARTESIAN_POINT('Ctrl Pts',(27.6672930286196,-2.18188745273454,14.6706243426214)) ;
#60320=CARTESIAN_POINT('Ctrl Pts',(27.6642614279573,-2.16512202808461,14.6689457390569)) ;
#60321=CARTESIAN_POINT('Ctrl Pts',(27.6582363492046,-2.13178503271551,14.6656021523692)) ;
#60322=CARTESIAN_POINT('Ctrl Pts',(27.6552428635025,-2.11521346583559,14.6639371852972)) ;
#60323=CARTESIAN_POINT('Ctrl Pts',(27.6493038328078,-2.08231264738407,14.6606237335042)) ;
#60324=CARTESIAN_POINT('Ctrl Pts',(27.6463582651616,-2.06598339560755,14.6589752914224)) ;
#60325=CARTESIAN_POINT('Ctrl Pts',(27.6419838500786,-2.04170760017737,14.6565159721111)) ;
#60326=CARTESIAN_POINT('Ctrl Pts',(27.6405330465524,-2.03365201627149,14.6556984005285)) ;
#60327=CARTESIAN_POINT('Ctrl Pts',(27.637647614093,-2.01761960235524,14.6540674946091)) ;
#60328=CARTESIAN_POINT('Ctrl Pts',(27.6362129847709,-2.00964277234037,14.6532541610049)) ;
#60329=CARTESIAN_POINT('Ctrl Pts',(27.6333616654222,-1.99377392725156,14.65163107656)) ;
#60330=CARTESIAN_POINT('Ctrl Pts',(27.6319449619722,-1.98588191235219,14.6508213511158)) ;
#60331=CARTESIAN_POINT('Ctrl Pts',(27.6298350755515,-1.97411205169318,14.6496082241895)) ;
#60332=CARTESIAN_POINT('Ctrl Pts',(27.6291343137748,-1.97020012519214,14.649204081625)) ;
#60333=CARTESIAN_POINT('Ctrl Pts',(27.6277382520011,-1.96239975276553,14.6483958539812)) ;
#60334=CARTESIAN_POINT('Ctrl Pts',(27.6270429511546,-1.95851130682655,14.6479917704986)) ;
#60335=CARTESIAN_POINT('Ctrl Pts',(27.6256575021144,-1.95075390138752,14.647182481904)) ;
#60336=CARTESIAN_POINT('Ctrl Pts',(27.6249305344201,-1.94667883312135,14.6467557917342)) ;
#60337=CARTESIAN_POINT('Ctrl Pts',(27.6234449317041,-1.93833487564255,14.6458766296228)) ;
#60338=CARTESIAN_POINT('Ctrl Pts',(27.6226862623354,-1.93406598575086,14.6454242221669)) ;
#60339=CARTESIAN_POINT('Ctrl Pts',(27.6215521528282,-1.92766291383711,14.6447383810907)) ;
#60340=CARTESIAN_POINT('Ctrl Pts',(27.6211747756013,-1.92552861362188,14.6445085490605)) ;
#60341=CARTESIAN_POINT('Ctrl Pts',(27.6204262099871,-1.9212843810226,14.6440479625576)) ;
#60342=CARTESIAN_POINT('Ctrl Pts',(27.6200550047194,-1.91917444818244,14.6438172397235)) ;
#60343=CARTESIAN_POINT('Ctrl Pts',(27.6195068479476,-1.91604602467482,14.6434709306027)) ;
#60344=CARTESIAN_POINT('Ctrl Pts',(27.6193255770221,-1.91500929994461,14.6433554468457)) ;
#60345=CARTESIAN_POINT('Ctrl Pts',(27.6189667196087,-1.91295104701829,14.6431242343686)) ;
#60346=CARTESIAN_POINT('Ctrl Pts',(27.6187891319118,-1.91192951877891,14.6430085079098)) ;
#60347=CARTESIAN_POINT('Ctrl Pts',(27.6184386344892,-1.9099046964915,14.642776276223)) ;
#60348=CARTESIAN_POINT('Ctrl Pts',(27.6182657066978,-1.90890140427079,14.6426598058766)) ;
#60349=CARTESIAN_POINT('Ctrl Pts',(27.618010978076,-1.90741243382484,14.6424833498222)) ;
#60350=CARTESIAN_POINT('Ctrl Pts',(27.6179268504269,-1.90691877216053,14.6424242307122)) ;
#60351=CARTESIAN_POINT('Ctrl Pts',(27.6177605161466,-1.90593716098465,14.6423048892371)) ;
#60352=CARTESIAN_POINT('Ctrl Pts',(27.6176782980773,-1.90544921082332,14.6422446881598)) ;
#60353=CARTESIAN_POINT('Ctrl Pts',(27.6175557499485,-1.90471492798114,14.6421518770811)) ;
#60354=CARTESIAN_POINT('Ctrl Pts',(27.617512265948,-1.90445312340757,14.6421183899336)) ;
#60355=CARTESIAN_POINT('Ctrl Pts',(27.6174239851282,-1.90391724903068,14.6420484805282)) ;
#60356=CARTESIAN_POINT('Ctrl Pts',(27.6173791859132,-1.90364317904312,14.6420120627081)) ;
#60357=CARTESIAN_POINT('Ctrl Pts',(27.6172909153254,-1.90309535201991,14.6419368605644)) ;
#60358=CARTESIAN_POINT('Ctrl Pts',(27.6172474060307,-1.9028216338149,14.6418981649009)) ;
#60359=CARTESIAN_POINT('Ctrl Pts',(27.617091807557,-1.90163369931123,14.6416675448799)) ;
#60360=CARTESIAN_POINT('Ctrl Pts',(27.6170854309663,-1.90158501649411,14.6416580938266)) ;
#60361=CARTESIAN_POINT('Ctrl Pts',(27.6170790543757,-1.90153633367698,14.6416486427733)) ;
#60362=CARTESIAN_POINT('',(20.5712511819766,-15.0366437072153,27.0365282098628)) ;
#60363=CARTESIAN_POINT('',(20.5476539041778,-15.0366437072153,27.0544663940874)) ;
#60364=CARTESIAN_POINT('Origin',(-0.82663321391253,-21.6462763158694,-1.08741739643852)) ;
#60365=CARTESIAN_POINT('',(18.916713407666,-1.90153624425509,24.8845109088162)) ;
#60366=CARTESIAN_POINT('Ctrl Pts',(18.9167134194622,-1.90153633693974,24.8845109239092)) ;
#60367=CARTESIAN_POINT('Ctrl Pts',(18.9167246001933,-1.90158489749522,24.8845150304531)) ;
#60368=CARTESIAN_POINT('Ctrl Pts',(18.9169173960229,-1.90242225530982,24.8845858419702)) ;
#60369=CARTESIAN_POINT('Ctrl Pts',(18.9169872501015,-1.90282386080039,24.8846369937121)) ;
#60370=CARTESIAN_POINT('Ctrl Pts',(18.9170325447247,-1.90309805778379,24.8846737408821)) ;
#60371=CARTESIAN_POINT('Ctrl Pts',(18.9171211741336,-1.90364684244124,24.8847488264717)) ;
#60372=CARTESIAN_POINT('Ctrl Pts',(18.917164427513,-1.90392139127148,24.8847872166913)) ;
#60373=CARTESIAN_POINT('Ctrl Pts',(18.9172478295099,-1.90445820158809,24.8848631676174)) ;
#60374=CARTESIAN_POINT('Ctrl Pts',(18.9172879740443,-1.90472046326274,24.8849007314765)) ;
#60375=CARTESIAN_POINT('Ctrl Pts',(18.9173995679819,-1.90545604096936,24.8850068498011)) ;
#60376=CARTESIAN_POINT('Ctrl Pts',(18.9174723960696,-1.90594485602389,24.8850783796347)) ;
#60377=CARTESIAN_POINT('Ctrl Pts',(18.917617312545,-1.9069282070596,24.8852234867119)) ;
#60378=CARTESIAN_POINT('Ctrl Pts',(18.9176893817405,-1.90742274369117,24.8852970787139)) ;
#60379=CARTESIAN_POINT('Ctrl Pts',(18.9179050798507,-1.90891435313948,24.8855203186311)) ;
#60380=CARTESIAN_POINT('Ctrl Pts',(18.9180482304223,-1.90991942349788,24.8856724062683)) ;
#60381=CARTESIAN_POINT('Ctrl Pts',(18.9183345848843,-1.91194783429415,24.8859812837709)) ;
#60382=CARTESIAN_POINT('Ctrl Pts',(18.9184777572423,-1.91297117290453,24.8861380971322)) ;
#60383=CARTESIAN_POINT('Ctrl Pts',(18.9187644623475,-1.91503307343387,24.8864554017379)) ;
#60384=CARTESIAN_POINT('Ctrl Pts',(18.9189079930907,-1.91607163539539,24.8866158945166)) ;
#60385=CARTESIAN_POINT('Ctrl Pts',(18.9193391502031,-1.91920560283358,24.8871016891789)) ;
#60386=CARTESIAN_POINT('Ctrl Pts',(18.9196273767154,-1.92131927460614,24.8874312766233)) ;
#60387=CARTESIAN_POINT('Ctrl Pts',(18.9202039805437,-1.92557102804893,24.8880966734798)) ;
#60388=CARTESIAN_POINT('Ctrl Pts',(18.9204923293024,-1.92770911017595,24.8884325047192)) ;
#60389=CARTESIAN_POINT('Ctrl Pts',(18.9213540857366,-1.93412352783167,24.8894425437714)) ;
#60390=CARTESIAN_POINT('Ctrl Pts',(18.9219242497512,-1.9383999815575,24.8901192480343)) ;
#60391=CARTESIAN_POINT('Ctrl Pts',(18.9230340800967,-1.94675872290243,24.8914454363964)) ;
#60392=CARTESIAN_POINT('Ctrl Pts',(18.9235736882947,-1.95084101120065,24.8920949648635)) ;
#60393=CARTESIAN_POINT('Ctrl Pts',(18.9245982302545,-1.95861222317853,24.893333470053)) ;
#60394=CARTESIAN_POINT('Ctrl Pts',(18.9251103696797,-1.96250762108956,24.8939553645543)) ;
#60395=CARTESIAN_POINT('Ctrl Pts',(18.926135595151,-1.97032193942165,24.8952045402017)) ;
#60396=CARTESIAN_POINT('Ctrl Pts',(18.9266486797592,-1.97424085985611,24.8958318224441)) ;
#60397=CARTESIAN_POINT('Ctrl Pts',(18.928189858839,-1.98603176322635,24.8977210686261)) ;
#60398=CARTESIAN_POINT('Ctrl Pts',(18.9292199162513,-1.99393788781487,24.8989904032649)) ;
#60399=CARTESIAN_POINT('Ctrl Pts',(18.9312865299045,-2.00983510388289,24.9015461889568)) ;
#60400=CARTESIAN_POINT('Ctrl Pts',(18.9323230632391,-2.01782619518781,24.9028326573775)) ;
#60401=CARTESIAN_POINT('Ctrl Pts',(18.9344029442502,-2.03388727245648,24.9054208944857)) ;
#60402=CARTESIAN_POINT('Ctrl Pts',(18.9354462912739,-2.04195725842473,24.9067226636703)) ;
#60403=CARTESIAN_POINT('Ctrl Pts',(18.9385864310043,-2.06627645495748,24.9106486518594)) ;
#60404=CARTESIAN_POINT('Ctrl Pts',(18.9406934032119,-2.08263490068957,24.9132934891451)) ;
#60405=CARTESIAN_POINT('Ctrl Pts',(18.9449314942448,-2.11559454019749,24.9186278233006)) ;
#60406=CARTESIAN_POINT('Ctrl Pts',(18.9470625746199,-2.13219573417824,24.9213173494524)) ;
#60407=CARTESIAN_POINT('Ctrl Pts',(18.9513444123465,-2.16559233026566,24.9267318585154)) ;
#60408=CARTESIAN_POINT('Ctrl Pts',(18.9534951550791,-2.18238772853293,24.9294568515428)) ;
#60409=CARTESIAN_POINT('Ctrl Pts',(18.9578112165814,-2.21612418118078,24.9349335682933)) ;
#60410=CARTESIAN_POINT('Ctrl Pts',(18.9599765335518,-2.23306523556928,24.9376852933859)) ;
#60411=CARTESIAN_POINT('Ctrl Pts',(18.9664862051206,-2.28403406873264,24.9459678532064)) ;
#60412=CARTESIAN_POINT('Ctrl Pts',(18.970844338311,-2.31820751721538,24.9515260283606)) ;
#60413=CARTESIAN_POINT('Ctrl Pts',(18.9795517811882,-2.38655453263177,24.9626491168712)) ;
#60414=CARTESIAN_POINT('Ctrl Pts',(18.9839010538543,-2.42072808590034,24.9682140548224)) ;
#60415=CARTESIAN_POINT('Ctrl Pts',(18.9925437571043,-2.48868692909063,24.9792855908494)) ;
#60416=CARTESIAN_POINT('Ctrl Pts',(18.9968371734376,-2.52247221905787,24.98479219977)) ;
#60417=CARTESIAN_POINT('Ctrl Pts',(19.0095621717323,-2.62266316565928,25.0011276406879)) ;
#60418=CARTESIAN_POINT('Ctrl Pts',(19.0178385952872,-2.68790389863798,25.0117720165858)) ;
#60419=CARTESIAN_POINT('Ctrl Pts',(19.03434711155,-2.81812392918961,25.0330266013669)) ;
#60420=CARTESIAN_POINT('Ctrl Pts',(19.0429988126584,-2.88642263976059,25.0441795241338)) ;
#60421=CARTESIAN_POINT('Ctrl Pts',(19.0603444951684,-3.02343231225636,25.0665602460336)) ;
#60422=CARTESIAN_POINT('Ctrl Pts',(19.0690384453017,-3.09214327425391,25.0777880689548)) ;
#60423=CARTESIAN_POINT('Ctrl Pts',(19.0864691080612,-3.22996414826103,25.100314771687)) ;
#60424=CARTESIAN_POINT('Ctrl Pts',(19.0952058080039,-3.29907406025701,25.111613661136)) ;
#60425=CARTESIAN_POINT('Ctrl Pts',(19.1127217414322,-3.43767953424804,25.134279218396)) ;
#60426=CARTESIAN_POINT('Ctrl Pts',(19.1215009732858,-3.50717509624653,25.1456458874472)) ;
#60427=CARTESIAN_POINT('Ctrl Pts',(19.1479015029145,-3.71622030857066,25.179843118157)) ;
#60428=CARTESIAN_POINT('Ctrl Pts',(19.1655857217907,-3.85632848456949,25.2027708370381)) ;
#60429=CARTESIAN_POINT('Ctrl Pts',(19.2011138810135,-4.13792784955716,25.2488638763194)) ;
#60430=CARTESIAN_POINT('Ctrl Pts',(19.2189577736851,-4.27941903862544,25.2720292329816)) ;
#60431=CARTESIAN_POINT('Ctrl Pts',(19.2547950843996,-4.56367804415205,25.3185776818844)) ;
#60432=CARTESIAN_POINT('Ctrl Pts',(19.27278848106,-4.70644585970026,25.3419607901433)) ;
#60433=CARTESIAN_POINT('Ctrl Pts',(19.3089135538598,-4.99315173061398,25.3889256738188)) ;
#60434=CARTESIAN_POINT('Ctrl Pts',(19.3270452193696,-5.13708978599453,25.4125074573199)) ;
#60435=CARTESIAN_POINT('Ctrl Pts',(19.3634349644308,-5.42602975175821,25.4598510947412)) ;
#60436=CARTESIAN_POINT('Ctrl Pts',(19.3816930387743,-5.57103166213904,25.4836129526197)) ;
#60437=CARTESIAN_POINT('Ctrl Pts',(19.4183233423265,-5.86199295357377,25.5312984414969)) ;
#60438=CARTESIAN_POINT('Ctrl Pts',(19.4366955705936,-6.007952334629,25.5552220732107)) ;
#60439=CARTESIAN_POINT('Ctrl Pts',(19.491964714102,-6.44710710781996,25.6272084747515)) ;
#60440=CARTESIAN_POINT('Ctrl Pts',(19.5290141484514,-6.74157912528294,25.6754867038415)) ;
#60441=CARTESIAN_POINT('Ctrl Pts',(19.6034176105111,-7.3330764193532,25.7724744209222)) ;
#60442=CARTESIAN_POINT('Ctrl Pts',(19.6407716074773,-7.63010169599417,25.8211839322927)) ;
#60443=CARTESIAN_POINT('Ctrl Pts',(19.7156804754865,-8.22585443201747,25.9188921269566)) ;
#60444=CARTESIAN_POINT('Ctrl Pts',(19.7532353312954,-8.52458189139653,25.9678908218298)) ;
#60445=CARTESIAN_POINT('Ctrl Pts',(19.8284413201389,-9.12288791730656,26.0660359638418)) ;
#60446=CARTESIAN_POINT('Ctrl Pts',(19.8660924460453,-9.42246648384445,26.1151824164005)) ;
#60447=CARTESIAN_POINT('Ctrl Pts',(19.9790325106291,-10.321202231654,26.2626319069737)) ;
#60448=CARTESIAN_POINT('Ctrl Pts',(20.0543082599602,-10.9203594456895,26.3609449797701)) ;
#60449=CARTESIAN_POINT('Ctrl Pts',(20.2039793991902,-12.1118653471233,26.5564729205436)) ;
#60450=CARTESIAN_POINT('Ctrl Pts',(20.2783747273927,-12.7042140345733,26.6536878354332)) ;
#60451=CARTESIAN_POINT('Ctrl Pts',(20.4260447461218,-13.880135442222,26.8466913840078)) ;
#60452=CARTESIAN_POINT('Ctrl Pts',(20.4993050558587,-14.4635951119166,26.9424616027179)) ;
#60453=CARTESIAN_POINT('Ctrl Pts',(20.5712511819835,-15.0366437072153,27.0365282098576)) ;
#60454=CARTESIAN_POINT('Ctrl Pts',(20.5476539041697,-15.0366437072153,27.0544663940936)) ;
#60455=CARTESIAN_POINT('Ctrl Pts',(20.5470684975163,-15.0319446558128,27.0536915741554)) ;
#60456=CARTESIAN_POINT('Ctrl Pts',(20.5464830041271,-15.0272449043538,27.0529166384232)) ;
#60457=CARTESIAN_POINT('Ctrl Pts',(20.4750716273534,-14.454025800044,26.9583992626796)) ;
#60458=CARTESIAN_POINT('Ctrl Pts',(20.4029804926787,-13.8752942608754,26.8629676433982)) ;
#60459=CARTESIAN_POINT('Ctrl Pts',(20.2571208155035,-12.7042140341984,26.6698446391085)) ;
#60460=CARTESIAN_POINT('Ctrl Pts',(20.1833522435298,-12.1118653466928,26.572153276506)) ;
#60461=CARTESIAN_POINT('Ctrl Pts',(20.0349925688502,-10.920359445147,26.375628386271)) ;
#60462=CARTESIAN_POINT('Ctrl Pts',(19.9604014044365,-10.3212022310552,26.2767949055354)) ;
#60463=CARTESIAN_POINT('Ctrl Pts',(19.8485411167186,-9.42246648316126,26.1285245899066)) ;
#60464=CARTESIAN_POINT('Ctrl Pts',(19.8112587958758,-9.12288791659522,26.07909777902)) ;
#60465=CARTESIAN_POINT('Ctrl Pts',(19.7368107782602,-8.52458189062898,25.980376442246)) ;
#60466=CARTESIAN_POINT('Ctrl Pts',(19.6996450743571,-8.22585443122183,25.9310819217775)) ;
#60467=CARTESIAN_POINT('Ctrl Pts',(19.6255385891123,-7.63010169514257,25.8327637715793)) ;
#60468=CARTESIAN_POINT('Ctrl Pts',(19.5885977925355,-7.3330764184737,25.7837401534318)) ;
#60469=CARTESIAN_POINT('Ctrl Pts',(19.5150503130468,-6.74157912434787,25.6861017353031)) ;
#60470=CARTESIAN_POINT('Ctrl Pts',(19.4784435993818,-6.44710710685725,25.6374869586913)) ;
#60471=CARTESIAN_POINT('Ctrl Pts',(19.4238671648451,-6.00795233362499,25.5649739734696)) ;
#60472=CARTESIAN_POINT('Ctrl Pts',(19.4057306413877,-5.86199295255608,25.5408711636141)) ;
#60473=CARTESIAN_POINT('Ctrl Pts',(19.3695829331826,-5.57103166109401,25.4928188152847)) ;
#60474=CARTESIAN_POINT('Ctrl Pts',(19.3515717474928,-5.42602975069957,25.4688692775275)) ;
#60475=CARTESIAN_POINT('Ctrl Pts',(19.3156890740419,-5.13708978490872,25.4211401742822)) ;
#60476=CARTESIAN_POINT('Ctrl Pts',(19.2978175810733,-4.99315172951466,25.3973606127537)) ;
#60477=CARTESIAN_POINT('Ctrl Pts',(19.2622290484611,-4.70644585857401,25.3499878618243)) ;
#60478=CARTESIAN_POINT('Ctrl Pts',(19.2445119981902,-4.56367804301236,25.3263946804981)) ;
#60479=CARTESIAN_POINT('Ctrl Pts',(19.2092477367877,-4.27941903745906,25.2794106108267)) ;
#60480=CARTESIAN_POINT('Ctrl Pts',(19.1917005045017,-4.13792784837747,25.2560197387988)) ;
#60481=CARTESIAN_POINT('Ctrl Pts',(19.1567923462519,-3.85632848336334,25.2094553870243)) ;
#60482=CARTESIAN_POINT('Ctrl Pts',(19.139431372585,-3.71622030735133,25.1862819435199)) ;
#60483=CARTESIAN_POINT('Ctrl Pts',(19.1135435210161,-3.50717509500758,25.1516949850762)) ;
#60484=CARTESIAN_POINT('Ctrl Pts',(19.1049398604539,-3.43767953300257,25.1401948501975)) ;
#60485=CARTESIAN_POINT('Ctrl Pts',(19.0877864714919,-3.29907405899852,25.1172536937959)) ;
#60486=CARTESIAN_POINT('Ctrl Pts',(19.0792367414662,-3.22996414699606,25.1058126735094)) ;
#60487=CARTESIAN_POINT('Ctrl Pts',(19.062194333463,-3.09214327297596,25.0829908271812)) ;
#60488=CARTESIAN_POINT('Ctrl Pts',(19.0537016428067,-3.02343231097198,25.0716100107814)) ;
#60489=CARTESIAN_POINT('Ctrl Pts',(19.0367771600085,-2.88642263846334,25.0489091011817)) ;
#60490=CARTESIAN_POINT('Ctrl Pts',(19.0283453365751,-2.81812392788592,25.03758903175)) ;
#60491=CARTESIAN_POINT('Ctrl Pts',(19.0122819774909,-2.68790389729668,25.0159960472697)) ;
#60492=CARTESIAN_POINT('Ctrl Pts',(19.0042397670059,-2.62266316428518,25.0051736272164)) ;
#60493=CARTESIAN_POINT('Ctrl Pts',(18.9919040506772,-2.52247221763345,24.9885422618283)) ;
#60494=CARTESIAN_POINT('Ctrl Pts',(18.9877467682398,-2.48868692764926,24.9829321666061)) ;
#60495=CARTESIAN_POINT('Ctrl Pts',(18.9793909578204,-2.42072808442481,24.9716425403104)) ;
#60496=CARTESIAN_POINT('Ctrl Pts',(18.975192415586,-2.38655453113906,24.9659630200594)) ;
#60497=CARTESIAN_POINT('Ctrl Pts',(18.966804251457,-2.31820751568836,24.9545972221456)) ;
#60498=CARTESIAN_POINT('Ctrl Pts',(18.9626145959631,-2.28403406718845,24.9489109735716)) ;
#60499=CARTESIAN_POINT('Ctrl Pts',(18.9563754571263,-2.23306523399947,24.9404227601082)) ;
#60500=CARTESIAN_POINT('Ctrl Pts',(18.9543033160809,-2.21612417960246,24.9376002045167)) ;
#60501=CARTESIAN_POINT('Ctrl Pts',(18.9501808944577,-2.18238772693766,24.9319762865525)) ;
#60502=CARTESIAN_POINT('Ctrl Pts',(18.9481306120741,-2.16559232866193,24.9291749255512)) ;
#60503=CARTESIAN_POINT('Ctrl Pts',(18.944058974838,-2.13219573255776,24.9236006262252)) ;
#60504=CARTESIAN_POINT('Ctrl Pts',(18.9420376063183,-2.11559453856861,24.9208276992869)) ;
#60505=CARTESIAN_POINT('Ctrl Pts',(18.9380315181337,-2.08263489904415,24.915317001147)) ;
#60506=CARTESIAN_POINT('Ctrl Pts',(18.9360467599696,-2.06627645330387,24.9125792591586)) ;
#60507=CARTESIAN_POINT('Ctrl Pts',(18.9331039504433,-2.04195725675893,24.908503264445)) ;
#60508=CARTESIAN_POINT('Ctrl Pts',(18.9321287556484,-2.03388727078661,24.9071496872821)) ;
#60509=CARTESIAN_POINT('Ctrl Pts',(18.9301912869132,-2.01782619350988,24.904453191174)) ;
#60510=CARTESIAN_POINT('Ctrl Pts',(18.9292290123289,-2.00983510220101,24.9031102727181)) ;
#60511=CARTESIAN_POINT('Ctrl Pts',(18.9273192627605,-1.99393788612502,24.9004352420469)) ;
#60512=CARTESIAN_POINT('Ctrl Pts',(18.9263717649069,-1.98603176153238,24.8991031472622)) ;
#60513=CARTESIAN_POINT('Ctrl Pts',(18.9249636908405,-1.97424085815624,24.897112717278)) ;
#60514=CARTESIAN_POINT('Ctrl Pts',(18.9244965377394,-1.97032193772004,24.8964505188111)) ;
#60515=CARTESIAN_POINT('Ctrl Pts',(18.9235671714202,-1.96250761938401,24.8951284729298)) ;
#60516=CARTESIAN_POINT('Ctrl Pts',(18.9231049567604,-1.9586122214708,24.894468626608)) ;
#60517=CARTESIAN_POINT('Ctrl Pts',(18.9221856891252,-1.95084100968508,24.8931500940073)) ;
#60518=CARTESIAN_POINT('Ctrl Pts',(18.9217041964974,-1.94675872159085,24.8924563872854)) ;
#60519=CARTESIAN_POINT('Ctrl Pts',(18.9207232588284,-1.93839998066323,24.8910322173662)) ;
#60520=CARTESIAN_POINT('Ctrl Pts',(18.9202237554944,-1.93412352715089,24.8903017983059)) ;
#60521=CARTESIAN_POINT('Ctrl Pts',(18.9194810766782,-1.9277091098154,24.8892012388849)) ;
#60522=CARTESIAN_POINT('Ctrl Pts',(18.91923462799,-1.92557102779551,24.8888335560678)) ;
#60523=CARTESIAN_POINT('Ctrl Pts',(18.9187477427387,-1.92131927456496,24.8880999569773)) ;
#60524=CARTESIAN_POINT('Ctrl Pts',(18.9185072775343,-1.91920560289798,24.8877340623579)) ;
#60525=CARTESIAN_POINT('Ctrl Pts',(18.9181545368557,-1.91607163561626,24.8871886571131)) ;
#60526=CARTESIAN_POINT('Ctrl Pts',(18.9180382925426,-1.91503307370567,24.8870074217427)) ;
#60527=CARTESIAN_POINT('Ctrl Pts',(18.9178092554453,-1.91297117327927,24.8866462790838)) ;
#60528=CARTESIAN_POINT('Ctrl Pts',(18.9176964606399,-1.9119478347208,24.8864663733209)) ;
#60529=CARTESIAN_POINT('Ctrl Pts',(18.9174754496683,-1.90991942402579,24.8861078230146)) ;
#60530=CARTESIAN_POINT('Ctrl Pts',(18.917367202443,-1.90891435371686,24.8859292025562)) ;
#60531=CARTESIAN_POINT('Ctrl Pts',(18.9172098049877,-1.90742274434305,24.8856616436526)) ;
#60532=CARTESIAN_POINT('Ctrl Pts',(18.9171581759787,-1.90692820773646,24.8855725134313)) ;
#60533=CARTESIAN_POINT('Ctrl Pts',(18.9170571273222,-1.90594485674973,24.8853940589178)) ;
#60534=CARTESIAN_POINT('Ctrl Pts',(18.9170076883461,-1.90545604172008,24.8853047491503)) ;
#60535=CARTESIAN_POINT('Ctrl Pts',(18.9169352925858,-1.90472046411337,24.885168833172)) ;
#60536=CARTESIAN_POINT('Ctrl Pts',(18.9169098377483,-1.90445820251875,24.8851201025163)) ;
#60537=CARTESIAN_POINT('Ctrl Pts',(18.9168589676523,-1.90392139236518,24.8850194215245)) ;
#60538=CARTESIAN_POINT('Ctrl Pts',(18.9168335483687,-1.90364684362271,24.8849674742005)) ;
#60539=CARTESIAN_POINT('Ctrl Pts',(18.9167849105521,-1.90309805913159,24.8848619878359)) ;
#60540=CARTESIAN_POINT('Ctrl Pts',(18.9167616202308,-1.90282386221791,24.8848085134487)) ;
#60541=CARTESIAN_POINT('Ctrl Pts',(18.9167170645518,-1.90163370354021,24.8845334285406)) ;
#60542=CARTESIAN_POINT('Ctrl Pts',(18.916715242007,-1.90158502023998,24.8845221762249)) ;
#60543=CARTESIAN_POINT('Ctrl Pts',(18.9167134194622,-1.90153633693974,24.8845109239092)) ;
#60544=CARTESIAN_POINT('',(7.31761838529024,-15.0366437072153,33.1753326132827)) ;
#60545=CARTESIAN_POINT('',(7.28867002793266,-15.0366437072153,33.181704628584)) ;
#60546=CARTESIAN_POINT('Origin',(-0.293637272419033,-21.6462763158694,-1.3340075774398)) ;
#60547=CARTESIAN_POINT('',(6.71960918123862,-1.90153624278853,30.5274922283378)) ;
#60548=CARTESIAN_POINT('Ctrl Pts',(6.7196091855373,-1.90153633400663,30.527492246694)) ;
#60549=CARTESIAN_POINT('Ctrl Pts',(6.71961763099485,-1.90158489163453,30.5275006628107)) ;
#60550=CARTESIAN_POINT('Ctrl Pts',(6.71976214984686,-1.90241581081184,30.5276446795811)) ;
#60551=CARTESIAN_POINT('Ctrl Pts',(6.7198038475356,-1.90281444934172,30.5277198556706)) ;
#60552=CARTESIAN_POINT('Ctrl Pts',(6.71982938587613,-1.90308662225266,30.5277718277734)) ;
#60553=CARTESIAN_POINT('Ctrl Pts',(6.71987802505912,-1.90363135851574,30.5278763911327)) ;
#60554=CARTESIAN_POINT('Ctrl Pts',(6.71990103052572,-1.90390388306625,30.5279289951723)) ;
#60555=CARTESIAN_POINT('Ctrl Pts',(6.71994458342815,-1.90443673670834,30.5280321636685)) ;
#60556=CARTESIAN_POINT('Ctrl Pts',(6.71996512589195,-1.90469706598677,30.5280827292591)) ;
#60557=CARTESIAN_POINT('Ctrl Pts',(6.72002151385849,-1.90542716873087,30.5282248117068)) ;
#60558=CARTESIAN_POINT('Ctrl Pts',(6.72005735925489,-1.90591232651548,30.528319584007)) ;
#60559=CARTESIAN_POINT('Ctrl Pts',(6.72012752404694,-1.90688832041617,30.5285106660766)) ;
#60560=CARTESIAN_POINT('Ctrl Pts',(6.72016181990902,-1.90737915718282,30.5286069811638)) ;
#60561=CARTESIAN_POINT('Ctrl Pts',(6.72026321513444,-1.90885960740112,30.528897935056)) ;
#60562=CARTESIAN_POINT('Ctrl Pts',(6.72032886026737,-1.90985715876355,30.5290945736736)) ;
#60563=CARTESIAN_POINT('Ctrl Pts',(6.72045822892328,-1.91187039526605,30.5294921111097)) ;
#60564=CARTESIAN_POINT('Ctrl Pts',(6.72052191412236,-1.91288607857933,30.5296930179773)) ;
#60565=CARTESIAN_POINT('Ctrl Pts',(6.72064806943539,-1.91493255493047,30.5300982964868)) ;
#60566=CARTESIAN_POINT('Ctrl Pts',(6.72071053707861,-1.91596334801114,30.5303026686815)) ;
#60567=CARTESIAN_POINT('Ctrl Pts',(6.72089664234593,-1.91907387250008,30.5309199105522)) ;
#60568=CARTESIAN_POINT('Ctrl Pts',(6.72101902700158,-1.92117173390307,30.5313368924495)) ;
#60569=CARTESIAN_POINT('Ctrl Pts',(6.72126132588643,-1.92539168486392,30.5321765268574)) ;
#60570=CARTESIAN_POINT('Ctrl Pts',(6.72138120521115,-1.92751377487788,30.5325991871476)) ;
#60571=CARTESIAN_POINT('Ctrl Pts',(6.72173680403374,-1.93388021616538,30.5338680933395)) ;
#60572=CARTESIAN_POINT('Ctrl Pts',(6.72196854648776,-1.93812468561987,30.5347152396626)) ;
#60573=CARTESIAN_POINT('Ctrl Pts',(6.7224158750982,-1.94642091221635,30.5363723094294)) ;
#60574=CARTESIAN_POINT('Ctrl Pts',(6.72263139013284,-1.95047267003741,30.5371822486719)) ;
#60575=CARTESIAN_POINT('Ctrl Pts',(6.72303836615672,-1.95818550039066,30.5387247503642)) ;
#60576=CARTESIAN_POINT('Ctrl Pts',(6.72324062169856,-1.96205150175638,30.5394983009961)) ;
#60577=CARTESIAN_POINT('Ctrl Pts',(6.72364373171298,-1.96980684956421,30.541050650625)) ;
#60578=CARTESIAN_POINT('Ctrl Pts',(6.72384458442883,-1.97369619601971,30.5418294500114)) ;
#60579=CARTESIAN_POINT('Ctrl Pts',(6.72444578258132,-1.98539811988876,30.5441733177044)) ;
#60580=CARTESIAN_POINT('Ctrl Pts',(6.72484481411897,-1.99324458139089,30.5457458453102)) ;
#60581=CARTESIAN_POINT('Ctrl Pts',(6.72564157932198,-2.00902183023835,30.5489090300892)) ;
#60582=CARTESIAN_POINT('Ctrl Pts',(6.72603928501628,-2.01695261740918,30.5504996933823)) ;
#60583=CARTESIAN_POINT('Ctrl Pts',(6.72683444436499,-2.03289249115159,30.5536976440974)) ;
#60584=CARTESIAN_POINT('Ctrl Pts',(6.72723189722214,-2.04090157772765,30.5553049316954)) ;
#60585=CARTESIAN_POINT('Ctrl Pts',(6.72842471757584,-2.06503725187992,30.5601496340252)) ;
#60586=CARTESIAN_POINT('Ctrl Pts',(6.72922064600262,-2.08127225042057,30.5634098657348)) ;
#60587=CARTESIAN_POINT('Ctrl Pts',(6.73081561318064,-2.11398316398243,30.5699806239775)) ;
#60588=CARTESIAN_POINT('Ctrl Pts',(6.73161460493413,-2.13045907920851,30.5732911608989)) ;
#60589=CARTESIAN_POINT('Ctrl Pts',(6.73321551517985,-2.16360365253471,30.579952376134)) ;
#60590=CARTESIAN_POINT('Ctrl Pts',(6.73401741622393,-2.180272306796,30.5833030574759)) ;
#60591=CARTESIAN_POINT('Ctrl Pts',(6.73562319127244,-2.21375417249349,30.5900345750952)) ;
#60592=CARTESIAN_POINT('Ctrl Pts',(6.73642706307232,-2.23056738393757,30.593415411859)) ;
#60593=CARTESIAN_POINT('Ctrl Pts',(6.73883960451742,-2.28115158932819,30.6035883104669)) ;
#60594=CARTESIAN_POINT('Ctrl Pts',(6.74044927101791,-2.31506715404313,30.6104107449792)) ;
#60595=CARTESIAN_POINT('Ctrl Pts',(6.7436578074868,-2.38289840191499,30.6240580155635)) ;
#60596=CARTESIAN_POINT('Ctrl Pts',(6.7452566337006,-2.41681407140828,30.6308828583751)) ;
#60597=CARTESIAN_POINT('Ctrl Pts',(6.74842826526026,-2.48426007754026,30.6444567327451)) ;
#60598=CARTESIAN_POINT('Ctrl Pts',(6.75000105319838,-2.51779041422449,30.6512057681449)) ;
#60599=CARTESIAN_POINT('Ctrl Pts',(6.75465637156452,-2.61722529246259,30.6712221068618)) ;
#60600=CARTESIAN_POINT('Ctrl Pts',(6.75767596939282,-2.68197370184678,30.6842586177816)) ;
#60601=CARTESIAN_POINT('Ctrl Pts',(6.76368709728244,-2.81116116814065,30.7102723568555)) ;
#60602=CARTESIAN_POINT('Ctrl Pts',(6.76683044475462,-2.87889443254617,30.7239132426992)) ;
#60603=CARTESIAN_POINT('Ctrl Pts',(6.77312397740687,-3.01476979976207,30.7512800220962)) ;
#60604=CARTESIAN_POINT('Ctrl Pts',(6.77627412448397,-3.08291190264499,30.7650059240521)) ;
#60605=CARTESIAN_POINT('Ctrl Pts',(6.7825832881807,-3.21959175557408,30.7925394970826)) ;
#60606=CARTESIAN_POINT('Ctrl Pts',(6.7857422893433,-3.28812950560671,30.8063471715564)) ;
#60607=CARTESIAN_POINT('Ctrl Pts',(6.79207032559441,-3.42558746291981,30.8340412422536)) ;
#60608=CARTESIAN_POINT('Ctrl Pts',(6.79523935870023,-3.49450767020372,30.8479276389131)) ;
#60609=CARTESIAN_POINT('Ctrl Pts',(6.80476249563476,-3.70182219440112,30.8897005080007)) ;
#60610=CARTESIAN_POINT('Ctrl Pts',(6.81113274335611,-3.84077041300617,30.9177006360046)) ;
#60611=CARTESIAN_POINT('Ctrl Pts',(6.82391799489518,-4.1200384133498,30.973981271921)) ;
#60612=CARTESIAN_POINT('Ctrl Pts',(6.83033294053835,-4.26035819516773,31.0022617926555)) ;
#60613=CARTESIAN_POINT('Ctrl Pts',(6.84320669650211,-4.54226381709422,31.0590810847542)) ;
#60614=CARTESIAN_POINT('Ctrl Pts',(6.84966548083055,-4.68384965629434,31.0876198616476)) ;
#60615=CARTESIAN_POINT('Ctrl Pts',(6.86262474154796,-4.96818188617416,31.1449338183818)) ;
#60616=CARTESIAN_POINT('Ctrl Pts',(6.86912520496441,-5.1109282768689,31.1737090010814)) ;
#60617=CARTESIAN_POINT('Ctrl Pts',(6.88216489466588,-5.39747610568063,31.2314740888635)) ;
#60618=CARTESIAN_POINT('Ctrl Pts',(6.88870411459209,-5.54127754379532,31.2604639953449)) ;
#60619=CARTESIAN_POINT('Ctrl Pts',(6.90181790733773,-5.82982996387431,31.3186369560578)) ;
#60620=CARTESIAN_POINT('Ctrl Pts',(6.90839247900822,-5.97458094583994,31.3478200105417)) ;
#60621=CARTESIAN_POINT('Ctrl Pts',(6.92816363850333,-6.41009995266176,31.435626637206)) ;
#60622=CARTESIAN_POINT('Ctrl Pts',(6.94140774507523,-6.70213403375071,31.494507655259)) ;
#60623=CARTESIAN_POINT('Ctrl Pts',(6.96799044907206,-7.28873431687813,31.6127847052307)) ;
#60624=CARTESIAN_POINT('Ctrl Pts',(6.98132900895718,-7.58330051895022,31.6721807454196)) ;
#60625=CARTESIAN_POINT('Ctrl Pts',(7.00806644621525,-8.17412101370043,31.7913167596082)) ;
#60626=CARTESIAN_POINT('Ctrl Pts',(7.02146530498564,-8.47037530637525,31.8510567377018)) ;
#60627=CARTESIAN_POINT('Ctrl Pts',(7.0482880948497,-9.06372795280004,31.9707097837378)) ;
#60628=CARTESIAN_POINT('Ctrl Pts',(7.06171201723382,-9.36082630655692,32.0306228535982)) ;
#60629=CARTESIAN_POINT('Ctrl Pts',(7.10196750689891,-10.2521214159956,32.2103656563209)) ;
#60630=CARTESIAN_POINT('Ctrl Pts',(7.12878294951035,-10.8463182044253,32.3301989454179)) ;
#60631=CARTESIAN_POINT('Ctrl Pts',(7.18207860074687,-12.0279596230766,32.5685105146323)) ;
#60632=CARTESIAN_POINT('Ctrl Pts',(7.20855873401127,-12.6154042533499,32.6869888113477)) ;
#60633=CARTESIAN_POINT('Ctrl Pts',(7.26088782347813,-13.7767891024697,32.9212267181271)) ;
#60634=CARTESIAN_POINT('Ctrl Pts',(7.28673674368023,-14.3507293213134,33.0369863361147)) ;
#60635=CARTESIAN_POINT('Ctrl Pts',(7.31395599106871,-14.9552953856141,33.1589249456923)) ;
#60636=CARTESIAN_POINT('Ctrl Pts',(7.31578843034751,-14.9959966435745,33.1671342399967)) ;
#60637=CARTESIAN_POINT('Ctrl Pts',(7.31761838590214,-15.036643707215,33.1753326131477)) ;
#60638=CARTESIAN_POINT('Ctrl Pts',(7.28867002732122,-15.036643707215,33.1817046287183)) ;
#60639=CARTESIAN_POINT('Ctrl Pts',(7.28688844246616,-14.9959966435996,33.1734956083764)) ;
#60640=CARTESIAN_POINT('Ctrl Pts',(7.28510452610483,-14.9552953856643,33.1652756333756)) ;
#60641=CARTESIAN_POINT('Ctrl Pts',(7.25860735275774,-14.3507293214144,33.0431780832932)) ;
#60642=CARTESIAN_POINT('Ctrl Pts',(7.23346099536329,-13.7767891025969,32.927263819543)) ;
#60643=CARTESIAN_POINT('Ctrl Pts',(7.18259964647052,-12.6154042535299,32.6927028386439)) ;
#60644=CARTESIAN_POINT('Ctrl Pts',(7.15688461897252,-12.0279596232834,32.5740561294197)) ;
#60645=CARTESIAN_POINT('Ctrl Pts',(7.10519001132364,-10.8463182046858,32.3353921438736)) ;
#60646=CARTESIAN_POINT('Ctrl Pts',(7.07921035581152,-10.2521214162831,32.21537488413)) ;
#60647=CARTESIAN_POINT('Ctrl Pts',(7.040273204793,-9.36082630688502,32.035341893136)) ;
#60648=CARTESIAN_POINT('Ctrl Pts',(7.02729958170864,-9.06372795314166,31.9753297049073)) ;
#60649=CARTESIAN_POINT('Ctrl Pts',(7.00140227647856,-8.47037530674386,31.8554729443044)) ;
#60650=CARTESIAN_POINT('Ctrl Pts',(6.98847858562182,-8.17412101408252,31.7956283738466)) ;
#60651=CARTESIAN_POINT('Ctrl Pts',(6.96272091250221,-7.5833005193592,31.6762766972686)) ;
#60652=CARTESIAN_POINT('Ctrl Pts',(6.94988691163539,-7.2887343173005,31.6167695952442)) ;
#60653=CARTESIAN_POINT('Ctrl Pts',(6.92434947612469,-6.70213403419977,31.4982624642858)) ;
#60654=CARTESIAN_POINT('Ctrl Pts',(6.91164600393193,-6.4100999531241,31.4392624436099)) ;
#60655=CARTESIAN_POINT('Ctrl Pts',(6.89272077672772,-5.97458094632212,31.3512696131719)) ;
#60656=CARTESIAN_POINT('Ctrl Pts',(6.88643404984998,-5.82982996436308,31.3220231992594)) ;
#60657=CARTESIAN_POINT('Ctrl Pts',(6.87390961359624,-5.54127754429721,31.2637205113756)) ;
#60658=CARTESIAN_POINT('Ctrl Pts',(6.86767190307711,-5.39747610618906,31.2346642376563)) ;
#60659=CARTESIAN_POINT('Ctrl Pts',(6.85525147412051,-5.11092827739036,31.1767628402795)) ;
#60660=CARTESIAN_POINT('Ctrl Pts',(6.84906874932502,-4.96818188670214,31.147917718022)) ;
#60661=CARTESIAN_POINT('Ctrl Pts',(6.83676475000976,-4.68384965683525,31.090459527349)) ;
#60662=CARTESIAN_POINT('Ctrl Pts',(6.83064346251804,-4.54226381764156,31.0618464617856)) ;
#60663=CARTESIAN_POINT('Ctrl Pts',(6.81846956547935,-4.26035819572789,31.004873119091)) ;
#60664=CARTESIAN_POINT('Ctrl Pts',(6.81241693002235,-4.12003841391635,30.9765128478552)) ;
#60665=CARTESIAN_POINT('Ctrl Pts',(6.80038888440364,-3.84077041358543,30.9200655383146)) ;
#60666=CARTESIAN_POINT('Ctrl Pts',(6.79441341605943,-3.7018221949867,30.8919785128001)) ;
#60667=CARTESIAN_POINT('Ctrl Pts',(6.78551640858875,-3.49450767079874,30.8500678221975)) ;
#60668=CARTESIAN_POINT('Ctrl Pts',(6.78256179852198,-3.42558746351796,30.8361342274587)) ;
#60669=CARTESIAN_POINT('Ctrl Pts',(6.77667653021486,-3.28812950621108,30.8083426961684)) ;
#60670=CARTESIAN_POINT('Ctrl Pts',(6.77374586998814,-3.21959175618158,30.7944847600546)) ;
#60671=CARTESIAN_POINT('Ctrl Pts',(6.76791086463551,-3.08291190325872,30.7668468168815)) ;
#60672=CARTESIAN_POINT('Ctrl Pts',(6.7650065040537,-3.01476980037891,30.7530668132276)) ;
#60673=CARTESIAN_POINT('Ctrl Pts',(6.75922734717836,-2.87889443316919,30.7255868111615)) ;
#60674=CARTESIAN_POINT('Ctrl Pts',(6.75635251278026,-2.81116116876676,30.7118868211215)) ;
#60675=CARTESIAN_POINT('Ctrl Pts',(6.75088517917376,-2.68197370257456,30.6857533838959)) ;
#60676=CARTESIAN_POINT('Ctrl Pts',(6.74815180308469,-2.61722529329389,30.672653870829)) ;
#60677=CARTESIAN_POINT('Ctrl Pts',(6.74397221313066,-2.51779041521477,30.6525328164037)) ;
#60678=CARTESIAN_POINT('Ctrl Pts',(6.74256579040069,-2.48426007858418,30.6457471612638)) ;
#60679=CARTESIAN_POINT('Ctrl Pts',(6.73974476333519,-2.41681407256003,30.6320961130316)) ;
#60680=CARTESIAN_POINT('Ctrl Pts',(6.73833014158143,-2.38289840312096,30.6252307237637)) ;
#60681=CARTESIAN_POINT('Ctrl Pts',(6.73551179023391,-2.31506715535754,30.6114975669625)) ;
#60682=CARTESIAN_POINT('Ctrl Pts',(6.73410801808841,-2.28115159069683,30.604629811687)) ;
#60683=CARTESIAN_POINT('Ctrl Pts',(6.73202609214958,-2.23056738538709,30.5943841391202)) ;
#60684=CARTESIAN_POINT('Ctrl Pts',(6.73133608993551,-2.21375417396992,30.5909782377709)) ;
#60685=CARTESIAN_POINT('Ctrl Pts',(6.72996696101551,-2.18027230832599,30.5841946304111)) ;
#60686=CARTESIAN_POINT('Ctrl Pts',(6.72928783210833,-2.16360365409132,30.5808169248839)) ;
#60687=CARTESIAN_POINT('Ctrl Pts',(6.72794380721774,-2.13045908081809,30.5740991649175)) ;
#60688=CARTESIAN_POINT('Ctrl Pts',(6.72727889411935,-2.11398316561836,30.570759115058)) ;
#60689=CARTESIAN_POINT('Ctrl Pts',(6.725967457352,-2.0812722521088,30.5641259470635)) ;
#60690=CARTESIAN_POINT('Ctrl Pts',(6.72532088666064,-2.06503725359408,30.5608328392358)) ;
#60691=CARTESIAN_POINT('Ctrl Pts',(6.72436922338636,-2.0409015794804,30.5559350542269)) ;
#60692=CARTESIAN_POINT('Ctrl Pts',(6.72405505930643,-2.03289249291726,30.5543094333854)) ;
#60693=CARTESIAN_POINT('Ctrl Pts',(6.72343394173311,-2.01695261920032,30.551073173184)) ;
#60694=CARTESIAN_POINT('Ctrl Pts',(6.72312698743446,-2.00902183204201,30.5494625340009)) ;
#60695=CARTESIAN_POINT('Ctrl Pts',(6.72252192513256,-1.99324458321975,30.5462571522277)) ;
#60696=CARTESIAN_POINT('Ctrl Pts',(6.72222378916939,-1.98539812173034,30.5446624158292)) ;
#60697=CARTESIAN_POINT('Ctrl Pts',(6.72178525733552,-1.97369619787999,30.5422827425759)) ;
#60698=CARTESIAN_POINT('Ctrl Pts',(6.7216405369464,-1.96980685143068,30.5414915875313)) ;
#60699=CARTESIAN_POINT('Ctrl Pts',(6.72135457499626,-1.96205150363523,30.5399134516662)) ;
#60700=CARTESIAN_POINT('Ctrl Pts',(6.72121333168194,-1.95818550227575,30.5391264712288)) ;
#60701=CARTESIAN_POINT('Ctrl Pts',(6.72093501346366,-1.95047267180703,30.5375556497875)) ;
#60702=CARTESIAN_POINT('Ctrl Pts',(6.72079052496425,-1.94642091385843,30.5367300763953)) ;
#60703=CARTESIAN_POINT('Ctrl Pts',(6.7205007238683,-1.93812468700046,30.5350383321452)) ;
#60704=CARTESIAN_POINT('Ctrl Pts',(6.72035534007046,-1.93388021741182,30.5341721768161)) ;
#60705=CARTESIAN_POINT('Ctrl Pts',(6.72014527293166,-1.92751377592369,30.5328712366358)) ;
#60706=CARTESIAN_POINT('Ctrl Pts',(6.72007660203497,-1.9253916858432,30.5324373045041)) ;
#60707=CARTESIAN_POINT('Ctrl Pts',(6.71994395320502,-1.92117173474938,30.5315735342658)) ;
#60708=CARTESIAN_POINT('Ctrl Pts',(6.71987994033495,-1.91907387328002,30.5311437037529)) ;
#60709=CARTESIAN_POINT('Ctrl Pts',(6.7197896717627,-1.91596334869304,30.5305053666097)) ;
#60710=CARTESIAN_POINT('Ctrl Pts',(6.71976055221698,-1.91493255558014,30.5302936539369)) ;
#60711=CARTESIAN_POINT('Ctrl Pts',(6.71970487564627,-1.91288607916449,30.5298728618694)) ;
#60712=CARTESIAN_POINT('Ctrl Pts',(6.71967831613871,-1.91187039581876,30.5296637830122)) ;
#60713=CARTESIAN_POINT('Ctrl Pts',(6.71962880631066,-1.90985715925278,30.5292486673054)) ;
#60714=CARTESIAN_POINT('Ctrl Pts',(6.71960581774062,-1.90885960785732,30.5290426392613)) ;
#60715=CARTESIAN_POINT('Ctrl Pts',(6.71957567318844,-1.9073791575924,30.5287360019001)) ;
#60716=CARTESIAN_POINT('Ctrl Pts',(6.71956635769722,-1.90688832081251,30.5286341882147)) ;
#60717=CARTESIAN_POINT('Ctrl Pts',(6.71954980425477,-1.9059123268808,30.5284313053881)) ;
#60718=CARTESIAN_POINT('Ctrl Pts',(6.7195425427954,-1.90542716908072,30.5283302412843)) ;
#60719=CARTESIAN_POINT('Ctrl Pts',(6.71953406025587,-1.90469706627519,30.5281776140417)) ;
#60720=CARTESIAN_POINT('Ctrl Pts',(6.719531472145,-1.9044367369481,30.528123096389)) ;
#60721=CARTESIAN_POINT('Ctrl Pts',(6.71952768036084,-1.9039038832069,30.5280111757878)) ;
#60722=CARTESIAN_POINT('Ctrl Pts',(6.71952647168563,-1.90363135860541,30.5279537739008)) ;
#60723=CARTESIAN_POINT('Ctrl Pts',(6.71952671038721,-1.90308662224053,30.527838451684)) ;
#60724=CARTESIAN_POINT('Ctrl Pts',(6.71952806578134,-1.90281444927565,30.5277805598112)) ;
#60725=CARTESIAN_POINT('Ctrl Pts',(6.7196030061094,-1.90163369649324,30.5275142094095)) ;
#60726=CARTESIAN_POINT('Ctrl Pts',(6.71960609582335,-1.90158501524993,30.5275032280517)) ;
#60727=CARTESIAN_POINT('Ctrl Pts',(6.7196091855373,-1.90153633400663,30.527492246694)) ;
#60728=CARTESIAN_POINT('',(-14.2513506240265,-15.0366437072153,30.8390862093178)) ;
#60729=CARTESIAN_POINT('',(-14.2782523899391,-15.0366437072153,30.8266401270699)) ;
#60730=CARTESIAN_POINT('Origin',(0.573544392334142,-21.6462763158694,-1.23969588788644)) ;
#60731=CARTESIAN_POINT('',(-13.1250168776941,-1.90153624278253,28.3692590890207)) ;
#60732=CARTESIAN_POINT('Ctrl Pts',(-13.1250168853804,-1.90153633399464,
28.3692591062341)) ;
#60733=CARTESIAN_POINT('Ctrl Pts',(-13.1250152689507,-1.90158489352019,
28.3692709113022)) ;
#60734=CARTESIAN_POINT('Ctrl Pts',(-13.1249874709885,-1.90241997831702,
28.3694739246719)) ;
#60735=CARTESIAN_POINT('Ctrl Pts',(-13.1249998825665,-1.90282053513345,
28.3695593911006)) ;
#60736=CARTESIAN_POINT('Ctrl Pts',(-13.125011087353,-1.90309401671833,28.3696164802336)) ;
#60737=CARTESIAN_POINT('Ctrl Pts',(-13.1250358173985,-1.90364137046846,
28.3697296738716)) ;
#60738=CARTESIAN_POINT('Ctrl Pts',(-13.1250494264321,-1.90391520380722,
28.3697857307775)) ;
#60739=CARTESIAN_POINT('Ctrl Pts',(-13.1250773667014,-1.90445061563352,
28.3698947199767)) ;
#60740=CARTESIAN_POINT('Ctrl Pts',(-13.1250917025522,-1.90471219430631,
28.3699476501771)) ;
#60741=CARTESIAN_POINT('Ctrl Pts',(-13.1251330497042,-1.9054458369876,28.3700955747726)) ;
#60742=CARTESIAN_POINT('Ctrl Pts',(-13.1251620395678,-1.90593335948141,
28.3701931737557)) ;
#60743=CARTESIAN_POINT('Ctrl Pts',(-13.1252221711934,-1.90691411034398,
28.3703886754018)) ;
#60744=CARTESIAN_POINT('Ctrl Pts',(-13.1252533348784,-1.90740733936085,
28.3704865680697)) ;
#60745=CARTESIAN_POINT('Ctrl Pts',(-13.1253492373837,-1.9088950048919,28.3707809471545)) ;
#60746=CARTESIAN_POINT('Ctrl Pts',(-13.1254163516026,-1.90989741787098,
28.3709781508729)) ;
#60747=CARTESIAN_POINT('Ctrl Pts',(-13.1255547019883,-1.91192046573787,
28.3713748005062)) ;
#60748=CARTESIAN_POINT('Ctrl Pts',(-13.1256259736338,-1.91294109879846,
28.3715742295908)) ;
#60749=CARTESIAN_POINT('Ctrl Pts',(-13.1257715916628,-1.91499754808388,
28.3719751225115)) ;
#60750=CARTESIAN_POINT('Ctrl Pts',(-13.1258459404148,-1.91603336435267,
28.3721765852616)) ;
#60751=CARTESIAN_POINT('Ctrl Pts',(-13.1260725286467,-1.9191590465366,28.3727834866439)) ;
#60752=CARTESIAN_POINT('Ctrl Pts',(-13.1262282666174,-1.9212671305763,28.3731914550528)) ;
#60753=CARTESIAN_POINT('Ctrl Pts',(-13.1265451591989,-1.92550764432193,
28.3740104294866)) ;
#60754=CARTESIAN_POINT('Ctrl Pts',(-13.1267063463805,-1.92764007448401,
28.3744214205466)) ;
#60755=CARTESIAN_POINT('Ctrl Pts',(-13.1271936927362,-1.93403753623515,
28.3756526816843)) ;
#60756=CARTESIAN_POINT('Ctrl Pts',(-13.1275235719574,-1.93830268601545,
28.3764712575976)) ;
#60757=CARTESIAN_POINT('Ctrl Pts',(-13.1281736016328,-1.94663933327223,
28.3780688149077)) ;
#60758=CARTESIAN_POINT('Ctrl Pts',(-13.1284938184142,-1.95071083142766,
28.3788477657729)) ;
#60759=CARTESIAN_POINT('Ctrl Pts',(-13.129106438373,-1.95846141009329,28.3803291801374)) ;
#60760=CARTESIAN_POINT('Ctrl Pts',(-13.1294151360898,-1.96234641865746,
28.3810709957486)) ;
#60761=CARTESIAN_POINT('Ctrl Pts',(-13.1300368386708,-1.97013989558661,
28.3825579761773)) ;
#60762=CARTESIAN_POINT('Ctrl Pts',(-13.1303498452033,-1.97404836396523,
28.3833031402261)) ;
#60763=CARTESIAN_POINT('Ctrl Pts',(-13.1312944889748,-1.98580782013941,
28.3855437839311)) ;
#60764=CARTESIAN_POINT('Ctrl Pts',(-13.1319317073656,-1.99369285855913,
28.3870444349558)) ;
#60765=CARTESIAN_POINT('Ctrl Pts',(-13.1332181965959,-2.0095476757302,28.3900594567134)) ;
#60766=CARTESIAN_POINT('Ctrl Pts',(-13.1338674934606,-2.0175174543069,28.3915738153658)) ;
#60767=CARTESIAN_POINT('Ctrl Pts',(-13.135176390318,-2.03353569574261,28.3946156827108)) ;
#60768=CARTESIAN_POINT('Ctrl Pts',(-13.1358359910487,-2.04158415860608,
28.3961431910624)) ;
#60769=CARTESIAN_POINT('Ctrl Pts',(-13.1378283038094,-2.06583849453389,
28.4007442732752)) ;
#60770=CARTESIAN_POINT('Ctrl Pts',(-13.1391744335532,-2.08215331147535,
28.4038364464638)) ;
#60771=CARTESIAN_POINT('Ctrl Pts',(-13.1418947741956,-2.11502504608969,
28.41006292857)) ;
#60772=CARTESIAN_POINT('Ctrl Pts',(-13.1432690289151,-2.13158196396751,
28.4131972172602)) ;
#60773=CARTESIAN_POINT('Ctrl Pts',(-13.1460395960048,-2.1648894899987,28.4194996938546)) ;
#60774=CARTESIAN_POINT('Ctrl Pts',(-13.1474359241405,-2.18164009431291,
28.4226678735906)) ;
#60775=CARTESIAN_POINT('Ctrl Pts',(-13.1502453305346,-2.21528657066704,
28.4290295617627)) ;
#60776=CARTESIAN_POINT('Ctrl Pts',(-13.1516584108559,-2.23218244271495,
28.4322230692458)) ;
#60777=CARTESIAN_POINT('Ctrl Pts',(-13.1559153789589,-2.28301534046843,
28.4418284715407)) ;
#60778=CARTESIAN_POINT('Ctrl Pts',(-13.158776927892,-2.31709764749398,28.4482652766609)) ;
#60779=CARTESIAN_POINT('Ctrl Pts',(-13.164510098709,-2.38526237999286,28.4611342536291)) ;
#60780=CARTESIAN_POINT('Ctrl Pts',(-13.1673817596031,-2.41934479180169,
28.4675664043175)) ;
#60781=CARTESIAN_POINT('Ctrl Pts',(-13.1730997731453,-2.48712238776894,
28.4803542410124)) ;
#60782=CARTESIAN_POINT('Ctrl Pts',(-13.1759461420269,-2.52081757197294,
28.4867099195188)) ;
#60783=CARTESIAN_POINT('Ctrl Pts',(-13.1843953174782,-2.6207413083776,28.5055540107254)) ;
#60784=CARTESIAN_POINT('Ctrl Pts',(-13.1899080876518,-2.68580804401566,
28.5178195277039)) ;
#60785=CARTESIAN_POINT('Ctrl Pts',(-13.2009227453959,-2.81566305062235,
28.5422921887985)) ;
#60786=CARTESIAN_POINT('Ctrl Pts',(-13.2067068091717,-2.8837618261483,28.5551226014694)) ;
#60787=CARTESIAN_POINT('Ctrl Pts',(-13.2183211631654,-3.02037042177582,
28.580855636929)) ;
#60788=CARTESIAN_POINT('Ctrl Pts',(-13.2241514889584,-3.08888024195006,
28.5937582432754)) ;
#60789=CARTESIAN_POINT('Ctrl Pts',(-13.2358547746908,-3.22629766446251,
28.6196343081466)) ;
#60790=CARTESIAN_POINT('Ctrl Pts',(-13.2417277490524,-3.2952052667871,28.6326077599955)) ;
#60791=CARTESIAN_POINT('Ctrl Pts',(-13.2535135489871,-3.43340499251651,
28.6586237837857)) ;
#60792=CARTESIAN_POINT('Ctrl Pts',(-13.2594263764131,-3.50269711592473,
28.6716663548693)) ;
#60793=CARTESIAN_POINT('Ctrl Pts',(-13.2772211700303,-3.71113037749264,
28.7108948224511)) ;
#60794=CARTESIAN_POINT('Ctrl Pts',(-13.2891593483695,-3.85082840634055,
28.7371815190198)) ;
#60795=CARTESIAN_POINT('Ctrl Pts',(-13.3131704391015,-4.13160342849318,
28.7900065741187)) ;
#60796=CARTESIAN_POINT('Ctrl Pts',(-13.3252434057619,-4.27268042187732,
28.81654490756)) ;
#60797=CARTESIAN_POINT('Ctrl Pts',(-13.3495113303093,-4.55610729892767,
28.8698549782839)) ;
#60798=CARTESIAN_POINT('Ctrl Pts',(-13.3617063123166,-4.69845718168438,
28.8966267042002)) ;
#60799=CARTESIAN_POINT('Ctrl Pts',(-13.3862067189839,-4.98432376133397,
28.9503847487854)) ;
#60800=CARTESIAN_POINT('Ctrl Pts',(-13.3985121557369,-5.1278404582419,28.977371061863)) ;
#60801=CARTESIAN_POINT('Ctrl Pts',(-13.4232226290045,-5.41593459280462,
29.0315391438259)) ;
#60802=CARTESIAN_POINT('Ctrl Pts',(-13.4356276714463,-5.5605120304571,29.0587209099683)) ;
#60803=CARTESIAN_POINT('Ctrl Pts',(-13.4605269614328,-5.85062157360454,
29.1132605538531)) ;
#60804=CARTESIAN_POINT('Ctrl Pts',(-13.4730212100494,-5.99615367910082,
29.1406184310989)) ;
#60805=CARTESIAN_POINT('Ctrl Pts',(-13.5106226096791,-6.43402288850668,
29.2229270113459)) ;
#60806=CARTESIAN_POINT('Ctrl Pts',(-13.5358483446402,-6.72763288063727,
29.2781126940939)) ;
#60807=CARTESIAN_POINT('Ctrl Pts',(-13.5865374915687,-7.31739864982827,
29.3889537854771)) ;
#60808=CARTESIAN_POINT('Ctrl Pts',(-13.6120009385329,-7.61355442692234,
29.4446091779287)) ;
#60809=CARTESIAN_POINT('Ctrl Pts',(-13.6630887777036,-8.20756318104024,
29.5562319618921)) ;
#60810=CARTESIAN_POINT('Ctrl Pts',(-13.6887131872509,-8.5054161580608,29.6121993453803)) ;
#60811=CARTESIAN_POINT('Ctrl Pts',(-13.7400472188843,-9.10197072784479,
29.72428792256)) ;
#60812=CARTESIAN_POINT('Ctrl Pts',(-13.7657568490879,-9.40067232061517,
29.7804091124971)) ;
#60813=CARTESIAN_POINT('Ctrl Pts',(-13.8429009085766,-10.2967771471123,
29.9487656754132)) ;
#60814=CARTESIAN_POINT('Ctrl Pts',(-13.8943503623133,-10.8941804135972,
30.0609941047966)) ;
#60815=CARTESIAN_POINT('Ctrl Pts',(-13.9966930472064,-12.0821983511367,
30.2841625050184)) ;
#60816=CARTESIAN_POINT('Ctrl Pts',(-14.0475863486027,-12.6728130222429,
30.395102443371)) ;
#60817=CARTESIAN_POINT('Ctrl Pts',(-14.1497718947981,-13.858425809999,30.6177958799877)) ;
#60818=CARTESIAN_POINT('Ctrl Pts',(-14.201028282145,-14.452999812307,30.7294693948825)) ;
#60819=CARTESIAN_POINT('Ctrl Pts',(-14.2513506239133,-15.0366437072152,
30.8390862093702)) ;
#60820=CARTESIAN_POINT('Ctrl Pts',(-14.2782523900534,-15.0366437072152,
30.826640127017)) ;
#60821=CARTESIAN_POINT('Ctrl Pts',(-14.2767312222616,-15.019224461707,30.8233774515699)) ;
#60822=CARTESIAN_POINT('Ctrl Pts',(-14.2752091967655,-15.0017954800496,
30.820112955973)) ;
#60823=CARTESIAN_POINT('Ctrl Pts',(-14.2241842264702,-14.4175024634034,
30.7106734040413)) ;
#60824=CARTESIAN_POINT('Ctrl Pts',(-14.1737849268775,-13.8404650781122,
30.6025965267698)) ;
#60825=CARTESIAN_POINT('Ctrl Pts',(-14.0717790076265,-12.6728130216194,
30.3839097272942)) ;
#60826=CARTESIAN_POINT('Ctrl Pts',(-14.0201724215192,-12.0821983504207,
30.2732997895684)) ;
#60827=CARTESIAN_POINT('Ctrl Pts',(-13.9163371854979,-10.894180412695,30.0508219169878)) ;
#60828=CARTESIAN_POINT('Ctrl Pts',(-13.8641086058156,-10.2967771461165,
29.9389539496297)) ;
#60829=CARTESIAN_POINT('Ctrl Pts',(-13.7857356278822,-9.40067231947891,
29.7711659448977)) ;
#60830=CARTESIAN_POINT('Ctrl Pts',(-13.7596062483987,-9.10197072666172,
29.7152389516462)) ;
#60831=CARTESIAN_POINT('Ctrl Pts',(-13.7074095360729,-8.50541615678423,
29.6035494930342)) ;
#60832=CARTESIAN_POINT('Ctrl Pts',(-13.6813422113468,-8.20756317971701,
29.5477870239176)) ;
#60833=CARTESIAN_POINT('Ctrl Pts',(-13.6293411273122,-7.61355442550602,
29.4365867519988)) ;
#60834=CARTESIAN_POINT('Ctrl Pts',(-13.6034073853457,-7.31739864836555,
29.3811489411741)) ;
#60835=CARTESIAN_POINT('Ctrl Pts',(-13.5517439698451,-6.72763287908212,
29.2707585944094)) ;
#60836=CARTESIAN_POINT('Ctrl Pts',(-13.5260143313033,-6.43402288690552,
29.2158060422727)) ;
#60837=CARTESIAN_POINT('Ctrl Pts',(-13.4876244850302,-5.99615367743104,
29.1338622362707)) ;
#60838=CARTESIAN_POINT('Ctrl Pts',(-13.4748619542748,-5.85062157191195,
29.1066284795542)) ;
#60839=CARTESIAN_POINT('Ctrl Pts',(-13.4494133660394,-5.56051202871903,
29.0523429680906)) ;
#60840=CARTESIAN_POINT('Ctrl Pts',(-13.4367273096283,-5.41593459104392,
29.0252912128496)) ;
#60841=CARTESIAN_POINT('Ctrl Pts',(-13.4114396744369,-5.12784045643605,
28.9713901544167)) ;
#60842=CARTESIAN_POINT('Ctrl Pts',(-13.3988381015846,-4.9843237595056,28.944540848483)) ;
#60843=CARTESIAN_POINT('Ctrl Pts',(-13.3737269870879,-4.69845717981123,
28.8910653474164)) ;
#60844=CARTESIAN_POINT('Ctrl Pts',(-13.361217457538,-4.5561072970322,28.8644391466846)) ;
#60845=CARTESIAN_POINT('Ctrl Pts',(-13.3362972659841,-4.27268041993744,
28.8114308468023)) ;
#60846=CARTESIAN_POINT('Ctrl Pts',(-13.3238866282584,-4.13160342653121,
28.7850487366265)) ;
#60847=CARTESIAN_POINT('Ctrl Pts',(-13.2991698265207,-3.85082840433457,
28.7325501781962)) ;
#60848=CARTESIAN_POINT('Ctrl Pts',(-13.2868637167631,-3.71113037546474,
28.7064337048231)) ;
#60849=CARTESIAN_POINT('Ctrl Pts',(-13.2684853726168,-3.50269711386417,
28.6674752164577)) ;
#60850=CARTESIAN_POINT('Ctrl Pts',(-13.2623727032127,-3.43340499044509,
28.6545251021161)) ;
#60851=CARTESIAN_POINT('Ctrl Pts',(-13.2501742422854,-3.29520526469404,
28.6286999956262)) ;
#60852=CARTESIAN_POINT('Ctrl Pts',(-13.2440884526162,-3.22629766235862,
28.6158250026206)) ;
#60853=CARTESIAN_POINT('Ctrl Pts',(-13.2319432445035,-3.08888023982465,
28.5901533928093)) ;
#60854=CARTESIAN_POINT('Ctrl Pts',(-13.2258838404854,-3.02037041963968,
28.5773567693331)) ;
#60855=CARTESIAN_POINT('Ctrl Pts',(-13.2137900707746,-2.88376182399075,
28.5518455351981)) ;
#60856=CARTESIAN_POINT('Ctrl Pts',(-13.2077557406446,-2.81566304845413,
28.5391309080698)) ;
#60857=CARTESIAN_POINT('Ctrl Pts',(-13.1962343453602,-2.68580804224111,
28.5148926888158)) ;
#60858=CARTESIAN_POINT('Ctrl Pts',(-13.1904549255703,-2.62074130702757,
28.5027505371832)) ;
#60859=CARTESIAN_POINT('Ctrl Pts',(-13.1815625546521,-2.52081757127485,
28.4841114901825)) ;
#60860=CARTESIAN_POINT('Ctrl Pts',(-13.1785611978528,-2.4871223872907,28.4778275167724)) ;
#60861=CARTESIAN_POINT('Ctrl Pts',(-13.1725165575394,-2.41934479176566,
28.4651907938141)) ;
#60862=CARTESIAN_POINT('Ctrl Pts',(-13.169473290243,-2.38526238017923,28.4588380367523)) ;
#60863=CARTESIAN_POINT('Ctrl Pts',(-13.163376620504,-2.31709764812506,28.4461372323948)) ;
#60864=CARTESIAN_POINT('Ctrl Pts',(-13.1603232594475,-2.28301534132186,
28.4397891690633)) ;
#60865=CARTESIAN_POINT('Ctrl Pts',(-13.1557582890889,-2.23218244390001,
28.4303262638613)) ;
#60866=CARTESIAN_POINT('Ctrl Pts',(-13.1542391276856,-2.21528657196237,
28.427181834738)) ;
#60867=CARTESIAN_POINT('Ctrl Pts',(-13.1512092615423,-2.18164009582775,
28.420922142157)) ;
#60868=CARTESIAN_POINT('Ctrl Pts',(-13.1496985588601,-2.16488949162284,
28.4178068777459)) ;
#60869=CARTESIAN_POINT('Ctrl Pts',(-13.146688677501,-2.13158196580896,28.411615119772)) ;
#60870=CARTESIAN_POINT('Ctrl Pts',(-13.1451895152596,-2.11502504803915,
28.4085386194796)) ;
#60871=CARTESIAN_POINT('Ctrl Pts',(-13.142205038103,-2.08215331363928,28.4024343399867)) ;
#60872=CARTESIAN_POINT('Ctrl Pts',(-13.1407197669701,-2.06583849680426,
28.3994065404838)) ;
#60873=CARTESIAN_POINT('Ctrl Pts',(-13.1385027926659,-2.0415841610347,28.3949093978052)) ;
#60874=CARTESIAN_POINT('Ctrl Pts',(-13.13776560024,-2.03353569822372,28.3934177872064)) ;
#60875=CARTESIAN_POINT('Ctrl Pts',(-13.1362945662569,-2.01751745689249,
28.3904509325074)) ;
#60876=CARTESIAN_POINT('Ctrl Pts',(-13.1355607254437,-2.00954767836777,
28.3889756880625)) ;
#60877=CARTESIAN_POINT('Ctrl Pts',(-13.1340956457591,-1.99369286130014,
28.386043291071)) ;
#60878=CARTESIAN_POINT('Ctrl Pts',(-13.1333644329482,-1.98580782293182,
28.3845861265074)) ;
#60879=CARTESIAN_POINT('Ctrl Pts',(-13.1322682487679,-1.97404836683433,
28.3824155928787)) ;
#60880=CARTESIAN_POINT('Ctrl Pts',(-13.1319029491467,-1.97013989848118,
28.3816946221949)) ;
#60881=CARTESIAN_POINT('Ctrl Pts',(-13.1311721108169,-1.96234642160287,
28.3802581333518)) ;
#60882=CARTESIAN_POINT('Ctrl Pts',(-13.1308065737453,-1.95846141306429,
28.3795426144322)) ;
#60883=CARTESIAN_POINT('Ctrl Pts',(-13.130074097652,-1.95071083402189,28.3781166513345)) ;
#60884=CARTESIAN_POINT('Ctrl Pts',(-13.1296877147739,-1.94663933544429,
28.3773683120693)) ;
#60885=CARTESIAN_POINT('Ctrl Pts',(-13.128890937428,-1.93830268732315,28.3758386472643)) ;
#60886=CARTESIAN_POINT('Ctrl Pts',(-13.1284806092105,-1.93403753710027,
28.3750572909193)) ;
#60887=CARTESIAN_POINT('Ctrl Pts',(-13.1278576899737,-1.92764007468588,
28.3738887523245)) ;
#60888=CARTESIAN_POINT('Ctrl Pts',(-13.1276487985248,-1.92550764430288,
28.3734998315585)) ;
#60889=CARTESIAN_POINT('Ctrl Pts',(-13.1272297591529,-1.92126713011769,
28.3727281151621)) ;
#60890=CARTESIAN_POINT('Ctrl Pts',(-13.127019643716,-1.91915904585948,28.3723453043983)) ;
#60891=CARTESIAN_POINT('Ctrl Pts',(-13.1267037765904,-1.91603336335157,
28.3717797077569)) ;
#60892=CARTESIAN_POINT('Ctrl Pts',(-13.1265983616708,-1.9149975469756,28.3715926177219)) ;
#60893=CARTESIAN_POINT('Ctrl Pts',(-13.1263870873875,-1.91294109747722,
28.3712221005706)) ;
#60894=CARTESIAN_POINT('Ctrl Pts',(-13.1262812303145,-1.91192046431214,
28.3710386723848)) ;
#60895=CARTESIAN_POINT('Ctrl Pts',(-13.1260684851354,-1.90989741623553,
28.3706764414003)) ;
#60896=CARTESIAN_POINT('Ctrl Pts',(-13.1259616328263,-1.90889500315093,
28.3704976224562)) ;
#60897=CARTESIAN_POINT('Ctrl Pts',(-13.1257993541946,-1.90740733746617,
28.3702339522025)) ;
#60898=CARTESIAN_POINT('Ctrl Pts',(-13.1257449190146,-1.90691410839945,
28.3701468260634)) ;
#60899=CARTESIAN_POINT('Ctrl Pts',(-13.1256348434522,-1.90593335743554,
28.3699744309199)) ;
#60900=CARTESIAN_POINT('Ctrl Pts',(-13.1255792249402,-1.90544583488841,
28.3698891516492)) ;
#60901=CARTESIAN_POINT('Ctrl Pts',(-13.1254932500023,-1.90471219217896,
28.3697618740597)) ;
#60902=CARTESIAN_POINT('Ctrl Pts',(-13.1254621892913,-1.90445061353546,
28.3697166816103)) ;
#60903=CARTESIAN_POINT('Ctrl Pts',(-13.1253972100148,-1.90391520175604,
28.3696248284912)) ;
#60904=CARTESIAN_POINT('Ctrl Pts',(-13.1253632960718,-1.9036413684333,28.3695781656405)) ;
#60905=CARTESIAN_POINT('Ctrl Pts',(-13.1252930340526,-1.90309401473251,
28.3694860373478)) ;
#60906=CARTESIAN_POINT('Ctrl Pts',(-13.1252567766583,-1.90282053317478,
28.3694405387916)) ;
#60907=CARTESIAN_POINT('Ctrl Pts',(-13.1250350734088,-1.90163369914819,
28.369272862051)) ;
#60908=CARTESIAN_POINT('Ctrl Pts',(-13.1250259793946,-1.90158501657141,
28.3692659841426)) ;
#60909=CARTESIAN_POINT('Ctrl Pts',(-13.1250168853804,-1.90153633399464,
28.3692591062341)) ;
#60910=CARTESIAN_POINT('',(-25.8831717248504,-15.0366437072153,22.0048097991458)) ;
#60911=CARTESIAN_POINT('',(-25.9023611320428,-15.0366437072153,21.98221828251)) ;
#60912=CARTESIAN_POINT('Origin',(1.04106958514517,-21.6462763158693,-0.884292476110772)) ;
#60913=CARTESIAN_POINT('',(-23.8238854115647,-1.90153624079472,20.2361906783538)) ;
#60914=CARTESIAN_POINT('Ctrl Pts',(-23.8238854254577,-1.90153633001901,
20.23619069048)) ;
#60915=CARTESIAN_POINT('Ctrl Pts',(-23.8238889212641,-1.90158489068798,
20.23620207647)) ;
#60916=CARTESIAN_POINT('Ctrl Pts',(-23.8239492198937,-1.9024225062293,20.2363984716666)) ;
#60917=CARTESIAN_POINT('Ctrl Pts',(-23.8239965310121,-1.90282422971975,
20.2364710111718)) ;
#60918=CARTESIAN_POINT('Ctrl Pts',(-23.8240307835122,-1.90309850720873,
20.2365182410673)) ;
#60919=CARTESIAN_POINT('Ctrl Pts',(-23.8241009836495,-1.90364745287506,
20.2366108299045)) ;
#60920=CARTESIAN_POINT('Ctrl Pts',(-23.8241369875051,-1.90392208221389,
20.2366561102625)) ;
#60921=CARTESIAN_POINT('Ctrl Pts',(-23.8242083345894,-1.90445904989118,
20.2367435251871)) ;
#60922=CARTESIAN_POINT('Ctrl Pts',(-23.8242436812157,-1.90472138841956,
20.236785655814)) ;
#60923=CARTESIAN_POINT('Ctrl Pts',(-23.8243436342305,-1.90545718379177,
20.2369028631524)) ;
#60924=CARTESIAN_POINT('Ctrl Pts',(-23.8244111378045,-1.90594614422066,
20.2369794780989)) ;
#60925=CARTESIAN_POINT('Ctrl Pts',(-23.8245482298291,-1.90692978769714,
20.2371320802637)) ;
#60926=CARTESIAN_POINT('Ctrl Pts',(-23.8246178340023,-1.90742447139286,
20.2372080491789)) ;
#60927=CARTESIAN_POINT('Ctrl Pts',(-23.8248291351697,-1.90891652441222,
20.2374355804445)) ;
#60928=CARTESIAN_POINT('Ctrl Pts',(-23.8249732947336,-1.90992189364657,
20.2375867973708)) ;
#60929=CARTESIAN_POINT('Ctrl Pts',(-23.825266307357,-1.91195090760971,20.2378895395296)) ;
#60930=CARTESIAN_POINT('Ctrl Pts',(-23.8254151855814,-1.9129745505112,20.2380410345524)) ;
#60931=CARTESIAN_POINT('Ctrl Pts',(-23.8257165959959,-1.91503706413992,
20.2383445838546)) ;
#60932=CARTESIAN_POINT('Ctrl Pts',(-23.8258691298177,-1.91607593490945,
20.2384966362262)) ;
#60933=CARTESIAN_POINT('Ctrl Pts',(-23.8263310116615,-1.91921083418716,
20.2389535916698)) ;
#60934=CARTESIAN_POINT('Ctrl Pts',(-23.8266446075399,-1.9213251344095,20.2392593264881)) ;
#60935=CARTESIAN_POINT('Ctrl Pts',(-23.827278005508,-1.92557815197685,20.2398712840593)) ;
#60936=CARTESIAN_POINT('Ctrl Pts',(-23.8275978309142,-1.9277168697781,20.2401774795076)) ;
#60937=CARTESIAN_POINT('Ctrl Pts',(-23.8285600272612,-1.93413319445796,
20.2410929181444)) ;
#60938=CARTESIAN_POINT('Ctrl Pts',(-23.8292050669925,-1.93841091953424,
20.241699057121)) ;
#60939=CARTESIAN_POINT('Ctrl Pts',(-23.8304696089694,-1.9467721457928,20.2428793998365)) ;
#60940=CARTESIAN_POINT('Ctrl Pts',(-23.8310891586715,-1.95085564765416,
20.2434535479221)) ;
#60941=CARTESIAN_POINT('Ctrl Pts',(-23.8322707390319,-1.9586291805441,20.2445439567061)) ;
#60942=CARTESIAN_POINT('Ctrl Pts',(-23.8328641758305,-1.96252574723342,
20.245089173699)) ;
#60943=CARTESIAN_POINT('Ctrl Pts',(-23.8340563782582,-1.97034241017641,
20.246180845225)) ;
#60944=CARTESIAN_POINT('Ctrl Pts',(-23.8346551450615,-1.9742625064435,20.2467272983799)) ;
#60945=CARTESIAN_POINT('Ctrl Pts',(-23.8364587317813,-1.98605694755246,
20.2483689818616)) ;
#60946=CARTESIAN_POINT('Ctrl Pts',(-23.8376708072141,-1.99396544428758,
20.249466572326)) ;
#60947=CARTESIAN_POINT('Ctrl Pts',(-23.8401117020587,-2.00986743013604,
20.2516691720465)) ;
#60948=CARTESIAN_POINT('Ctrl Pts',(-23.8413405400649,-2.0178609190749,20.2527741593558)) ;
#60949=CARTESIAN_POINT('Ctrl Pts',(-23.8438131290869,-2.03392681527835,
20.254991769387)) ;
#60950=CARTESIAN_POINT('Ctrl Pts',(-23.8450568806311,-2.04199922254737,
20.2561043914876)) ;
#60951=CARTESIAN_POINT('Ctrl Pts',(-23.8488082444504,-2.06632571575214,
20.2594534651195)) ;
#60952=CARTESIAN_POINT('Ctrl Pts',(-23.8513358992443,-2.08268906962494,
20.2617012013615)) ;
#60953=CARTESIAN_POINT('Ctrl Pts',(-23.8564345078822,-2.11565859823547,
20.2662232117135)) ;
#60954=CARTESIAN_POINT('Ctrl Pts',(-23.8590054930501,-2.13226477317813,
20.2684974490114)) ;
#60955=CARTESIAN_POINT('Ctrl Pts',(-23.8641818125931,-2.16567138944634,
20.2730674984476)) ;
#60956=CARTESIAN_POINT('Ctrl Pts',(-23.866787157862,-2.18247182693246,20.2753632965351)) ;
#60957=CARTESIAN_POINT('Ctrl Pts',(-23.8720237580892,-2.21621840171076,
20.2799708998623)) ;
#60958=CARTESIAN_POINT('Ctrl Pts',(-23.8746550145169,-2.23316453901088,
20.2822827033741)) ;
#60959=CARTESIAN_POINT('Ctrl Pts',(-23.8825753927727,-2.28414866460182,
20.289233302234)) ;
#60960=CARTESIAN_POINT('Ctrl Pts',(-23.8878910763925,-2.31833236629326,
20.2938873413591)) ;
#60961=CARTESIAN_POINT('Ctrl Pts',(-23.8985296507322,-2.38669988812742,
20.3031869725674)) ;
#60962=CARTESIAN_POINT('Ctrl Pts',(-23.9038525680176,-2.42088369460506,
20.3078325290128)) ;
#60963=CARTESIAN_POINT('Ctrl Pts',(-23.9144431540245,-2.48886292769985,
20.3170647066451)) ;
#60964=CARTESIAN_POINT('Ctrl Pts',(-23.9197108343457,-2.52265835436257,
20.3216513141901)) ;
#60965=CARTESIAN_POINT('Ctrl Pts',(-23.9353381111146,-2.6228793615095,20.3352460832032)) ;
#60966=CARTESIAN_POINT('Ctrl Pts',(-23.9455218681759,-2.68813966879725,
20.344089279458)) ;
#60967=CARTESIAN_POINT('Ctrl Pts',(-23.9658579668207,-2.8184007703173,20.3617298151846)) ;
#60968=CARTESIAN_POINT('Ctrl Pts',(-23.9765296668213,-2.88672197974776,
20.3709756639712)) ;
#60969=CARTESIAN_POINT('Ctrl Pts',(-23.9979455672397,-3.02377678576226,
20.3895136499768)) ;
#60970=CARTESIAN_POINT('Ctrl Pts',(-24.0086897931138,-3.09251038241904,
20.3988057572494)) ;
#60971=CARTESIAN_POINT('Ctrl Pts',(-24.0302469042348,-3.23037665716361,
20.4174365347916)) ;
#60972=CARTESIAN_POINT('Ctrl Pts',(-24.0410597997926,-3.29950933523776,
20.4267751929177)) ;
#60973=CARTESIAN_POINT('Ctrl Pts',(-24.0627509880244,-3.43816046842335,
20.4454986657553)) ;
#60974=CARTESIAN_POINT('Ctrl Pts',(-24.0736292820235,-3.50767892353821,
20.4548834789066)) ;
#60975=CARTESIAN_POINT('Ctrl Pts',(-24.1063578732419,-3.71679299919776,
20.4831059472441)) ;
#60976=CARTESIAN_POINT('Ctrl Pts',(-24.1283018087199,-3.8569473294019,20.5020117146455)) ;
#60977=CARTESIAN_POINT('Ctrl Pts',(-24.1724183592319,-4.13863945838501,
20.5399956588899)) ;
#60978=CARTESIAN_POINT('Ctrl Pts',(-24.194591013067,-4.28017725724343,20.5590737900776)) ;
#60979=CARTESIAN_POINT('Ctrl Pts',(-24.2391457094888,-4.56452990289024,
20.5973912011102)) ;
#60980=CARTESIAN_POINT('Ctrl Pts',(-24.2615277692301,-4.70734474876847,
20.6166304604686)) ;
#60981=CARTESIAN_POINT('Ctrl Pts',(-24.306482840028,-4.99414506583698,20.6552578617666)) ;
#60982=CARTESIAN_POINT('Ctrl Pts',(-24.3290558597318,-5.13813053704231,
20.6746459935306)) ;
#60983=CARTESIAN_POINT('Ctrl Pts',(-24.3743749176294,-5.42716568490539,
20.7135582803702)) ;
#60984=CARTESIAN_POINT('Ctrl Pts',(-24.3971209600605,-5.57221536156083,
20.7330824304562)) ;
#60985=CARTESIAN_POINT('Ctrl Pts',(-24.442768450973,-5.86327250094969,20.7722535176391)) ;
#60986=CARTESIAN_POINT('Ctrl Pts',(-24.4656699002175,-6.00927996368441,
20.7919004538369)) ;
#60987=CARTESIAN_POINT('Ctrl Pts',(-24.5345812515141,-6.44857940245386,
20.8510052199905)) ;
#60988=CARTESIAN_POINT('Ctrl Pts',(-24.580798106769,-6.7431484243555,20.8906270652943)) ;
#60989=CARTESIAN_POINT('Ctrl Pts',(-24.673646087651,-7.3348405683828,20.9701983608142)) ;
#60990=CARTESIAN_POINT('Ctrl Pts',(-24.7202772382944,-7.63196369054212,
21.0101477815896)) ;
#60991=CARTESIAN_POINT('Ctrl Pts',(-24.8138175020744,-8.22791267832212,
21.0902629313793)) ;
#60992=CARTESIAN_POINT('Ctrl Pts',(-24.8607266276025,-8.52673854393955,
21.1304286458044)) ;
#60993=CARTESIAN_POINT('Ctrl Pts',(-24.9546872472594,-9.12524166268665,
21.2108642459101)) ;
#60994=CARTESIAN_POINT('Ctrl Pts',(-25.001738747189,-9.42491891582326,21.2511341247632)) ;
#60995=CARTESIAN_POINT('Ctrl Pts',(-25.142904087342,-10.3239507234301,21.3719310144489)) ;
#60996=CARTESIAN_POINT('Ctrl Pts',(-25.2370286632435,-10.9233053106647,
21.4524453967184)) ;
#60997=CARTESIAN_POINT('Ctrl Pts',(-25.4242285326933,-12.1152037156214,
21.6125353332349)) ;
#60998=CARTESIAN_POINT('Ctrl Pts',(-25.5173038764335,-12.707747533395,21.6921108284061)) ;
#60999=CARTESIAN_POINT('Ctrl Pts',(-25.7018585299048,-13.8825790582674,
21.8498668522659)) ;
#61000=CARTESIAN_POINT('Ctrl Pts',(-25.7933256204984,-14.4647882728862,
21.9280367100096)) ;
#61001=CARTESIAN_POINT('Ctrl Pts',(-25.8831717248474,-15.0366437072153,
22.0048097991493)) ;
#61002=CARTESIAN_POINT('Ctrl Pts',(-25.9023611320459,-15.0366437072153,
21.9822182825064)) ;
#61003=CARTESIAN_POINT('Ctrl Pts',(-25.9018452635895,-15.0333766937121,
21.9817827114191)) ;
#61004=CARTESIAN_POINT('Ctrl Pts',(-25.9013293415857,-15.0301093422777,
21.9813470954983)) ;
#61005=CARTESIAN_POINT('Ctrl Pts',(-25.8110134109735,-14.4581357186702,
21.90508940013)) ;
#61006=CARTESIAN_POINT('Ctrl Pts',(-25.7195946111273,-13.8792135350187,
21.8279119784973)) ;
#61007=CARTESIAN_POINT('Ctrl Pts',(-25.5345906631916,-12.7077475336248,
21.6717592497823)) ;
#61008=CARTESIAN_POINT('Ctrl Pts',(-25.4410055390766,-12.1152037158853,
21.592783914476)) ;
#61009=CARTESIAN_POINT('Ctrl Pts',(-25.2527389751069,-10.9233053109973,
21.4339497878536)) ;
#61010=CARTESIAN_POINT('Ctrl Pts',(-25.1580575854303,-10.3239507237972,
21.3540909374484)) ;
#61011=CARTESIAN_POINT('Ctrl Pts',(-25.0160140002822,-9.42491891624215,
21.2343279977195)) ;
#61012=CARTESIAN_POINT('Ctrl Pts',(-24.9686625301724,-9.12524166312279,
21.1944112710693)) ;
#61013=CARTESIAN_POINT('Ctrl Pts',(-24.8740854099916,-8.52673854441016,
21.114701471501)) ;
#61014=CARTESIAN_POINT('Ctrl Pts',(-24.826859765719,-8.22791267880993,21.0749083917548)) ;
#61015=CARTESIAN_POINT('Ctrl Pts',(-24.7326668804222,-7.63196369106424,
20.9955615674227)) ;
#61016=CARTESIAN_POINT('Ctrl Pts',(-24.6856996517898,-7.33484056892204,
20.956007808249)) ;
#61017=CARTESIAN_POINT('Ctrl Pts',(-24.5921554552203,-6.74314842492882,
20.8772561612121)) ;
#61018=CARTESIAN_POINT('Ctrl Pts',(-24.5455785122871,-6.44857940304413,
20.8380582439013)) ;
#61019=CARTESIAN_POINT('Ctrl Pts',(-24.4761037454443,-6.00927996429998,
20.779616781815)) ;
#61020=CARTESIAN_POINT('Ctrl Pts',(-24.4530105855386,-5.86327250157364,
20.7601955448585)) ;
#61021=CARTESIAN_POINT('Ctrl Pts',(-24.406970575575,-5.57221536220158,20.7214865668323)) ;
#61022=CARTESIAN_POINT('Ctrl Pts',(-24.3840237262814,-5.42716568555446,
20.7021988248636)) ;
#61023=CARTESIAN_POINT('Ctrl Pts',(-24.3382922419094,-5.13813053770804,
20.6637720840111)) ;
#61024=CARTESIAN_POINT('Ctrl Pts',(-24.3155076110681,-4.994145066511,20.6446330801402)) ;
#61025=CARTESIAN_POINT('Ctrl Pts',(-24.2701161458643,-4.70734474945901,
20.6065194420599)) ;
#61026=CARTESIAN_POINT('Ctrl Pts',(-24.2475093201436,-4.56452990358902,
20.5875447976717)) ;
#61027=CARTESIAN_POINT('Ctrl Pts',(-24.2024885349213,-4.28017725795857,
20.5497761088005)) ;
#61028=CARTESIAN_POINT('Ctrl Pts',(-24.1800745928605,-4.13863945910828,
20.530982044075)) ;
#61029=CARTESIAN_POINT('Ctrl Pts',(-24.1354537656291,-3.85694733014141,
20.4935917802858)) ;
#61030=CARTESIAN_POINT('Ctrl Pts',(-24.1132469192356,-3.71679299994535,
20.474995535545)) ;
#61031=CARTESIAN_POINT('Ctrl Pts',(-24.0801013421189,-3.50767892429782,
20.447263980962)) ;
#61032=CARTESIAN_POINT('Ctrl Pts',(-24.0690802474695,-3.43816046918698,
20.4380472857343)) ;
#61033=CARTESIAN_POINT('Ctrl Pts',(-24.0470941841408,-3.29950933600938,
20.4196709667008)) ;
#61034=CARTESIAN_POINT('Ctrl Pts',(-24.0361292167885,-3.2303766579392,20.4105113413331)) ;
#61035=CARTESIAN_POINT('Ctrl Pts',(-24.0142563188986,-3.09251038320258,
20.3922523367185)) ;
#61036=CARTESIAN_POINT('Ctrl Pts',(-24.0033483986767,-3.02377678654973,
20.3831529453317)) ;
#61037=CARTESIAN_POINT('Ctrl Pts',(-23.9815899152853,-2.88672198054314,
20.365018279184)) ;
#61038=CARTESIAN_POINT('Ctrl Pts',(-23.9707393775487,-2.81840077111661,
20.355982974458)) ;
#61039=CARTESIAN_POINT('Ctrl Pts',(-23.9500412143655,-2.6881396694976,20.3387686940272)) ;
#61040=CARTESIAN_POINT('Ctrl Pts',(-23.9396669651916,-2.62287936210179,
20.33014976239)) ;
#61041=CARTESIAN_POINT('Ctrl Pts',(-23.9237230744987,-2.52265835478894,
20.3169277400514)) ;
#61042=CARTESIAN_POINT('Ctrl Pts',(-23.9183446726732,-2.4888629280703,20.3124714839205)) ;
#61043=CARTESIAN_POINT('Ctrl Pts',(-23.9075207487582,-2.42088369486294,
20.3035140128745)) ;
#61044=CARTESIAN_POINT('Ctrl Pts',(-23.9020752382555,-2.3866998883287,20.2990127843041)) ;
#61045=CARTESIAN_POINT('Ctrl Pts',(-23.8911769857135,-2.31833236638135,
20.2900188698735)) ;
#61046=CARTESIAN_POINT('Ctrl Pts',(-23.8857242745468,-2.28414866463331,
20.2855261520298)) ;
#61047=CARTESIAN_POINT('Ctrl Pts',(-23.8775838646232,-2.23316453895799,
20.2788345944482)) ;
#61048=CARTESIAN_POINT('Ctrl Pts',(-23.8748768256776,-2.21621840162983,
20.2766120090047)) ;
#61049=CARTESIAN_POINT('Ctrl Pts',(-23.8694827328601,-2.18247182679563,
20.2721898202708)) ;
#61050=CARTESIAN_POINT('Ctrl Pts',(-23.8667956804559,-2.16567138928169,
20.2699902152505)) ;
#61051=CARTESIAN_POINT('Ctrl Pts',(-23.8614483991428,-2.13226477295818,
20.2656214375521)) ;
#61052=CARTESIAN_POINT('Ctrl Pts',(-23.8587881823468,-2.11565859798799,
20.2634522518394)) ;
#61053=CARTESIAN_POINT('Ctrl Pts',(-23.8535008795025,-2.08268906932289,
20.2591523894634)) ;
#61054=CARTESIAN_POINT('Ctrl Pts',(-23.850873824714,-2.06632571542302,20.2570216759331)) ;
#61055=CARTESIAN_POINT('Ctrl Pts',(-23.8469619668925,-2.041999222178,20.2538615504348)) ;
#61056=CARTESIAN_POINT('Ctrl Pts',(-23.8456627852911,-2.03392681489554,
20.2528141856382)) ;
#61057=CARTESIAN_POINT('Ctrl Pts',(-23.8430743685028,-2.0178609186655,20.2507329385867)) ;
#61058=CARTESIAN_POINT('Ctrl Pts',(-23.8417851338501,-2.0098674297134,20.2496990557024)) ;
#61059=CARTESIAN_POINT('Ctrl Pts',(-23.8392166571814,-1.99396544383862,
20.2476466569085)) ;
#61060=CARTESIAN_POINT('Ctrl Pts',(-23.8379374338061,-1.9860569470905,20.2466281191092)) ;
#61061=CARTESIAN_POINT('Ctrl Pts',(-23.8360255891411,-1.974262505962,20.2451138867272)) ;
#61062=CARTESIAN_POINT('Ctrl Pts',(-23.8353894649892,-1.97034240968838,
20.244611414041)) ;
#61063=CARTESIAN_POINT('Ctrl Pts',(-23.8341192976822,-1.96252574673243,
20.2436115298626)) ;
#61064=CARTESIAN_POINT('Ctrl Pts',(-23.833485255703,-1.95862918003667,20.2431141169819)) ;
#61065=CARTESIAN_POINT('Ctrl Pts',(-23.8322180529177,-1.95085564685803,
20.242124510617)) ;
#61066=CARTESIAN_POINT('Ctrl Pts',(-23.831551236331,-1.94677214470025,20.2416060093154)) ;
#61067=CARTESIAN_POINT('Ctrl Pts',(-23.8301818626089,-1.93841091783493,
20.2405490838777)) ;
#61068=CARTESIAN_POINT('Ctrl Pts',(-23.8294793527083,-1.93413319244849,
20.2400106039159)) ;
#61069=CARTESIAN_POINT('Ctrl Pts',(-23.8284203074574,-1.92771686730304,
20.2392091844746)) ;
#61070=CARTESIAN_POINT('Ctrl Pts',(-23.8280664036579,-1.92557814934648,
20.238943109163)) ;
#61071=CARTESIAN_POINT('Ctrl Pts',(-23.8273600352524,-1.9213251314707,20.2384170589335)) ;
#61072=CARTESIAN_POINT('Ctrl Pts',(-23.8270075938031,-1.91921083109556,
20.238157056608)) ;
#61073=CARTESIAN_POINT('Ctrl Pts',(-23.8264819338432,-1.91607593159048,
20.2377751864947)) ;
#61074=CARTESIAN_POINT('Ctrl Pts',(-23.8263072072762,-1.91503706074593,
20.2376492614186)) ;
#61075=CARTESIAN_POINT('Ctrl Pts',(-23.8259588939672,-1.91297454696765,
20.2374009304249)) ;
#61076=CARTESIAN_POINT('Ctrl Pts',(-23.8257853088977,-1.91195090399017,
20.2372785225245)) ;
#61077=CARTESIAN_POINT('Ctrl Pts',(-23.8254391507072,-1.90992188988011,
20.2370383481173)) ;
#61078=CARTESIAN_POINT('Ctrl Pts',(-23.8252666033692,-1.908916520574,20.2369205518394)) ;
#61079=CARTESIAN_POINT('Ctrl Pts',(-23.8250078847294,-1.9074244674468,20.2367488447037)) ;
#61080=CARTESIAN_POINT('Ctrl Pts',(-23.8249216558837,-1.90692978371519,
20.2366924478544)) ;
#61081=CARTESIAN_POINT('Ctrl Pts',(-23.8247488849763,-1.90594614016797,
20.2365818500951)) ;
#61082=CARTESIAN_POINT('Ctrl Pts',(-23.8246623585185,-1.90545717970068,
20.2365276306065)) ;
#61083=CARTESIAN_POINT('Ctrl Pts',(-23.8245305246237,-1.90472138440371,
20.2364479563656)) ;
#61084=CARTESIAN_POINT('Ctrl Pts',(-23.8244832305277,-1.90445904599412,
20.2364198914254)) ;
#61085=CARTESIAN_POINT('Ctrl Pts',(-23.8243854245268,-1.90392207855429,
20.2363636264214)) ;
#61086=CARTESIAN_POINT('Ctrl Pts',(-23.8243349158579,-1.90364744934,20.2363354224894)) ;
#61087=CARTESIAN_POINT('Ctrl Pts',(-23.8242321896462,-1.9030985039168,20.236281126385)) ;
#61088=CARTESIAN_POINT('Ctrl Pts',(-23.8241800404489,-1.90282422655538,
20.2362549661509)) ;
#61089=CARTESIAN_POINT('Ctrl Pts',(-23.8239076987598,-1.90163369678401,
20.2361955498099)) ;
#61090=CARTESIAN_POINT('Ctrl Pts',(-23.8238965621088,-1.90158501340151,
20.236193120145)) ;
#61091=CARTESIAN_POINT('Ctrl Pts',(-23.8238854254577,-1.90153633001901,
20.23619069048)) ;
#61092=CARTESIAN_POINT('',(-32.7305102571637,-15.0366437072153,9.10296276716422)) ;
#61093=CARTESIAN_POINT('',(-32.738440159828,-15.0366437072153,9.0744018390217)) ;
#61094=CARTESIAN_POINT('Origin',(1.31615393895547,-21.6462763158694,-0.365428342349787)) ;
#61095=CARTESIAN_POINT('',(-30.1189287239454,-1.90153624313405,8.36247940662196)) ;
#61096=CARTESIAN_POINT('Ctrl Pts',(-30.1189287421105,-1.90153633469768,
8.3624794119278)) ;
#61097=CARTESIAN_POINT('Ctrl Pts',(-30.1189366899314,-1.90158489287906,
8.36248829647417)) ;
#61098=CARTESIAN_POINT('Ctrl Pts',(-30.1190728896525,-1.90241702169426,
8.36264054861436)) ;
#61099=CARTESIAN_POINT('Ctrl Pts',(-30.1191458040911,-1.90281621613969,
8.36268630250738)) ;
#61100=CARTESIAN_POINT('Ctrl Pts',(-30.1191963902888,-1.9030887682969,8.36271464737924)) ;
#61101=CARTESIAN_POINT('Ctrl Pts',(-30.1192983133845,-1.90363426309853,
8.36276893498663)) ;
#61102=CARTESIAN_POINT('Ctrl Pts',(-30.1193496681974,-1.90390716693057,
8.362794783217)) ;
#61103=CARTESIAN_POINT('Ctrl Pts',(-30.1194504713046,-1.90444076192566,
8.36284391234841)) ;
#61104=CARTESIAN_POINT('Ctrl Pts',(-30.1194999210193,-1.90470145327792,
8.36286718827989)) ;
#61105=CARTESIAN_POINT('Ctrl Pts',(-30.1196389419315,-1.90543258195801,
8.36293125926836)) ;
#61106=CARTESIAN_POINT('Ctrl Pts',(-30.1197317682973,-1.90591842510436,
8.3629722308881)) ;
#61107=CARTESIAN_POINT('Ctrl Pts',(-30.1199190407705,-1.9068957977074,8.36305273288145)) ;
#61108=CARTESIAN_POINT('Ctrl Pts',(-30.1200134934398,-1.90738732781205,
8.36309224012143)) ;
#61109=CARTESIAN_POINT('Ctrl Pts',(-30.1202989406533,-1.90886986923223,
8.36320937923951)) ;
#61110=CARTESIAN_POINT('Ctrl Pts',(-30.1204920133598,-1.90986882963001,
8.36328566672494)) ;
#61111=CARTESIAN_POINT('Ctrl Pts',(-30.120882522362,-1.91188490974371,8.36343655309822)) ;
#61112=CARTESIAN_POINT('Ctrl Pts',(-30.1210799687811,-1.91290202763325,
8.36351111411351)) ;
#61113=CARTESIAN_POINT('Ctrl Pts',(-30.121478391718,-1.914951394423,8.36365921021491)) ;
#61114=CARTESIAN_POINT('Ctrl Pts',(-30.1216793689211,-1.91598364336599,
8.36373274286551)) ;
#61115=CARTESIAN_POINT('Ctrl Pts',(-30.1222864955005,-1.91909856098391,
8.36395226839086)) ;
#61116=CARTESIAN_POINT('Ctrl Pts',(-30.1226968244005,-1.92119938519643,
8.36409723269177)) ;
#61117=CARTESIAN_POINT('Ctrl Pts',(-30.1235232857103,-1.92542529583428,
8.36438500090773)) ;
#61118=CARTESIAN_POINT('Ctrl Pts',(-30.1239394277851,-1.92755038271577,
8.36452777036499)) ;
#61119=CARTESIAN_POINT('Ctrl Pts',(-30.1251889974469,-1.9339258146116,8.36495209273466)) ;
#61120=CARTESIAN_POINT('Ctrl Pts',(-30.1260235402243,-1.93817627781002,
8.36522972038847)) ;
#61121=CARTESIAN_POINT('Ctrl Pts',(-30.127656279388,-1.94648421945793,8.36576680755742)) ;
#61122=CARTESIAN_POINT('Ctrl Pts',(-30.1284544954223,-1.95054169858679,
8.36602619683147)) ;
#61123=CARTESIAN_POINT('Ctrl Pts',(-30.1299748675873,-1.95826546921425,
8.36651673549711)) ;
#61124=CARTESIAN_POINT('Ctrl Pts',(-30.1307374247382,-1.96213697914807,
8.36676089979701)) ;
#61125=CARTESIAN_POINT('Ctrl Pts',(-30.1322678626644,-1.96990337734099,
8.36724811362133)) ;
#61126=CARTESIAN_POINT('Ctrl Pts',(-30.1330357439221,-1.97379826561344,
8.36749116141787)) ;
#61127=CARTESIAN_POINT('Ctrl Pts',(-30.1353469300952,-1.98551686319814,
8.36821935177273)) ;
#61128=CARTESIAN_POINT('Ctrl Pts',(-30.1368977646678,-1.99337450486331,
8.36870358687115)) ;
#61129=CARTESIAN_POINT('Ctrl Pts',(-30.1400176319817,-2.00917423416183,
8.3696717456377)) ;
#61130=CARTESIAN_POINT('Ctrl Pts',(-30.1415866723529,-2.01711632162066,
8.37015564168992)) ;
#61131=CARTESIAN_POINT('Ctrl Pts',(-30.1447413894306,-2.03307890748333,
8.37112408567312)) ;
#61132=CARTESIAN_POINT('Ctrl Pts',(-30.1463270663545,-2.04109940589163,
8.37160863282255)) ;
#61133=CARTESIAN_POINT('Ctrl Pts',(-30.1511069097881,-2.06526946998702,
8.37306397729435)) ;
#61134=CARTESIAN_POINT('Ctrl Pts',(-30.1543238610328,-2.08152760108453,
8.37403657554525)) ;
#61135=CARTESIAN_POINT('Ctrl Pts',(-30.1608078860201,-2.11428512297351,
8.37598761435187)) ;
#61136=CARTESIAN_POINT('Ctrl Pts',(-30.1640749726964,-2.13078451396997,
8.37696600848241)) ;
#61137=CARTESIAN_POINT('Ctrl Pts',(-30.1706491258843,-2.16397631340779,
8.37892790365587)) ;
#61138=CARTESIAN_POINT('Ctrl Pts',(-30.1739561963703,-2.18066871801029,
8.37991138741871)) ;
#61139=CARTESIAN_POINT('Ctrl Pts',(-30.1806003831165,-2.21419829031838,
8.38188196581156)) ;
#61140=CARTESIAN_POINT('Ctrl Pts',(-30.1839374999802,-2.23103545803188,
8.38286905827254)) ;
#61141=CARTESIAN_POINT('Ctrl Pts',(-30.1939791862586,-2.28169173815909,
8.38583291307417)) ;
#61142=CARTESIAN_POINT('Ctrl Pts',(-30.2007140718881,-2.31565562726959,
8.38781232274202)) ;
#61143=CARTESIAN_POINT('Ctrl Pts',(-30.2141868277967,-2.38358352393428,
8.39176048383652)) ;
#61144=CARTESIAN_POINT('Ctrl Pts',(-30.2209247071832,-2.41754751782455,
8.39372919190598)) ;
#61145=CARTESIAN_POINT('Ctrl Pts',(-30.234326067002,-2.48508962361059,8.3976364844371)) ;
#61146=CARTESIAN_POINT('Ctrl Pts',(-30.2409895522187,-2.51866773555189,
8.39957505170218)) ;
#61147=CARTESIAN_POINT('Ctrl Pts',(-30.2607526662601,-2.61824429213986,
8.40531520776665)) ;
#61148=CARTESIAN_POINT('Ctrl Pts',(-30.2736249224652,-2.68308495719539,
8.40904136225151)) ;
#61149=CARTESIAN_POINT('Ctrl Pts',(-30.2993135315686,-2.81246585171732,
8.41646293757522)) ;
#61150=CARTESIAN_POINT('Ctrl Pts',(-30.312785289604,-2.88030501170083,8.42034614576319)) ;
#61151=CARTESIAN_POINT('Ctrl Pts',(-30.339813448705,-3.01639280924263,8.42812401692986)) ;
#61152=CARTESIAN_POINT('Ctrl Pts',(-30.3533698602386,-3.0846414468735,8.43201864226201)) ;
#61153=CARTESIAN_POINT('Ctrl Pts',(-30.3805639776459,-3.22153498784917,
8.43982120276864)) ;
#61154=CARTESIAN_POINT('Ctrl Pts',(-30.394201687757,-3.29017989118037,8.44372912266984)) ;
#61155=CARTESIAN_POINT('Ctrl Pts',(-30.4215552917968,-3.42785275302243,
8.45155927059217)) ;
#61156=CARTESIAN_POINT('Ctrl Pts',(-30.4352711862702,-3.49688071153673,
8.45548149664984)) ;
#61157=CARTESIAN_POINT('Ctrl Pts',(-30.4765316882847,-3.70451935539514,
8.46727038395918)) ;
#61158=CARTESIAN_POINT('Ctrl Pts',(-30.5041890851405,-3.84368480840043,
8.47515935928979)) ;
#61159=CARTESIAN_POINT('Ctrl Pts',(-30.5597818551889,-4.12338942184984,
8.4909972851407)) ;
#61160=CARTESIAN_POINT('Ctrl Pts',(-30.58771724435,-4.26392858237327,8.49894617820889)) ;
#61161=CARTESIAN_POINT('Ctrl Pts',(-30.6438439166593,-4.54627494106967,
8.5149018456369)) ;
#61162=CARTESIAN_POINT('Ctrl Pts',(-30.6720352067423,-4.68808213833386,
8.52290859431798)) ;
#61163=CARTESIAN_POINT('Ctrl Pts',(-30.7286519494228,-4.97285889875352,
8.53897661380741)) ;
#61164=CARTESIAN_POINT('Ctrl Pts',(-30.7570774055805,-5.11582846192401,
8.54703787180537)) ;
#61165=CARTESIAN_POINT('Ctrl Pts',(-30.8141409569631,-5.40282428515253,
8.56321080365312)) ;
#61166=CARTESIAN_POINT('Ctrl Pts',(-30.8427790539311,-5.54685054520825,
8.57132247122268)) ;
#61167=CARTESIAN_POINT('Ctrl Pts',(-30.9002464954105,-5.83585409368823,
8.58759164117081)) ;
#61168=CARTESIAN_POINT('Ctrl Pts',(-30.9290758402359,-5.98083138211383,
8.59574914241628)) ;
#61169=CARTESIAN_POINT('Ctrl Pts',(-31.0158187876865,-6.41703128767462,
8.62028306277105)) ;
#61170=CARTESIAN_POINT('Ctrl Pts',(-31.0739872819299,-6.70952194040057,
8.63672097178661)) ;
#61171=CARTESIAN_POINT('Ctrl Pts',(-31.1908342051894,-7.29703932551894,
8.66971923040377)) ;
#61172=CARTESIAN_POINT('Ctrl Pts',(-31.2495126445056,-7.59206605794504,
8.68627954293313)) ;
#61173=CARTESIAN_POINT('Ctrl Pts',(-31.3672102153851,-8.18381025254895,
8.7194791528873)) ;
#61174=CARTESIAN_POINT('Ctrl Pts',(-31.4262293520484,-8.48052771472347,
8.73611843194019)) ;
#61175=CARTESIAN_POINT('Ctrl Pts',(-31.5444393691136,-9.07480801972223,
8.7694314609245)) ;
#61176=CARTESIAN_POINT('Ctrl Pts',(-31.6036302519042,-9.37237086255337,
8.78610520225537)) ;
#61177=CARTESIAN_POINT('Ctrl Pts',(-31.7812073724757,-10.26505943922,8.83611035606427)) ;
#61178=CARTESIAN_POINT('Ctrl Pts',(-31.89959803729,-10.8601852058064,8.86942584909673)) ;
#61179=CARTESIAN_POINT('Ctrl Pts',(-32.13504239898,-12.0436740242095,8.93564812637502)) ;
#61180=CARTESIAN_POINT('Ctrl Pts',(-32.2520961165265,-12.6320370760777,
8.96855483620709)) ;
#61181=CARTESIAN_POINT('Ctrl Pts',(-32.4835188253346,-13.7952376552548,
9.03358962841841)) ;
#61182=CARTESIAN_POINT('Ctrl Pts',(-32.6047730141693,-14.40468127544,9.06765183250815)) ;
#61183=CARTESIAN_POINT('Ctrl Pts',(-32.7237611936004,-15.002722575796,9.1010674510721)) ;
#61184=CARTESIAN_POINT('Ctrl Pts',(-32.7305102570438,-15.0366437072151,
9.1029627675952)) ;
#61185=CARTESIAN_POINT('Ctrl Pts',(-32.738440159947,-15.0366437072151,9.07440183859236)) ;
#61186=CARTESIAN_POINT('Ctrl Pts',(-32.7316800387762,-15.0027225758828,
9.07254634847045)) ;
#61187=CARTESIAN_POINT('Ctrl Pts',(-32.7249124353925,-14.9687639420613,
9.07068883708644)) ;
#61188=CARTESIAN_POINT('Ctrl Pts',(-32.6055998276366,-14.3700751829105,
9.03794155762668)) ;
#61189=CARTESIAN_POINT('Ctrl Pts',(-32.4910381898364,-13.7952376556947,
9.0065073254432)) ;
#61190=CARTESIAN_POINT('Ctrl Pts',(-32.2592130431272,-12.6320370767004,
8.94292198369549)) ;
#61191=CARTESIAN_POINT('Ctrl Pts',(-32.141949544088,-12.0436740249246,8.91077083858567)) ;
#61192=CARTESIAN_POINT('Ctrl Pts',(-31.9060662027409,-10.8601852067075,
8.84612962328421)) ;
#61193=CARTESIAN_POINT('Ctrl Pts',(-31.7874463810849,-10.2650594402146,
8.81363947867534)) ;
#61194=CARTESIAN_POINT('Ctrl Pts',(-31.6095078011031,-9.3723708636882,8.76493618411246)) ;
#61195=CARTESIAN_POINT('Ctrl Pts',(-31.5501934567731,-9.0748080209038,8.74870711109432)) ;
#61196=CARTESIAN_POINT('Ctrl Pts',(-31.4317296947875,-8.48052771599843,
8.71630798878961)) ;
#61197=CARTESIAN_POINT('Ctrl Pts',(-31.3725802795186,-8.18381025387053,
8.70013793090298)) ;
#61198=CARTESIAN_POINT('Ctrl Pts',(-31.254614084343,-7.59206605935958,8.66790581829583)) ;
#61199=CARTESIAN_POINT('Ctrl Pts',(-31.1957973095379,-7.29703932697985,
8.65184374520358)) ;
#61200=CARTESIAN_POINT('Ctrl Pts',(-31.0786638053382,-6.70952194195379,
8.61987765791991)) ;
#61201=CARTESIAN_POINT('Ctrl Pts',(-31.0203470862311,-6.4170312892738,8.60397360665013)) ;
#61202=CARTESIAN_POINT('Ctrl Pts',(-30.9333722119693,-5.98083138378153,
8.58027501122829)) ;
#61203=CARTESIAN_POINT('Ctrl Pts',(-30.9044639497444,-5.83585409537872,
8.5724017447851)) ;
#61204=CARTESIAN_POINT('Ctrl Pts',(-30.846834926806,-5.54685054694414,8.55671453869105)) ;
#61205=CARTESIAN_POINT('Ctrl Pts',(-30.8181141664073,-5.40282428691104,
8.54890059790883)) ;
#61206=CARTESIAN_POINT('Ctrl Pts',(-30.7608808355205,-5.11582846372763,
8.53333915660507)) ;
#61207=CARTESIAN_POINT('Ctrl Pts',(-30.7323682667758,-4.97285890057961,
8.52559164980705)) ;
#61208=CARTESIAN_POINT('Ctrl Pts',(-30.6755718751027,-4.68808214020468,
8.51017066754581)) ;
#61209=CARTESIAN_POINT('Ctrl Pts',(-30.647288055729,-4.54627494296275,8.50249717926813)) ;
#61210=CARTESIAN_POINT('Ctrl Pts',(-30.590969507909,-4.26392858431071,8.48723258500705)) ;
#61211=CARTESIAN_POINT('Ctrl Pts',(-30.5629347867595,-4.12338942380938,
8.47964145344446)) ;
#61212=CARTESIAN_POINT('Ctrl Pts',(-30.5071344190471,-3.84368481040393,
8.46455122683816)) ;
#61213=CARTESIAN_POINT('Ctrl Pts',(-30.4793687884229,-3.70451935742048,
8.45705207432742)) ;
#61214=CARTESIAN_POINT('Ctrl Pts',(-30.4379366248619,-3.49688071359469,
8.44588145605661)) ;
#61215=CARTESIAN_POINT('Ctrl Pts',(-30.4241619434822,-3.42785275509126,
8.44217096130755)) ;
#61216=CARTESIAN_POINT('Ctrl Pts',(-30.3966869486075,-3.29017989327082,
8.4347780236757)) ;
#61217=CARTESIAN_POINT('Ctrl Pts',(-30.3829866356556,-3.2215349899504,8.4310955788379)) ;
#61218=CARTESIAN_POINT('Ctrl Pts',(-30.3556625208449,-3.08464144899626,
8.42376122667959)) ;
#61219=CARTESIAN_POINT('Ctrl Pts',(-30.3420387232273,-3.01639281137611,
8.42010930409529)) ;
#61220=CARTESIAN_POINT('Ctrl Pts',(-30.3148695396667,-2.88030501385569,
8.41283935714398)) ;
#61221=CARTESIAN_POINT('Ctrl Pts',(-30.301324164162,-2.81246585388284,8.40922129512537)) ;
#61222=CARTESIAN_POINT('Ctrl Pts',(-30.2754864732429,-2.68308495896682,
8.4023366636702)) ;
#61223=CARTESIAN_POINT('Ctrl Pts',(-30.2625357547394,-2.61824429348635,
8.39889310451541)) ;
#61224=CARTESIAN_POINT('Ctrl Pts',(-30.2426422289194,-2.51866773624582,
8.39362264872344)) ;
#61225=CARTESIAN_POINT('Ctrl Pts',(-30.2359331379167,-2.48508962408448,
8.39184833848451)) ;
#61226=CARTESIAN_POINT('Ctrl Pts',(-30.2224356667615,-2.4175475178558,8.38828720735983)) ;
#61227=CARTESIAN_POINT('Ctrl Pts',(-30.2156472913765,-2.38358352374292,
8.38650036926848)) ;
#61228=CARTESIAN_POINT('Ctrl Pts',(-30.2020675740235,-2.31565562663307,
8.38293744813557)) ;
#61229=CARTESIAN_POINT('Ctrl Pts',(-30.1952762466078,-2.28169173729999,
8.38116132323752)) ;
#61230=CARTESIAN_POINT('Ctrl Pts',(-30.1851439288179,-2.23103545684079,
8.37852389338254)) ;
#61231=CARTESIAN_POINT('Ctrl Pts',(-30.1817755969363,-2.21419828901697,
8.37764922716979)) ;
#61232=CARTESIAN_POINT('Ctrl Pts',(-30.1750665385079,-2.18066871648915,
8.37591229529037)) ;
#61233=CARTESIAN_POINT('Ctrl Pts',(-30.171725812564,-2.16397631177722,8.37505002744728)) ;
#61234=CARTESIAN_POINT('Ctrl Pts',(-30.16508123956,-2.13078451212187,8.37334176136098)) ;
#61235=CARTESIAN_POINT('Ctrl Pts',(-30.1617773979994,-2.11428512101739,
8.3724957462761)) ;
#61236=CARTESIAN_POINT('Ctrl Pts',(-30.1552156490333,-2.08152759891375,
8.37082464377552)) ;
#61237=CARTESIAN_POINT('Ctrl Pts',(-30.1519577544726,-2.06526946770973,
8.36999950993898)) ;
#61238=CARTESIAN_POINT('Ctrl Pts',(-30.1471118028374,-2.04109940345594,
8.36878226556815)) ;
#61239=CARTESIAN_POINT('Ctrl Pts',(-30.1455032940284,-2.03307890499497,
8.36837995139651)) ;
#61240=CARTESIAN_POINT('Ctrl Pts',(-30.1423008670093,-2.01711631902769,
8.36758334301117)) ;
#61241=CARTESIAN_POINT('Ctrl Pts',(-30.1407069490228,-2.00917423151679,
8.36718904799129)) ;
#61242=CARTESIAN_POINT('Ctrl Pts',(-30.1375345303182,-1.99337450211475,
8.36641016214816)) ;
#61243=CARTESIAN_POINT('Ctrl Pts',(-30.1359560372963,-1.98551686039824,
8.3660255437412)) ;
#61244=CARTESIAN_POINT('Ctrl Pts',(-30.1336002594764,-1.97379826273675,
8.36545795792382)) ;
#61245=CARTESIAN_POINT('Ctrl Pts',(-30.1328169906812,-1.96990337443867,
8.36527033100878)) ;
#61246=CARTESIAN_POINT('Ctrl Pts',(-30.1312544389846,-1.96213697619486,
8.36489878049294)) ;
#61247=CARTESIAN_POINT('Ctrl Pts',(-30.1304751565699,-1.95826546623556,
8.36471485512932)) ;
#61248=CARTESIAN_POINT('Ctrl Pts',(-30.1289195156902,-1.95054169571453,
8.36435134297619)) ;
#61249=CARTESIAN_POINT('Ctrl Pts',(-30.1281018294351,-1.94648421672414,
8.36416207920644)) ;
#61250=CARTESIAN_POINT('Ctrl Pts',(-30.1264259078607,-1.93817627535945,
8.36378052124339)) ;
#61251=CARTESIAN_POINT('Ctrl Pts',(-30.1255676919097,-1.9339258123061,8.36358815676693)) ;
#61252=CARTESIAN_POINT('Ctrl Pts',(-30.1242782281864,-1.9275503806276,8.363307519989)) ;
#61253=CARTESIAN_POINT('Ctrl Pts',(-30.1238480485303,-1.9254252938187,8.36321530938629)) ;
#61254=CARTESIAN_POINT('Ctrl Pts',(-30.122991529241,-1.92119938332494,8.36303580033953)) ;
#61255=CARTESIAN_POINT('Ctrl Pts',(-30.1225651990868,-1.91909855918412,
8.36294846740335)) ;
#61256=CARTESIAN_POINT('Ctrl Pts',(-30.1219318011106,-1.91598364167241,
8.36282356297935)) ;
#61257=CARTESIAN_POINT('Ctrl Pts',(-30.1217216823121,-1.91495139276497,
8.36278295540766)) ;
#61258=CARTESIAN_POINT('Ctrl Pts',(-30.121303939256,-1.91290202604524,8.36270444414061)) ;
#61259=CARTESIAN_POINT('Ctrl Pts',(-30.1210963156627,-1.91188490819044,
8.36266653802089)) ;
#61260=CARTESIAN_POINT('Ctrl Pts',(-30.1206839151831,-1.90986882814559,
8.36259449767639)) ;
#61261=CARTESIAN_POINT('Ctrl Pts',(-30.1204791491518,-1.90886986778167,
8.3625603257668)) ;
#61262=CARTESIAN_POINT('Ctrl Pts',(-30.1201741701421,-1.90738732641242,
8.36251353386047)) ;
#61263=CARTESIAN_POINT('Ctrl Pts',(-30.1200728696049,-1.90689579632289,
8.36249869042318)) ;
#61264=CARTESIAN_POINT('Ctrl Pts',(-30.1198709007348,-1.90591842375347,
8.36247112009354)) ;
#61265=CARTESIAN_POINT('Ctrl Pts',(-30.119770238727,-1.90543258062349,8.36245836991853)) ;
#61266=CARTESIAN_POINT('Ctrl Pts',(-30.1196180856502,-1.9047014521107,8.3624415968411)) ;
#61267=CARTESIAN_POINT('Ctrl Pts',(-30.1195637143114,-1.90444076092128,
8.36243604712368)) ;
#61268=CARTESIAN_POINT('Ctrl Pts',(-30.1194520118001,-1.90390716624985,
8.36242617434808)) ;
#61269=CARTESIAN_POINT('Ctrl Pts',(-30.1193946819637,-1.90363426257986,
8.3624218463327)) ;
#61270=CARTESIAN_POINT('Ctrl Pts',(-30.119279360318,-1.90308876810775,8.36241581619551)) ;
#61271=CARTESIAN_POINT('Ctrl Pts',(-30.1192214019085,-1.90281621611284,
8.36241402375624)) ;
#61272=CARTESIAN_POINT('Ctrl Pts',(-30.1189510053552,-1.90163369796138,
8.36247443771244)) ;
#61273=CARTESIAN_POINT('Ctrl Pts',(-30.1189398737328,-1.90158501632953,
8.36247692482012)) ;
#61274=CARTESIAN_POINT('Ctrl Pts',(-30.1189287421105,-1.90153633469768,
8.3624794119278)) ;
#61275=CARTESIAN_POINT('',(-33.5276414405313,-15.0366437072153,-5.48155929182975)) ;
#61276=CARTESIAN_POINT('',(-33.5228460028119,-15.0366437072153,-5.51081016788253)) ;
#61277=CARTESIAN_POINT('Origin',(1.34794834185301,-21.6462763158694,0.220984913775247)) ;
#61278=CARTESIAN_POINT('',(-30.8465133415523,-1.9015362431713,-5.057029164855)) ;
#61279=CARTESIAN_POINT('Ctrl Pts',(-30.8465133602742,-1.90153633477217,
-5.05702916766694)) ;
#61280=CARTESIAN_POINT('Ctrl Pts',(-30.846524305277,-1.90158489180048,-5.05702443248837)) ;
#61281=CARTESIAN_POINT('Ctrl Pts',(-30.8467113041087,-1.9024145039777,-5.05694353046583)) ;
#61282=CARTESIAN_POINT('Ctrl Pts',(-30.8467964485072,-1.90281253800259,
-5.05693261829815)) ;
#61283=CARTESIAN_POINT('Ctrl Pts',(-30.8468540962568,-1.90308429852864,
-5.05692812744458)) ;
#61284=CARTESIAN_POINT('Ctrl Pts',(-30.8469690650942,-1.90362820994333,
-5.05692163693397)) ;
#61285=CARTESIAN_POINT('Ctrl Pts',(-30.8470263627717,-1.90390032204335,
-5.05691973052414)) ;
#61286=CARTESIAN_POINT('Ctrl Pts',(-30.8471381575833,-1.90443236952265,
-5.05691744581171)) ;
#61287=CARTESIAN_POINT('Ctrl Pts',(-30.8471926539434,-1.90469230508585,
-5.05691707246499)) ;
#61288=CARTESIAN_POINT('Ctrl Pts',(-30.8473452861646,-1.90542129310748,
-5.05691726094962)) ;
#61289=CARTESIAN_POINT('Ctrl Pts',(-30.8474464415333,-1.90590570652529,
-5.05691902657438)) ;
#61290=CARTESIAN_POINT('Ctrl Pts',(-30.8476496141687,-1.90688020302458,
-5.05692454286342)) ;
#61291=CARTESIAN_POINT('Ctrl Pts',(-30.847751627679,-1.90737028675471,-5.0569283172706)) ;
#61292=CARTESIAN_POINT('Ctrl Pts',(-30.8480589795514,-1.90884846572905,
-5.05694176855341)) ;
#61293=CARTESIAN_POINT('Ctrl Pts',(-30.8482656351864,-1.90984448674729,
-5.05695353474426)) ;
#61294=CARTESIAN_POINT('Ctrl Pts',(-30.8486821875314,-1.9118546348179,-5.05698042595716)) ;
#61295=CARTESIAN_POINT('Ctrl Pts',(-30.8488920775291,-1.91286876004502,
-5.0569955895894)) ;
#61296=CARTESIAN_POINT('Ctrl Pts',(-30.8493146220058,-1.91491209710514,
-5.0570283257827)) ;
#61297=CARTESIAN_POINT('Ctrl Pts',(-30.8495272760765,-1.91594130898178,
-5.05704590088905)) ;
#61298=CARTESIAN_POINT('Ctrl Pts',(-30.8501685848949,-1.91904706211498,
-5.05710135597619)) ;
#61299=CARTESIAN_POINT('Ctrl Pts',(-30.8506005906325,-1.9211417056253,-5.05714191950652)) ;
#61300=CARTESIAN_POINT('Ctrl Pts',(-30.8514689484867,-1.9253551838102,-5.05722743644029)) ;
#61301=CARTESIAN_POINT('Ctrl Pts',(-30.85190529492,-1.92747401894057,-5.05727242509241)) ;
#61302=CARTESIAN_POINT('Ctrl Pts',(-30.8532136992813,-1.93383069557251,
-5.05741148274527)) ;
#61303=CARTESIAN_POINT('Ctrl Pts',(-30.8540851221337,-1.93806865525155,
-5.05750957649476)) ;
#61304=CARTESIAN_POINT('Ctrl Pts',(-30.8557874699047,-1.94635215818821,
-5.05770699916352)) ;
#61305=CARTESIAN_POINT('Ctrl Pts',(-30.8566183831832,-1.95039770212494,
-5.05780639995181)) ;
#61306=CARTESIAN_POINT('Ctrl Pts',(-30.8581995372407,-1.95809865038701,
-5.05799892058496)) ;
#61307=CARTESIAN_POINT('Ctrl Pts',(-30.8589917862104,-1.96195866901122,
-5.0580971745769)) ;
#61308=CARTESIAN_POINT('Ctrl Pts',(-30.8605806341267,-1.96970201522502,
-5.05829692357479)) ;
#61309=CARTESIAN_POINT('Ctrl Pts',(-30.8613772327858,-1.97358534282792,
-5.05839842034979)) ;
#61310=CARTESIAN_POINT('Ctrl Pts',(-30.8637734540801,-1.98526915772027,
-5.0587069348275)) ;
#61311=CARTESIAN_POINT('Ctrl Pts',(-30.8653795095856,-1.99310347667916,
-5.05891793007803)) ;
#61312=CARTESIAN_POINT('Ctrl Pts',(-30.8686079562012,-2.00885630997501,
-5.05934782834555)) ;
#61313=CARTESIAN_POINT('Ctrl Pts',(-30.8702303426481,-2.01677482413742,
-5.05956675958315)) ;
#61314=CARTESIAN_POINT('Ctrl Pts',(-30.8734904414554,-2.03269003071707,
-5.06001100244198)) ;
#61315=CARTESIAN_POINT('Ctrl Pts',(-30.8751281536876,-2.04068672313867,
-5.06023631484786)) ;
#61316=CARTESIAN_POINT('Ctrl Pts',(-30.8800626450534,-2.06478504708697,
-5.06092026785506)) ;
#61317=CARTESIAN_POINT('Ctrl Pts',(-30.8833807945906,-2.08099492183752,
-5.06138682384106)) ;
#61318=CARTESIAN_POINT('Ctrl Pts',(-30.8900648925976,-2.11365521506201,
-5.06233564397943)) ;
#61319=CARTESIAN_POINT('Ctrl Pts',(-30.8934308333245,-2.1301056337409,-5.0628179556211)) ;
#61320=CARTESIAN_POINT('Ctrl Pts',(-30.9002010284063,-2.16319891576677,
-5.06379470349268)) ;
#61321=CARTESIAN_POINT('Ctrl Pts',(-30.9036052791168,-2.17984177527506,
-5.0642891570483)) ;
#61322=CARTESIAN_POINT('Ctrl Pts',(-30.9104424789968,-2.21327182781219,
-5.0652873818654)) ;
#61323=CARTESIAN_POINT('Ctrl Pts',(-30.9138754278022,-2.23005902084895,
-5.06579115535564)) ;
#61324=CARTESIAN_POINT('Ctrl Pts',(-30.924202802114,-2.28056494736301,-5.06731285165701)) ;
#61325=CARTESIAN_POINT('Ctrl Pts',(-30.9311257671805,-2.31442802795414,
-5.06834107877602)) ;
#61326=CARTESIAN_POINT('Ctrl Pts',(-30.94496993347,-2.38215430757668,-5.07040844327922)) ;
#61327=CARTESIAN_POINT('Ctrl Pts',(-30.951891124766,-2.41601749294468,-5.07144762376045)) ;
#61328=CARTESIAN_POINT('Ctrl Pts',(-30.9656535719189,-2.48335912723555,
-5.07352210987511)) ;
#61329=CARTESIAN_POINT('Ctrl Pts',(-30.972494824902,-2.51683757620396,-5.07455743309499)) ;
#61330=CARTESIAN_POINT('Ctrl Pts',(-30.9927812370883,-2.61611858052478,
-5.07763660537817)) ;
#61331=CARTESIAN_POINT('Ctrl Pts',(-31.0059890681356,-2.68076679293773,
-5.07965354311224)) ;
#61332=CARTESIAN_POINT('Ctrl Pts',(-31.0323372989951,-2.80974421399637,
-5.08369123789235)) ;
#61333=CARTESIAN_POINT('Ctrl Pts',(-31.0461493683562,-2.87736250066609,
-5.08581643560629)) ;
#61334=CARTESIAN_POINT('Ctrl Pts',(-31.0738548685374,-3.01300721842185,
-5.09009190871467)) ;
#61335=CARTESIAN_POINT('Ctrl Pts',(-31.087748293069,-3.08103364958037,-5.09224222256004)) ;
#61336=CARTESIAN_POINT('Ctrl Pts',(-31.1156142511499,-3.21748148745996,
-5.0965648454186)) ;
#61337=CARTESIAN_POINT('Ctrl Pts',(-31.129586782141,-3.28590289416745,-5.09873717001806)) ;
#61338=CARTESIAN_POINT('Ctrl Pts',(-31.1576085574405,-3.42312751561677,
-5.10310160741578)) ;
#61339=CARTESIAN_POINT('Ctrl Pts',(-31.1716578014195,-3.49193073036205,
-5.10529372222149)) ;
#61340=CARTESIAN_POINT('Ctrl Pts',(-31.2139168843255,-3.69889333670347,
-5.11189720543959)) ;
#61341=CARTESIAN_POINT('Ctrl Pts',(-31.2422380916696,-3.83760568975149,
-5.11633560537967)) ;
#61342=CARTESIAN_POINT('Ctrl Pts',(-31.2991570663195,-4.11639963076904,
-5.12527451457136)) ;
#61343=CARTESIAN_POINT('Ctrl Pts',(-31.3277548240148,-4.25648121881785,
-5.12977508254569)) ;
#61344=CARTESIAN_POINT('Ctrl Pts',(-31.3852060477396,-4.53790830408714,
-5.13883097478029)) ;
#61345=CARTESIAN_POINT('Ctrl Pts',(-31.41405950929,-4.67925380039948,-5.14338632520198)) ;
#61346=CARTESIAN_POINT('Ctrl Pts',(-31.4720010766913,-4.96310337447864,
-5.1525457224151)) ;
#61347=CARTESIAN_POINT('Ctrl Pts',(-31.5010891803993,-5.10560745226049,
-5.15714978229708)) ;
#61348=CARTESIAN_POINT('Ctrl Pts',(-31.55947884342,-5.39166886431443,-5.16640130243607)) ;
#61349=CARTESIAN_POINT('Ctrl Pts',(-31.5887804016795,-5.53522619858423,
-5.17104876911307)) ;
#61350=CARTESIAN_POINT('Ctrl Pts',(-31.6475757056389,-5.82328879913435,
-5.18038229220635)) ;
#61351=CARTESIAN_POINT('Ctrl Pts',(-31.6770694511483,-5.96779406541603,
-5.1850683497823)) ;
#61352=CARTESIAN_POINT('Ctrl Pts',(-31.7658069889186,-6.40257377606671,
-5.19917766558687)) ;
#61353=CARTESIAN_POINT('Ctrl Pts',(-31.825307093791,-6.69411212755049,-5.20865199154413)) ;
#61354=CARTESIAN_POINT('Ctrl Pts',(-31.944819839875,-7.27971665323027,-5.2277033319237)) ;
#61355=CARTESIAN_POINT('Ctrl Pts',(-32.0048324748802,-7.57378282745991,
-5.23728038424542)) ;
#61356=CARTESIAN_POINT('Ctrl Pts',(-32.1251989946871,-8.16360040103258,
-5.25650565117136)) ;
#61357=CARTESIAN_POINT('Ctrl Pts',(-32.1855528764093,-8.45935180037231,
-5.26615388455479)) ;
#61358=CARTESIAN_POINT('Ctrl Pts',(-32.306430425885,-9.05169722737876,-5.28549106947084)) ;
#61359=CARTESIAN_POINT('Ctrl Pts',(-32.3669540921975,-9.34829125505241,
-5.29518002979795)) ;
#61360=CARTESIAN_POINT('Ctrl Pts',(-32.5485224061834,-10.2380733862356,
-5.32426334980075)) ;
#61361=CARTESIAN_POINT('Ctrl Pts',(-32.6695643911593,-10.8312615224899,
-5.34367399302085)) ;
#61362=CARTESIAN_POINT('Ctrl Pts',(-32.9102678483355,-12.0108970987381,
-5.38230551988749)) ;
#61363=CARTESIAN_POINT('Ctrl Pts',(-33.0299293080724,-12.5973445387836,
-5.40152647961662)) ;
#61364=CARTESIAN_POINT('Ctrl Pts',(-33.2664976872741,-13.756757931353,-5.43954920009931)) ;
#61365=CARTESIAN_POINT('Ctrl Pts',(-33.3834046007805,-14.329723883874,-5.45835099719278)) ;
#61366=CARTESIAN_POINT('Ctrl Pts',(-33.5080604096064,-14.9406748977399,
-5.4784084571226)) ;
#61367=CARTESIAN_POINT('Ctrl Pts',(-33.5178586766213,-14.9886972685975,
-5.47998508973445)) ;
#61368=CARTESIAN_POINT('Ctrl Pts',(-33.5276414406682,-15.0366437072149,
-5.48155929099228)) ;
#61369=CARTESIAN_POINT('Ctrl Pts',(-33.5228460026744,-15.0366437072149,
-5.51081016871838)) ;
#61370=CARTESIAN_POINT('Ctrl Pts',(-33.513072690402,-14.9886972684499,-5.5091783139983)) ;
#61371=CARTESIAN_POINT('Ctrl Pts',(-33.5032839103576,-14.9406748974443,
-5.50754381323711)) ;
#61372=CARTESIAN_POINT('Ctrl Pts',(-33.3787490601101,-14.3297238832788,
-5.48674853823682)) ;
#61373=CARTESIAN_POINT('Ctrl Pts',(-33.2619584101797,-13.756757930604,-5.4672375645064)) ;
#61374=CARTESIAN_POINT('Ctrl Pts',(-33.0256329225343,-12.5973445377235,
-5.42773327067727)) ;
#61375=CARTESIAN_POINT('Ctrl Pts',(-32.9060980788614,-12.0108970975206,
-5.40773998692343)) ;
#61376=CARTESIAN_POINT('Ctrl Pts',(-32.6656595786491,-10.8312615209558,
-5.36749229367)) ;
#61377=CARTESIAN_POINT('Ctrl Pts',(-32.5447559096276,-10.2380733845424,
-5.34723796024904)) ;
#61378=CARTESIAN_POINT('Ctrl Pts',(-32.3634057724657,-9.34829125312033,
-5.31682382019003)) ;
#61379=CARTESIAN_POINT('Ctrl Pts',(-32.3029566282788,-9.05169722536708,
-5.30668029490438)) ;
#61380=CARTESIAN_POINT('Ctrl Pts',(-32.1822322424287,-8.45935179820167,
-5.28640885299969)) ;
#61381=CARTESIAN_POINT('Ctrl Pts',(-32.1219569993225,-8.16360039878257,
-5.27628094517738)) ;
#61382=CARTESIAN_POINT('Ctrl Pts',(-32.0017526279443,-7.57378282505162,
-5.25606661638952)) ;
#61383=CARTESIAN_POINT('Ctrl Pts',(-31.9418234965939,-7.27971665074306,
-5.24598021420588)) ;
#61384=CARTESIAN_POINT('Ctrl Pts',(-31.8224837416044,-6.6941121249061,-5.22587367463099)) ;
#61385=CARTESIAN_POINT('Ctrl Pts',(-31.7630731117453,-6.40257377334411,
-5.21585357513672)) ;
#61386=CARTESIAN_POINT('Ctrl Pts',(-31.6744755765251,-5.96779406257672,
-5.20089028140719)) ;
#61387=CARTESIAN_POINT('Ctrl Pts',(-31.645029469701,-5.82328879625627,-5.19591364065643)) ;
#61388=CARTESIAN_POINT('Ctrl Pts',(-31.5863317052322,-5.53522619562883,
-5.18598515289222)) ;
#61389=CARTESIAN_POINT('Ctrl Pts',(-31.5570800473982,-5.39166886132052,
-5.18103330703587)) ;
#61390=CARTESIAN_POINT('Ctrl Pts',(-31.4987928735203,-5.10560744918979,
-5.17115663068443)) ;
#61391=CARTESIAN_POINT('Ctrl Pts',(-31.469757356425,-4.9631033713697,-5.16623180660667)) ;
#61392=CARTESIAN_POINT('Ctrl Pts',(-31.411924236773,-4.67925379721435,-5.15641090728921)) ;
#61393=CARTESIAN_POINT('Ctrl Pts',(-31.3831266320664,-4.53790830086409,
-5.15151484514484)) ;
#61394=CARTESIAN_POINT('Ctrl Pts',(-31.3257912374526,-4.25648121551928,
-5.14175242649281)) ;
#61395=CARTESIAN_POINT('Ctrl Pts',(-31.2972534434363,-4.11639962743284,
-5.13688609621007)) ;
#61396=CARTESIAN_POINT('Ctrl Pts',(-31.2404597892109,-3.8376056863405,-5.12718276615013)) ;
#61397=CARTESIAN_POINT('Ctrl Pts',(-31.2122039193593,-3.69889333325525,
-5.12234582508958)) ;
#61398=CARTESIAN_POINT('Ctrl Pts',(-31.1700484631251,-3.49193072685828,
-5.11511024706567)) ;
#61399=CARTESIAN_POINT('Ctrl Pts',(-31.1560347069013,-3.42312751209455,
-5.11270166650645)) ;
#61400=CARTESIAN_POINT('Ctrl Pts',(-31.1280862111298,-3.28590289060839,
-5.10789024371521)) ;
#61401=CARTESIAN_POINT('Ctrl Pts',(-31.1141514712529,-3.21748148388252,
-5.10548740349358)) ;
#61402=CARTESIAN_POINT('Ctrl Pts',(-31.0863639876091,-3.08103364596632,
-5.10068610769772)) ;
#61403=CARTESIAN_POINT('Ctrl Pts',(-31.0725112412887,-3.01300721478954,
-5.09828766771808)) ;
#61404=CARTESIAN_POINT('Ctrl Pts',(-31.0448908710698,-2.87736249699739,
-5.09349292476487)) ;
#61405=CARTESIAN_POINT('Ctrl Pts',(-31.0311232408531,-2.80974421030951,
-5.09109666023862)) ;
#61406=CARTESIAN_POINT('Ctrl Pts',(-31.0048650142947,-2.68076678970341,
-5.08650996408753)) ;
#61407=CARTESIAN_POINT('Ctrl Pts',(-30.9917045601157,-2.61611857778466,
-5.08420404087192)) ;
#61408=CARTESIAN_POINT('Ctrl Pts',(-30.9714968930084,-2.51683757422274,
-5.08064454582576)) ;
#61409=CARTESIAN_POINT('Ctrl Pts',(-30.9646831776891,-2.48335912551026,
-5.07944125061466)) ;
#61410=CARTESIAN_POINT('Ctrl Pts',(-30.9509787645156,-2.41601749173412,
-5.07701277354403)) ;
#61411=CARTESIAN_POINT('Ctrl Pts',(-30.9440880637705,-2.38215430662499,
-5.07578760926055)) ;
#61412=CARTESIAN_POINT('Ctrl Pts',(-30.9303084831399,-2.31442802752013,
-5.07332629032738)) ;
#61413=CARTESIAN_POINT('Ctrl Pts',(-30.9234195988981,-2.2805649471878,-5.07209017970508)) ;
#61414=CARTESIAN_POINT('Ctrl Pts',(-30.9131469500024,-2.23005902105978,
-5.07023467362553)) ;
#61415=CARTESIAN_POINT('Ctrl Pts',(-30.9097328495601,-2.21327182815133,
-5.06961593037097)) ;
#61416=CARTESIAN_POINT('Ctrl Pts',(-30.9029348207521,-2.17984177586973,
-5.06837877291122)) ;
#61417=CARTESIAN_POINT('Ctrl Pts',(-30.8995508920192,-2.16319891648864,
-5.06776036093859)) ;
#61418=CARTESIAN_POINT('Ctrl Pts',(-30.8928232181419,-2.13010563471574,
-5.06652424551718)) ;
#61419=CARTESIAN_POINT('Ctrl Pts',(-30.8894794709209,-2.11365521616266,
-5.06590655963874)) ;
#61420=CARTESIAN_POINT('Ctrl Pts',(-30.882842304577,-2.08099492318782,-5.06467146933891)) ;
#61421=CARTESIAN_POINT('Ctrl Pts',(-30.8795488776322,-2.06478504856123,
-5.06405411236837)) ;
#61422=CARTESIAN_POINT('Ctrl Pts',(-30.8746543040369,-2.04068672479713,
-5.06312667196831)) ;
#61423=CARTESIAN_POINT('Ctrl Pts',(-30.8730303782615,-2.03269003243661,
-5.06281726597446)) ;
#61424=CARTESIAN_POINT('Ctrl Pts',(-30.8697990878884,-2.01677482597858,
-5.06219729959632)) ;
#61425=CARTESIAN_POINT('Ctrl Pts',(-30.8681917231571,-2.00885631187657,
-5.06188674002439)) ;
#61426=CARTESIAN_POINT('Ctrl Pts',(-30.8649950083338,-1.99310347870114,
-5.06126328654053)) ;
#61427=CARTESIAN_POINT('Ctrl Pts',(-30.8634056536514,-1.98526915980233,
-5.06095042085202)) ;
#61428=CARTESIAN_POINT('Ctrl Pts',(-30.8610363578164,-1.9735853449993,-5.06047766845265)) ;
#61429=CARTESIAN_POINT('Ctrl Pts',(-30.8602490504964,-1.96970201742585,
-5.06031949705393)) ;
#61430=CARTESIAN_POINT('Ctrl Pts',(-30.8586795935814,-1.96195867127126,
-5.06000146825683)) ;
#61431=CARTESIAN_POINT('Ctrl Pts',(-30.8578974436936,-1.95809865267673,
-5.05984161262806)) ;
#61432=CARTESIAN_POINT('Ctrl Pts',(-30.8563375858908,-1.95039770434896,
-5.05951919050395)) ;
#61433=CARTESIAN_POINT('Ctrl Pts',(-30.8555184294407,-1.94635216031222,
-5.05934807610711)) ;
#61434=CARTESIAN_POINT('Ctrl Pts',(-30.853842156775,-1.93806865717107,-5.05899160207087)) ;
#61435=CARTESIAN_POINT('Ctrl Pts',(-30.8529850286401,-1.93383069738739,
-5.0588063142689)) ;
#61436=CARTESIAN_POINT('Ctrl Pts',(-30.8517007137438,-1.92747402059848,
-5.05852031717912)) ;
#61437=CARTESIAN_POINT('Ctrl Pts',(-30.8512728437056,-1.92535518541571,
-5.05842362473753)) ;
#61438=CARTESIAN_POINT('Ctrl Pts',(-30.8504226359227,-1.92114170712674,
-5.05822739713357)) ;
#61439=CARTESIAN_POINT('Ctrl Pts',(-30.8500002923028,-1.9190470635643,-5.05812789722599)) ;
#61440=CARTESIAN_POINT('Ctrl Pts',(-30.8493748470567,-1.91594131035434,
-5.05797567853019)) ;
#61441=CARTESIAN_POINT('Ctrl Pts',(-30.8491677129878,-1.9149120984522,-5.05792443286985)) ;
#61442=CARTESIAN_POINT('Ctrl Pts',(-30.8487568346472,-1.91286876134158,
-5.05782053632988)) ;
#61443=CARTESIAN_POINT('Ctrl Pts',(-30.8485530899563,-1.91185463609014,
-5.05776788795337)) ;
#61444=CARTESIAN_POINT('Ctrl Pts',(-30.848149756389,-1.90984448796971,-5.05766036570063)) ;
#61445=CARTESIAN_POINT('Ctrl Pts',(-30.8479501615709,-1.90884846692931,
-5.05760553040331)) ;
#61446=CARTESIAN_POINT('Ctrl Pts',(-30.8476546035702,-1.90737028791818,
-5.05752013963832)) ;
#61447=CARTESIAN_POINT('Ctrl Pts',(-30.8475567249699,-1.90688020417638,
-5.05749114338188)) ;
#61448=CARTESIAN_POINT('Ctrl Pts',(-30.8473624264111,-1.90590570765277,
-5.05743149758875)) ;
#61449=CARTESIAN_POINT('Ctrl Pts',(-30.847266002424,-1.90542129422109,-5.05740087179522)) ;
#61450=CARTESIAN_POINT('Ctrl Pts',(-30.8471212998049,-1.90469230606236,
-5.05735231470238)) ;
#61451=CARTESIAN_POINT('Ctrl Pts',(-30.8470697753425,-1.90443237036805,
-5.0573345601076)) ;
#61452=CARTESIAN_POINT('Ctrl Pts',(-30.8469645620923,-1.90390032261935,
-5.05729669872756)) ;
#61453=CARTESIAN_POINT('Ctrl Pts',(-30.8469108724233,-1.90362821037409,
-5.05727659707329)) ;
#61454=CARTESIAN_POINT('Ctrl Pts',(-30.84680399421,-1.9030842986835,-5.05723373660809)) ;
#61455=CARTESIAN_POINT('Ctrl Pts',(-30.8467507980804,-1.90281253803109,
-5.05721107361941)) ;
#61456=CARTESIAN_POINT('Ctrl Pts',(-30.8465314744222,-1.90163369641421,
-5.05704304528566)) ;
#61457=CARTESIAN_POINT('Ctrl Pts',(-30.8465224173482,-1.90158501559319,
-5.0570361064763)) ;
#61458=CARTESIAN_POINT('Ctrl Pts',(-30.8465133602742,-1.90153633477217,
-5.05702916766694)) ;
#61459=CARTESIAN_POINT('',(-28.127216244771,-15.0366437072153,-19.0528197166343)) ;
#61460=CARTESIAN_POINT('',(-28.1105818993065,-15.0366437072153,-19.0773535407052)) ;
#61461=CARTESIAN_POINT('Origin',(1.13057562514854,-21.6462763158694,0.766549294070828)) ;
#61462=CARTESIAN_POINT('',(-25.8721458584193,-1.90153624169001,-17.541750139775)) ;
#61463=CARTESIAN_POINT('Ctrl Pts',(-25.8721458739748,-1.90153633180959,
-17.5417501500193)) ;
#61464=CARTESIAN_POINT('Ctrl Pts',(-25.8721577813986,-1.90158489219061,
-17.5417504704143)) ;
#61465=CARTESIAN_POINT('Ctrl Pts',(-25.8723630148979,-1.90242186726325,
-17.5417559926659)) ;
#61466=CARTESIAN_POINT('Ctrl Pts',(-25.8724455119795,-1.90282329663281,
-17.5417821463521)) ;
#61467=CARTESIAN_POINT('Ctrl Pts',(-25.8725001466519,-1.90309737347548,
-17.541802496001)) ;
#61468=CARTESIAN_POINT('Ctrl Pts',(-25.8726080673333,-1.90364591781988,
-17.5418453282902)) ;
#61469=CARTESIAN_POINT('Ctrl Pts',(-25.8726612926932,-1.90392034648623,
-17.5418678860799)) ;
#61470=CARTESIAN_POINT('Ctrl Pts',(-25.8727645374215,-1.90445692193452,
-17.5419132072959)) ;
#61471=CARTESIAN_POINT('Ctrl Pts',(-25.8728145539649,-1.90471906890233,
-17.5419359749571)) ;
#61472=CARTESIAN_POINT('Ctrl Pts',(-25.8729541313185,-1.90545432128996,
-17.542000873042)) ;
#61473=CARTESIAN_POINT('Ctrl Pts',(-25.8730459476192,-1.90594291892127,
-17.5420453819276)) ;
#61474=CARTESIAN_POINT('Ctrl Pts',(-25.8732295327942,-1.90692583257785,
-17.5421365754662)) ;
#61475=CARTESIAN_POINT('Ctrl Pts',(-25.8733212882221,-1.90742014925225,
-17.5421832801901)) ;
#61476=CARTESIAN_POINT('Ctrl Pts',(-25.8735968579746,-1.90891109528826,
-17.5423258913389)) ;
#61477=CARTESIAN_POINT('Ctrl Pts',(-25.8737809976514,-1.90991571864561,
-17.5424242617222)) ;
#61478=CARTESIAN_POINT('Ctrl Pts',(-25.8741508279643,-1.91194322733529,
-17.5426254400316)) ;
#61479=CARTESIAN_POINT('Ctrl Pts',(-25.8743364962106,-1.91296611084088,
-17.5427282803074)) ;
#61480=CARTESIAN_POINT('Ctrl Pts',(-25.8747093476694,-1.91502709440813,
-17.5429373300016)) ;
#61481=CARTESIAN_POINT('Ctrl Pts',(-25.8748965294705,-1.91606519451243,
-17.5430435415171)) ;
#61482=CARTESIAN_POINT('Ctrl Pts',(-25.8754599872941,-1.91919776827529,
-17.5433660847172)) ;
#61483=CARTESIAN_POINT('Ctrl Pts',(-25.8758381993206,-1.92131050012656,
-17.543586284653)) ;
#61484=CARTESIAN_POINT('Ctrl Pts',(-25.8765967515513,-1.92556036292269,
-17.5440325307497)) ;
#61485=CARTESIAN_POINT('Ctrl Pts',(-25.8769770716705,-1.92769749432427,
-17.5442586067019)) ;
#61486=CARTESIAN_POINT('Ctrl Pts',(-25.8781157276811,-1.93410905980131,
-17.5449402962874)) ;
#61487=CARTESIAN_POINT('Ctrl Pts',(-25.8788717873392,-1.93838361207301,
-17.54539931064)) ;
#61488=CARTESIAN_POINT('Ctrl Pts',(-25.8803463297327,-1.94673863693752,
-17.5463012906347)) ;
#61489=CARTESIAN_POINT('Ctrl Pts',(-25.8810647715554,-1.9508191102094,-17.5467443168686)) ;
#61490=CARTESIAN_POINT('Ctrl Pts',(-25.8824305365614,-1.95858685131004,
-17.5475904621936)) ;
#61491=CARTESIAN_POINT('Ctrl Pts',(-25.8831141360427,-1.96248050149649,
-17.5480160787776)) ;
#61492=CARTESIAN_POINT('Ctrl Pts',(-25.8844839505559,-1.97029131383045,
-17.5488721126596)) ;
#61493=CARTESIAN_POINT('Ctrl Pts',(-25.8851701645755,-1.97420847599133,
-17.5493025314554)) ;
#61494=CARTESIAN_POINT('Ctrl Pts',(-25.8872329915253,-1.98599408922772,
-17.5506001828878)) ;
#61495=CARTESIAN_POINT('Ctrl Pts',(-25.8886138158768,-1.99389666664285,
-17.5514737712874)) ;
#61496=CARTESIAN_POINT('Ctrl Pts',(-25.8913870826419,-2.00978675025176,
-17.5532350880485)) ;
#61497=CARTESIAN_POINT('Ctrl Pts',(-25.8927795088963,-2.01777425627098,
-17.5541228401787)) ;
#61498=CARTESIAN_POINT('Ctrl Pts',(-25.8955756988877,-2.033828127578,-17.5559106631073)) ;
#61499=CARTESIAN_POINT('Ctrl Pts',(-25.8969794621623,-2.04189449287027,
-17.5568107345884)) ;
#61500=CARTESIAN_POINT('Ctrl Pts',(-25.9012069175401,-2.06620277837357,
-17.5595273160892)) ;
#61501=CARTESIAN_POINT('Ctrl Pts',(-25.9040468319125,-2.08255388475044,
-17.5613601082406)) ;
#61502=CARTESIAN_POINT('Ctrl Pts',(-25.9097637854993,-2.1154987366553,-17.5650602902202)) ;
#61503=CARTESIAN_POINT('Ctrl Pts',(-25.9126407976318,-2.13209248238822,
-17.5669277200662)) ;
#61504=CARTESIAN_POINT('Ctrl Pts',(-25.9184247760832,-2.16547409486571,
-17.5706898863848)) ;
#61505=CARTESIAN_POINT('Ctrl Pts',(-25.9213317317786,-2.18226195777091,
-17.5725846371116)) ;
#61506=CARTESIAN_POINT('Ctrl Pts',(-25.9271679807421,-2.21598327435907,
-17.5763948074275)) ;
#61507=CARTESIAN_POINT('Ctrl Pts',(-25.9300972727453,-2.2329167280499,-17.5783102288843)) ;
#61508=CARTESIAN_POINT('Ctrl Pts',(-25.9389068846414,-2.28386269378459,
-17.5840780546505)) ;
#61509=CARTESIAN_POINT('Ctrl Pts',(-25.9448089812287,-2.3180208102006,-17.587951960061)) ;
#61510=CARTESIAN_POINT('Ctrl Pts',(-25.9566069656804,-2.38633716148301,
-17.5957089716833)) ;
#61511=CARTESIAN_POINT('Ctrl Pts',(-25.9625028263135,-2.4204953826845,-17.5995921130256)) ;
#61512=CARTESIAN_POINT('Ctrl Pts',(-25.9742230316132,-2.48842373596822,
-17.6073209586855)) ;
#61513=CARTESIAN_POINT('Ctrl Pts',(-25.980047366237,-2.52219386809602,-17.6111666778318)) ;
#61514=CARTESIAN_POINT('Ctrl Pts',(-25.9973144624853,-2.62233986386287,
-17.6225787316677)) ;
#61515=CARTESIAN_POINT('Ctrl Pts',(-26.0085513815388,-2.68755132653018,
-17.6300198666794)) ;
#61516=CARTESIAN_POINT('Ctrl Pts',(-26.030971806787,-2.81770994459726,-17.6448835826939)) ;
#61517=CARTESIAN_POINT('Ctrl Pts',(-26.042725988924,-2.88597501437035,-17.6526863133006)) ;
#61518=CARTESIAN_POINT('Ctrl Pts',(-26.06629829559,-3.02291720221945,-17.6683492047793)) ;
#61519=CARTESIAN_POINT('Ctrl Pts',(-26.0781163980912,-3.09159432036822,
-17.6762093981667)) ;
#61520=CARTESIAN_POINT('Ctrl Pts',(-26.101815783507,-3.22934731017729,-17.6919834431879)) ;
#61521=CARTESIAN_POINT('Ctrl Pts',(-26.1136970574824,-3.29842318182397,
-17.6998973080004)) ;
#61522=CARTESIAN_POINT('Ctrl Pts',(-26.1375215228422,-3.43696038516605,
-17.7157756633011)) ;
#61523=CARTESIAN_POINT('Ctrl Pts',(-26.1494647130785,-3.50642171686489,
-17.7237401554819)) ;
#61524=CARTESIAN_POINT('Ctrl Pts',(-26.1853848266085,-3.71536396318966,
-17.7477056693359)) ;
#61525=CARTESIAN_POINT('Ctrl Pts',(-26.2094523540066,-3.85540312838846,
-17.7637786376903)) ;
#61526=CARTESIAN_POINT('Ctrl Pts',(-26.2578145218226,-4.13686379057535,
-17.7960986563036)) ;
#61527=CARTESIAN_POINT('Ctrl Pts',(-26.2821091286492,-4.2782852876429,-17.812345756135)) ;
#61528=CARTESIAN_POINT('Ctrl Pts',(-26.3309094580666,-4.56240428036738,
-17.8449984743132)) ;
#61529=CARTESIAN_POINT('Ctrl Pts',(-26.3554151655153,-4.70510177511429,
-17.8614041146579)) ;
#61530=CARTESIAN_POINT('Ctrl Pts',(-26.4046209589496,-4.99166642802495,
-17.8943594411247)) ;
#61531=CARTESIAN_POINT('Ctrl Pts',(-26.4293210374488,-5.13553358620376,
-17.9109091382938)) ;
#61532=CARTESIAN_POINT('Ctrl Pts',(-26.4788983993845,-5.42433123356354,
-17.9441387502879)) ;
#61533=CARTESIAN_POINT('Ctrl Pts',(-26.5037756791504,-5.56926172274222,
-17.9608186705255)) ;
#61534=CARTESIAN_POINT('Ctrl Pts',(-26.553689992587,-5.86007970017216,-17.9942953098974)) ;
#61535=CARTESIAN_POINT('Ctrl Pts',(-26.5787270255941,-6.00596718842478,
-18.0110920300097)) ;
#61536=CARTESIAN_POINT('Ctrl Pts',(-26.6540513077496,-6.44490565440716,
-18.0616376606911)) ;
#61537=CARTESIAN_POINT('Ctrl Pts',(-26.7045517822166,-6.73923262866378,
-18.0955419776558)) ;
#61538=CARTESIAN_POINT('Ctrl Pts',(-26.8059788688949,-7.33043857872017,
-18.163661888986)) ;
#61539=CARTESIAN_POINT('Ctrl Pts',(-26.8569054594421,-7.62731755455363,
-18.1978775153162)) ;
#61540=CARTESIAN_POINT('Ctrl Pts',(-26.9590411910106,-8.22277685056084,
-18.2665185632472)) ;
#61541=CARTESIAN_POINT('Ctrl Pts',(-27.0102503212944,-8.52135717073135,
-18.3009440006836)) ;
#61542=CARTESIAN_POINT('Ctrl Pts',(-27.1128069266711,-9.11936849902312,
-18.369904101061)) ;
#61543=CARTESIAN_POINT('Ctrl Pts',(-27.1641543967405,-9.41879950715136,
-18.4044387714126)) ;
#61544=CARTESIAN_POINT('Ctrl Pts',(-27.318187428206,-10.3170925797302,-18.5080566328313)) ;
#61545=CARTESIAN_POINT('Ctrl Pts',(-27.4208636968131,-10.9159546769438,
-18.5771535417962)) ;
#61546=CARTESIAN_POINT('Ctrl Pts',(-27.6250318782106,-12.1068736983314,
-18.7145881249444)) ;
#61547=CARTESIAN_POINT('Ctrl Pts',(-27.7265237475234,-12.6989306225571,
-18.7829258632698)) ;
#61548=CARTESIAN_POINT('Ctrl Pts',(-27.9283695022688,-13.8764819136135,
-18.9188630557109)) ;
#61549=CARTESIAN_POINT('Ctrl Pts',(-28.0286949437812,-14.4618113900316,
-18.9864437399958)) ;
#61550=CARTESIAN_POINT('Ctrl Pts',(-28.1272162447821,-15.0366437072153,
-19.0528197166179)) ;
#61551=CARTESIAN_POINT('Ctrl Pts',(-28.1105818992957,-15.0366437072153,
-19.0773535407212)) ;
#61552=CARTESIAN_POINT('Ctrl Pts',(-28.1094142530856,-15.0298036696733,
-19.0765568221348)) ;
#61553=CARTESIAN_POINT('Ctrl Pts',(-28.1082463538653,-15.0229621458316,
-19.0757599293754)) ;
#61554=CARTESIAN_POINT('Ctrl Pts',(-28.0100756837395,-14.4478805124694,
-19.0087749993418)) ;
#61555=CARTESIAN_POINT('Ctrl Pts',(-27.9113355275183,-13.8694340292541,
-18.9413908806558)) ;
#61556=CARTESIAN_POINT('Ctrl Pts',(-27.711545210769,-12.6989306216801,-18.8050175518778)) ;
#61557=CARTESIAN_POINT('Ctrl Pts',(-27.6104950294686,-12.1068736973243,
-18.7360283724237)) ;
#61558=CARTESIAN_POINT('Ctrl Pts',(-27.4072510671399,-10.9159546756748,
-18.5972306680339)) ;
#61559=CARTESIAN_POINT('Ctrl Pts',(-27.305057242619,-10.3170925783295,-18.5274222072277)) ;
#61560=CARTESIAN_POINT('Ctrl Pts',(-27.1517851594422,-9.41879950555309,
-18.4226820309762)) ;
#61561=CARTESIAN_POINT('Ctrl Pts',(-27.1006975967947,-9.11936849735901,
-18.3877640258319)) ;
#61562=CARTESIAN_POINT('Ctrl Pts',(-26.9986751561934,-8.52135716893573,
-18.318016091304)) ;
#61563=CARTESIAN_POINT('Ctrl Pts',(-26.9477402732135,-8.22277684869958,
-18.2831861693315)) ;
#61564=CARTESIAN_POINT('Ctrl Pts',(-26.8461700063625,-7.62731755256142,
-18.2137111232893)) ;
#61565=CARTESIAN_POINT('Ctrl Pts',(-26.7955346117563,-7.33043857666269,
-18.1790660150537)) ;
#61566=CARTESIAN_POINT('Ctrl Pts',(-26.6947107651878,-6.73923262647628,
-18.1100563910771)) ;
#61567=CARTESIAN_POINT('Ctrl Pts',(-26.6445222915509,-6.44490565215494,
-18.0756919072913)) ;
#61568=CARTESIAN_POINT('Ctrl Pts',(-26.5696861864936,-6.00596718607602,
-18.0244262692216)) ;
#61569=CARTESIAN_POINT('Ctrl Pts',(-26.5448152633208,-5.86007969779135,
-18.007384555421)) ;
#61570=CARTESIAN_POINT('Ctrl Pts',(-26.4952410527753,-5.56926172029744,
-17.9734063017893)) ;
#61571=CARTESIAN_POINT('Ctrl Pts',(-26.4705377647392,-5.42433123108689,
-17.9564697629374)) ;
#61572=CARTESIAN_POINT('Ctrl Pts',(-26.4213177554839,-5.13553358366361,
-17.9227130951479)) ;
#61573=CARTESIAN_POINT('Ctrl Pts',(-26.3968010305949,-4.99166642545318,
-17.9058929716238)) ;
#61574=CARTESIAN_POINT('Ctrl Pts',(-26.3479733578889,-4.70510177247949,
-17.8723799587828)) ;
#61575=CARTESIAN_POINT('Ctrl Pts',(-26.3236624025812,-4.5624042777012,-17.8556870805081)) ;
#61576=CARTESIAN_POINT('Ctrl Pts',(-26.2752659236338,-4.27828528491426,
-17.8224387274259)) ;
#61577=CARTESIAN_POINT('Ctrl Pts',(-26.2511803851627,-4.13686378781561,
-17.805883274828)) ;
#61578=CARTESIAN_POINT('Ctrl Pts',(-26.2032551566929,-3.85540312556682,
-17.7729188188696)) ;
#61579=CARTESIAN_POINT('Ctrl Pts',(-26.1794154330761,-3.71536396033722,
-17.756509865063)) ;
#61580=CARTESIAN_POINT('Ctrl Pts',(-26.1438566240579,-3.5064217139665,-17.7320114669046)) ;
#61581=CARTESIAN_POINT('Ctrl Pts',(-26.1320371658283,-3.43696038225238,
-17.7238644836613)) ;
#61582=CARTESIAN_POINT('Ctrl Pts',(-26.1084681997397,-3.29842317887984,
-17.7076092951171)) ;
#61583=CARTESIAN_POINT('Ctrl Pts',(-26.096718690731,-3.22934730721796,-17.6995010915124)) ;
#61584=CARTESIAN_POINT('Ctrl Pts',(-26.0732929233236,-3.09159431737861,
-17.6833234901097)) ;
#61585=CARTESIAN_POINT('Ctrl Pts',(-26.0616166559903,-3.02291719921474,
-17.6752541054946)) ;
#61586=CARTESIAN_POINT('Ctrl Pts',(-26.0383411843299,-2.88597501133551,
-17.6591534151252)) ;
#61587=CARTESIAN_POINT('Ctrl Pts',(-26.0267419579497,-2.81770994154741,
-17.6511221418702)) ;
#61588=CARTESIAN_POINT('Ctrl Pts',(-26.0046352570039,-2.68755132374404,
-17.6357957172242)) ;
#61589=CARTESIAN_POINT('Ctrl Pts',(-25.9935634033709,-2.62233986136937,
-17.6281111290389)) ;
#61590=CARTESIAN_POINT('Ctrl Pts',(-25.9765706599549,-2.52219386605188,
-17.6162944352138)) ;
#61591=CARTESIAN_POINT('Ctrl Pts',(-25.9708422679448,-2.48842373407561,
-17.6123072113547)) ;
#61592=CARTESIAN_POINT('Ctrl Pts',(-25.9593242551378,-2.4204953810967,-17.6042801541909)) ;
#61593=CARTESIAN_POINT('Ctrl Pts',(-25.9535346242879,-2.38633716004853,
-17.6002403356964)) ;
#61594=CARTESIAN_POINT('Ctrl Pts',(-25.941961656926,-2.31802080907265,-17.5921514488089)) ;
#61595=CARTESIAN_POINT('Ctrl Pts',(-25.9361782978659,-2.2838626928099,-17.5881024187041)) ;
#61596=CARTESIAN_POINT('Ctrl Pts',(-25.9275593485474,-2.23291672730382,
-17.5820533867584)) ;
#61597=CARTESIAN_POINT('Ctrl Pts',(-25.9246957238749,-2.21598327368894,
-17.5800411132628)) ;
#61598=CARTESIAN_POINT('Ctrl Pts',(-25.9189959459532,-2.1822619572521,-17.5760296632747)) ;
#61599=CARTESIAN_POINT('Ctrl Pts',(-25.9161597914317,-2.16547409442222,
-17.5740304886564)) ;
#61600=CARTESIAN_POINT('Ctrl Pts',(-25.9105239554163,-2.13209248209452,
-17.5700498286465)) ;
#61601=CARTESIAN_POINT('Ctrl Pts',(-25.9077242646122,-2.11549873643605,
-17.5680683584003)) ;
#61602=CARTESIAN_POINT('Ctrl Pts',(-25.9021708190636,-2.08255388467903,
-17.5641270201609)) ;
#61603=CARTESIAN_POINT('Ctrl Pts',(-25.8994170371719,-2.06620277837558,
-17.5621671921317)) ;
#61604=CARTESIAN_POINT('Ctrl Pts',(-25.8953286536826,-2.04189449298133,
-17.5592454949812)) ;
#61605=CARTESIAN_POINT('Ctrl Pts',(-25.8939729218816,-2.03382812772519,
-17.5582745823897)) ;
#61606=CARTESIAN_POINT('Ctrl Pts',(-25.8912770994085,-2.01777425649022,
-17.556338728473)) ;
#61607=CARTESIAN_POINT('Ctrl Pts',(-25.8899370082718,-2.00978675050687,
-17.5553737878323)) ;
#61608=CARTESIAN_POINT('Ctrl Pts',(-25.8872742941722,-1.99389666696925,
-17.5534494181145)) ;
#61609=CARTESIAN_POINT('Ctrl Pts',(-25.8859516551153,-1.98599408958961,
-17.5524900128389)) ;
#61610=CARTESIAN_POINT('Ctrl Pts',(-25.8839826361903,-1.97420847640609,
-17.5510540049405)) ;
#61611=CARTESIAN_POINT('Ctrl Pts',(-25.8833287931713,-1.97029131426291,
-17.5505758424973)) ;
#61612=CARTESIAN_POINT('Ctrl Pts',(-25.8820265370122,-1.96248050196401,
-17.5496201675104)) ;
#61613=CARTESIAN_POINT('Ctrl Pts',(-25.8813781228567,-1.9585868517949,-17.5491426564597)) ;
#61614=CARTESIAN_POINT('Ctrl Pts',(-25.8800865517807,-1.95081911052775,
-17.5481870832136)) ;
#61615=CARTESIAN_POINT('Ctrl Pts',(-25.8794090679542,-1.94673863706264,
-17.5476836483835)) ;
#61616=CARTESIAN_POINT('Ctrl Pts',(-25.8780253650712,-1.93838361180268,
-17.5466476899886)) ;
#61617=CARTESIAN_POINT('Ctrl Pts',(-25.8773191048395,-1.93410905932831,
-17.5461152269026)) ;
#61618=CARTESIAN_POINT('Ctrl Pts',(-25.8762643710015,-1.92769749354789,
-17.5453097612609)) ;
#61619=CARTESIAN_POINT('Ctrl Pts',(-25.8759135807207,-1.92556036204565,
-17.5450401320186)) ;
#61620=CARTESIAN_POINT('Ctrl Pts',(-25.8752182593306,-1.9213104990485,-17.544500627335)) ;
#61621=CARTESIAN_POINT('Ctrl Pts',(-25.8748737080166,-1.91919776709772,
-17.5442307815258)) ;
#61622=CARTESIAN_POINT('Ctrl Pts',(-25.8743655156321,-1.91606519318668,
-17.5438267278466)) ;
#61623=CARTESIAN_POINT('Ctrl Pts',(-25.8741975644428,-1.91502709303237,
-17.5436921532823)) ;
#61624=CARTESIAN_POINT('Ctrl Pts',(-25.8738653555782,-1.91296610936764,
-17.5434231602105)) ;
#61625=CARTESIAN_POINT('Ctrl Pts',(-25.8737010964528,-1.91194322581388,
-17.543288743826)) ;
#61626=CARTESIAN_POINT('Ctrl Pts',(-25.8733773181643,-1.9099157170284,-17.5430196438268)) ;
#61627=CARTESIAN_POINT('Ctrl Pts',(-25.8732177772496,-1.90891109362396,
-17.5428849929664)) ;
#61628=CARTESIAN_POINT('Ctrl Pts',(-25.8729832959266,-1.90742014751768,
-17.542681780892)) ;
#61629=CARTESIAN_POINT('Ctrl Pts',(-25.8729059461416,-1.90692583082018,
-17.5426138294259)) ;
#61630=CARTESIAN_POINT('Ctrl Pts',(-25.8727532775796,-1.90594291711709,
-17.5424770372775)) ;
#61631=CARTESIAN_POINT('Ctrl Pts',(-25.8726779451098,-1.90545431946123,
-17.5424082165512)) ;
#61632=CARTESIAN_POINT('Ctrl Pts',(-25.8725659934106,-1.90471906717225,
-17.5423025737106)) ;
#61633=CARTESIAN_POINT('Ctrl Pts',(-25.8725263298085,-1.90445692033434,
-17.5422645366511)) ;
#61634=CARTESIAN_POINT('Ctrl Pts',(-25.8724460126798,-1.90392034514695,
-17.5421853998518)) ;
#61635=CARTESIAN_POINT('Ctrl Pts',(-25.8724053562799,-1.90364591661258,
-17.5421443042816)) ;
#61636=CARTESIAN_POINT('Ctrl Pts',(-25.8723256205637,-1.90309737253521,
-17.5420599023772)) ;
#61637=CARTESIAN_POINT('Ctrl Pts',(-25.8722864938872,-1.90282329582858,
-17.5420166801957)) ;
#61638=CARTESIAN_POINT('Ctrl Pts',(-25.872156512694,-1.90163369816862,-17.5417703145868)) ;
#61639=CARTESIAN_POINT('Ctrl Pts',(-25.8721511933344,-1.9015850149891,-17.5417602323031)) ;
#61640=CARTESIAN_POINT('Ctrl Pts',(-25.8721458739748,-1.90153633180959,
-17.5417501500193)) ;
#61641=CARTESIAN_POINT('',(-17.5274987345151,-15.0366437072153,-29.1021824086485)) ;
#61642=CARTESIAN_POINT('',(-17.5021003261057,-15.0366437072153,-29.1174641239516)) ;
#61643=CARTESIAN_POINT('Origin',(0.704216953074891,-21.6462763158693,1.17041768075435)) ;
#61644=CARTESIAN_POINT('',(-16.1153339290263,-1.90153624083151,-26.7838933247298)) ;
#61645=CARTESIAN_POINT('Ctrl Pts',(-16.1153339387476,-1.90153633009259,
-26.783893340409)) ;
#61646=CARTESIAN_POINT('Ctrl Pts',(-16.1153446126417,-1.90158489024226,
-26.7838986300072)) ;
#61647=CARTESIAN_POINT('Ctrl Pts',(-16.1155284746913,-1.90242135803618,
-26.7839897454288)) ;
#61648=CARTESIAN_POINT('Ctrl Pts',(-16.1155923341218,-1.90282255286718,
-26.7840480837299)) ;
#61649=CARTESIAN_POINT('Ctrl Pts',(-16.1156333539989,-1.90309646971259,
-26.7840894668884)) ;
#61650=CARTESIAN_POINT('Ctrl Pts',(-16.1157132749115,-1.90364469403042,
-26.7841736022824)) ;
#61651=CARTESIAN_POINT('Ctrl Pts',(-16.1157520893281,-1.90391896267546,
-26.7842163972704)) ;
#61652=CARTESIAN_POINT('Ctrl Pts',(-16.1158267233644,-1.90445522534681,
-26.7843008287304)) ;
#61653=CARTESIAN_POINT('Ctrl Pts',(-16.1158625386521,-1.90471721955859,
-26.7843424678536)) ;
#61654=CARTESIAN_POINT('Ctrl Pts',(-16.1159619132824,-1.90545203961471,
-26.7844599019948)) ;
#61655=CARTESIAN_POINT('Ctrl Pts',(-16.116026520158,-1.90594034860819,-26.7845388010006)) ;
#61656=CARTESIAN_POINT('Ctrl Pts',(-16.1161547774474,-1.90692268162604,
-26.7846985528625)) ;
#61657=CARTESIAN_POINT('Ctrl Pts',(-16.1162184071348,-1.90741670630277,
-26.7847794183467)) ;
#61658=CARTESIAN_POINT('Ctrl Pts',(-16.1164085234146,-1.90890677163164,
-26.7850244071299)) ;
#61659=CARTESIAN_POINT('Ctrl Pts',(-16.1165342707288,-1.90991080157223,
-26.7851909021158)) ;
#61660=CARTESIAN_POINT('Ctrl Pts',(-16.1167853089992,-1.91193711267859,
-26.7855285685486)) ;
#61661=CARTESIAN_POINT('Ctrl Pts',(-16.1169105661903,-1.9129593920142,-26.7856997598699)) ;
#61662=CARTESIAN_POINT('Ctrl Pts',(-16.1171610404156,-1.91501915827682,
-26.7860458344817)) ;
#61663=CARTESIAN_POINT('Ctrl Pts',(-16.1172862552069,-1.91605664524807,
-26.7862207191324)) ;
#61664=CARTESIAN_POINT('Ctrl Pts',(-16.1176619936659,-1.9191873688501,-26.7867497211197)) ;
#61665=CARTESIAN_POINT('Ctrl Pts',(-16.1179126495691,-1.92129885291666,
-26.7871081598582)) ;
#61666=CARTESIAN_POINT('Ctrl Pts',(-16.1184134373359,-1.92554620580213,
-26.7878312338195)) ;
#61667=CARTESIAN_POINT('Ctrl Pts',(-16.1186635385443,-1.92768207507662,
-26.7881958875967)) ;
#61668=CARTESIAN_POINT('Ctrl Pts',(-16.119410298339,-1.93408985417006,-26.7892920224878)) ;
#61669=CARTESIAN_POINT('Ctrl Pts',(-16.1199034641827,-1.938361882184,-26.7900256336217)) ;
#61670=CARTESIAN_POINT('Ctrl Pts',(-16.1208624448587,-1.94671197326914,
-26.7914625314618)) ;
#61671=CARTESIAN_POINT('Ctrl Pts',(-16.1213281971216,-1.95079003701957,
-26.7921658559786)) ;
#61672=CARTESIAN_POINT('Ctrl Pts',(-16.1222119368299,-1.95855317037308,
-26.7935064607666)) ;
#61673=CARTESIAN_POINT('Ctrl Pts',(-16.1226533878534,-1.96244450036797,
-26.7941793699059)) ;
#61674=CARTESIAN_POINT('Ctrl Pts',(-16.1235366471255,-1.97025065831423,
-26.7955306405496)) ;
#61675=CARTESIAN_POINT('Ctrl Pts',(-16.1239784538358,-1.97416548627894,
-26.7962090029826)) ;
#61676=CARTESIAN_POINT('Ctrl Pts',(-16.1253049854054,-1.98594407659837,
-26.7982516474305)) ;
#61677=CARTESIAN_POINT('Ctrl Pts',(-16.1261908623444,-1.99384194496366,
-26.799623462041)) ;
#61678=CARTESIAN_POINT('Ctrl Pts',(-16.1279672192149,-2.0097225598768,-26.8023847928812)) ;
#61679=CARTESIAN_POINT('Ctrl Pts',(-16.1288576745073,-2.01770530625007,
-26.8037743238935)) ;
#61680=CARTESIAN_POINT('Ctrl Pts',(-16.1306436982338,-2.03374961128295,
-26.8065693176019)) ;
#61681=CARTESIAN_POINT('Ctrl Pts',(-16.1315392659522,-2.04181116994711,
-26.8079747807291)) ;
#61682=CARTESIAN_POINT('Ctrl Pts',(-16.1342337624508,-2.06610497051377,
-26.8122127999703)) ;
#61683=CARTESIAN_POINT('Ctrl Pts',(-16.1360405716602,-2.08244633352993,
-26.8150669327094)) ;
#61684=CARTESIAN_POINT('Ctrl Pts',(-16.1396733430882,-2.11537155415295,
-26.8208221597007)) ;
#61685=CARTESIAN_POINT('Ctrl Pts',(-16.141499263935,-2.13195541196474,-26.8237232788947)) ;
#61686=CARTESIAN_POINT('Ctrl Pts',(-16.1451668147149,-2.16531713295146,
-26.829562856173)) ;
#61687=CARTESIAN_POINT('Ctrl Pts',(-16.1470084290269,-2.18209499228712,
-26.8325013227301)) ;
#61688=CARTESIAN_POINT('Ctrl Pts',(-16.1507032439754,-2.21579621499984,
-26.8384063776397)) ;
#61689=CARTESIAN_POINT('Ctrl Pts',(-16.1525564426753,-2.23271957838481,
-26.8413729671588)) ;
#61690=CARTESIAN_POINT('Ctrl Pts',(-16.1581267045493,-2.28363518646551,
-26.8503014147369)) ;
#61691=CARTESIAN_POINT('Ctrl Pts',(-16.1618544958079,-2.31777294879703,
-26.8562919142551)) ;
#61692=CARTESIAN_POINT('Ctrl Pts',(-16.1693005829469,-2.38604859190971,
-26.8682786550392)) ;
#61693=CARTESIAN_POINT('Ctrl Pts',(-16.17301883939,-2.42018645902605,-26.8742749167378)) ;
#61694=CARTESIAN_POINT('Ctrl Pts',(-16.180406192469,-2.48807433543556,-26.8862034740195)) ;
#61695=CARTESIAN_POINT('Ctrl Pts',(-16.1840752737782,-2.52182434477429,
-26.8921357788352)) ;
#61696=CARTESIAN_POINT('Ctrl Pts',(-16.1949482476549,-2.62191066606263,
-26.9097328149812)) ;
#61697=CARTESIAN_POINT('Ctrl Pts',(-16.2020179694901,-2.68708327092924,
-26.9211976081664)) ;
#61698=CARTESIAN_POINT('Ctrl Pts',(-16.2161163182727,-2.81716036567911,
-26.9440872558194)) ;
#61699=CARTESIAN_POINT('Ctrl Pts',(-16.2235030433896,-2.88538078045149,
-26.9560963934278)) ;
#61700=CARTESIAN_POINT('Ctrl Pts',(-16.2383103870237,-3.02223338876827,
-26.9801935895711)) ;
#61701=CARTESIAN_POINT('Ctrl Pts',(-16.2457309719123,-3.09086558238541,
-26.9922816683572)) ;
#61702=CARTESIAN_POINT('Ctrl Pts',(-16.2606069272933,-3.22852846229517,
-27.0165330056586)) ;
#61703=CARTESIAN_POINT('Ctrl Pts',(-16.2680622841446,-3.29755914857421,
-27.0286962723779)) ;
#61704=CARTESIAN_POINT('Ctrl Pts',(-16.2830079107993,-3.43600572903974,
-27.0530947048677)) ;
#61705=CARTESIAN_POINT('Ctrl Pts',(-16.2904981788528,-3.50542162322967,
-27.0653298716909)) ;
#61706=CARTESIAN_POINT('Ctrl Pts',(-16.3130208735933,-3.71422719185778,
-27.1021387030916)) ;
#61707=CARTESIAN_POINT('Ctrl Pts',(-16.3281052845003,-3.85417475169892,
-27.1268156420992)) ;
#61708=CARTESIAN_POINT('Ctrl Pts',(-16.3584070420383,-4.13545129894057,
-27.176422711748)) ;
#61709=CARTESIAN_POINT('Ctrl Pts',(-16.3736243373896,-4.27678028642054,
-27.2013528732623)) ;
#61710=CARTESIAN_POINT('Ctrl Pts',(-16.4041838861447,-4.56071342529593,
-27.2514455589791)) ;
#61711=CARTESIAN_POINT('Ctrl Pts',(-16.4195261165778,-4.70331757578152,
-27.2766080967833)) ;
#61712=CARTESIAN_POINT('Ctrl Pts',(-16.4503264287325,-4.98969477505206,
-27.3271453850117)) ;
#61713=CARTESIAN_POINT('Ctrl Pts',(-16.4657844990219,-5.13346782385208,
-27.3525201423181)) ;
#61714=CARTESIAN_POINT('Ctrl Pts',(-16.4968067176875,-5.42207655689294,
-27.4034621211301)) ;
#61715=CARTESIAN_POINT('Ctrl Pts',(-16.5123708604603,-5.56691224113146,
-27.4290293460064)) ;
#61716=CARTESIAN_POINT('Ctrl Pts',(-16.5435950273506,-5.85753998267579,
-27.4803367664907)) ;
#61717=CARTESIAN_POINT('Ctrl Pts',(-16.5592550504579,-6.00333203998292,
-27.506076962706)) ;
#61718=CARTESIAN_POINT('Ctrl Pts',(-16.6063632327434,-6.44198337845498,
-27.5835280164297)) ;
#61719=CARTESIAN_POINT('Ctrl Pts',(-16.6379395699958,-6.73611782147322,
-27.6354692987059)) ;
#61720=CARTESIAN_POINT('Ctrl Pts',(-16.7013481215964,-7.32693703970546,
-27.7398130030787)) ;
#61721=CARTESIAN_POINT('Ctrl Pts',(-16.733180302874,-7.62362181495312,-27.7922154450812)) ;
#61722=CARTESIAN_POINT('Ctrl Pts',(-16.7970128957945,-8.21869159689002,
-27.897329174614)) ;
#61723=CARTESIAN_POINT('Ctrl Pts',(-16.8290132910475,-8.51707660357599,
-27.950040472005)) ;
#61724=CARTESIAN_POINT('Ctrl Pts',(-16.8930937212076,-9.11469674844867,
-28.055620186193)) ;
#61725=CARTESIAN_POINT('Ctrl Pts',(-16.9251737484442,-9.41393188664231,
-28.1084886076062)) ;
#61726=CARTESIAN_POINT('Ctrl Pts',(-17.0213995067575,-10.3116373494152,
-28.2671025015741)) ;
#61727=CARTESIAN_POINT('Ctrl Pts',(-17.0855310480243,-10.9101077067561,
-28.372856519752)) ;
#61728=CARTESIAN_POINT('Ctrl Pts',(-17.2130385160227,-12.1002476999845,
-28.5831789780471)) ;
#61729=CARTESIAN_POINT('Ctrl Pts',(-17.2764143763867,-12.6919173359235,
-28.6877474581075)) ;
#61730=CARTESIAN_POINT('Ctrl Pts',(-17.4027580047438,-13.8716326279716,
-28.8962559180836)) ;
#61731=CARTESIAN_POINT('Ctrl Pts',(-17.4657003340837,-14.4594442697278,
-29.0001547637196)) ;
#61732=CARTESIAN_POINT('Ctrl Pts',(-17.5274987345487,-15.0366437072153,
-29.1021824086283)) ;
#61733=CARTESIAN_POINT('Ctrl Pts',(-17.502100326071,-15.0366437072153,-29.1174641239725)) ;
#61734=CARTESIAN_POINT('Ctrl Pts',(-17.5010738690874,-15.026962147902,-29.1157466982005)) ;
#61735=CARTESIAN_POINT('Ctrl Pts',(-17.5000470977353,-15.0172776029008,
-29.1140287414815)) ;
#61736=CARTESIAN_POINT('Ctrl Pts',(-17.4388139593873,-14.4397231677713,
-29.0115753703577)) ;
#61737=CARTESIAN_POINT('Ctrl Pts',(-17.3775338698389,-13.8616550697814,
-28.9090263622473)) ;
#61738=CARTESIAN_POINT('Ctrl Pts',(-17.2535520883261,-12.6919173358369,
-28.7015032404052)) ;
#61739=CARTESIAN_POINT('Ctrl Pts',(-17.1908503646563,-12.100247699885,-28.5965291457508)) ;
#61740=CARTESIAN_POINT('Ctrl Pts',(-17.064753513795,-10.9101077066308,-28.3853579472788)) ;
#61741=CARTESIAN_POINT('Ctrl Pts',(-17.0013583202276,-10.3116373492769,
-28.2791608833869)) ;
#61742=CARTESIAN_POINT('Ctrl Pts',(-16.9062939918949,-9.41393188648451,
-28.1198481801811)) ;
#61743=CARTESIAN_POINT('Ctrl Pts',(-16.8746106603403,-9.11469674828439,
-28.0667410748938)) ;
#61744=CARTESIAN_POINT('Ctrl Pts',(-16.8113455255754,-8.51707660339873,
-27.9606708137394)) ;
#61745=CARTESIAN_POINT('Ctrl Pts',(-16.7797637146953,-8.21869159670628,
-27.907707662486)) ;
#61746=CARTESIAN_POINT('Ctrl Pts',(-16.7167941939307,-7.62362181475645,
-27.8020746396636)) ;
#61747=CARTESIAN_POINT('Ctrl Pts',(-16.6854064676566,-7.32693703950234,
-27.7494047779567)) ;
#61748=CARTESIAN_POINT('Ctrl Pts',(-16.622918648862,-6.73611782125726,-27.6445070870324)) ;
#61749=CARTESIAN_POINT('Ctrl Pts',(-16.5918185232645,-6.44198337823263,
-27.5922792777087)) ;
#61750=CARTESIAN_POINT('Ctrl Pts',(-16.545455454652,-6.00333203975106,-27.5143799039606)) ;
#61751=CARTESIAN_POINT('Ctrl Pts',(-16.5300489682726,-5.85753998244076,
-27.4884871597568)) ;
#61752=CARTESIAN_POINT('Ctrl Pts',(-16.4993439076299,-5.56691224089011,
-27.4368674034048)) ;
#61753=CARTESIAN_POINT('Ctrl Pts',(-16.4840453323553,-5.42207655664842,
-27.4111403918658)) ;
#61754=CARTESIAN_POINT('Ctrl Pts',(-16.4535685495787,-5.13346782360132,
-27.3598702351666)) ;
#61755=CARTESIAN_POINT('Ctrl Pts',(-16.4383903364743,-4.98969477479818,
-27.3343270933781)) ;
#61756=CARTESIAN_POINT('Ctrl Pts',(-16.4081671598198,-4.70331757552142,
-27.2834425542393)) ;
#61757=CARTESIAN_POINT('Ctrl Pts',(-16.3931221848344,-4.56071342503274,
-27.2581011637657)) ;
#61758=CARTESIAN_POINT('Ctrl Pts',(-16.3631790442451,-4.27678028615114,
-27.2076375975596)) ;
#61759=CARTESIAN_POINT('Ctrl Pts',(-16.3482808558656,-4.13545129866813,
-27.18251543575)) ;
#61760=CARTESIAN_POINT('Ctrl Pts',(-16.3186460113394,-3.85417475142036,
-27.1325070978543)) ;
#61761=CARTESIAN_POINT('Ctrl Pts',(-16.3039093038976,-3.71422719157617,
-27.1076209526123)) ;
#61762=CARTESIAN_POINT('Ctrl Pts',(-16.2819380783363,-3.50542162294355,
-27.0704803132146)) ;
#61763=CARTESIAN_POINT('Ctrl Pts',(-16.2746366658577,-3.4360057287521,-27.0581315157619)) ;
#61764=CARTESIAN_POINT('Ctrl Pts',(-16.2600810145637,-3.29755914828356,
-27.0334984428819)) ;
#61765=CARTESIAN_POINT('Ctrl Pts',(-16.2528267739962,-3.22852846200301,
-27.0212141685092)) ;
#61766=CARTESIAN_POINT('Ctrl Pts',(-16.23836844846,-3.09086558209025,-26.9967115516668)) ;
#61767=CARTESIAN_POINT('Ctrl Pts',(-16.2311643498569,-3.02223338847166,
-26.9844932174041)) ;
#61768=CARTESIAN_POINT('Ctrl Pts',(-16.2168100715694,-2.8853807801519,-26.9601234208857)) ;
#61769=CARTESIAN_POINT('Ctrl Pts',(-16.2096598582408,-2.81716036537802,
-26.9479719788555)) ;
#61770=CARTESIAN_POINT('Ctrl Pts',(-16.1960403644138,-2.68708327060819,
-26.9247942137304)) ;
#61771=CARTESIAN_POINT('Ctrl Pts',(-16.1892225989311,-2.62191066572221,
-26.9131778234331)) ;
#61772=CARTESIAN_POINT('Ctrl Pts',(-16.1787683982861,-2.52182434440409,
-26.8953288197866)) ;
#61773=CARTESIAN_POINT('Ctrl Pts',(-16.1752457641844,-2.48807433505531,
-26.8893084006073)) ;
#61774=CARTESIAN_POINT('Ctrl Pts',(-16.1681670386877,-2.42018645862559,
-26.8771941482657)) ;
#61775=CARTESIAN_POINT('Ctrl Pts',(-16.1646109319503,-2.3860485914991,-26.8711003243238)) ;
#61776=CARTESIAN_POINT('Ctrl Pts',(-16.1575083121581,-2.31777294836608,
-26.8589069260889)) ;
#61777=CARTESIAN_POINT('Ctrl Pts',(-16.1539617625691,-2.2836351860244,-26.8528073770738)) ;
#61778=CARTESIAN_POINT('Ctrl Pts',(-16.148682529273,-2.23271957792855,-26.8437038234067)) ;
#61779=CARTESIAN_POINT('Ctrl Pts',(-16.1469295656237,-2.21579621453857,
-26.8406769244575)) ;
#61780=CARTESIAN_POINT('Ctrl Pts',(-16.1434430609953,-2.18209499181582,
-26.8346465333844)) ;
#61781=CARTESIAN_POINT('Ctrl Pts',(-16.1417095180719,-2.16531713247511,
-26.831643042429)) ;
#61782=CARTESIAN_POINT('Ctrl Pts',(-16.1382680929536,-2.13195541147845,
-26.8256674098519)) ;
#61783=CARTESIAN_POINT('Ctrl Pts',(-16.1365601959534,-2.11537155366181,
-26.8226952780645)) ;
#61784=CARTESIAN_POINT('Ctrl Pts',(-16.1331770043878,-2.082446333029,-26.81678988385)) ;
#61785=CARTESIAN_POINT('Ctrl Pts',(-16.1315016684144,-2.06610497000793,
-26.8138566462883)) ;
#61786=CARTESIAN_POINT('Ctrl Pts',(-16.1290194522718,-2.04181116943406,
-26.809490902193)) ;
#61787=CARTESIAN_POINT('Ctrl Pts',(-16.1281972001465,-2.03374961076746,
-26.8080413265364)) ;
#61788=CARTESIAN_POINT('Ctrl Pts',(-16.1265643781298,-2.01770530572983,
-26.8051541544166)) ;
#61789=CARTESIAN_POINT('Ctrl Pts',(-16.1257538075399,-2.00972255935432,
-26.803716558373)) ;
#61790=CARTESIAN_POINT('Ctrl Pts',(-16.1241461990354,-1.99384194443646,
-26.8008536950086)) ;
#61791=CARTESIAN_POINT('Ctrl Pts',(-16.1233491365322,-1.98594407606877,
-26.7994284425245)) ;
#61792=CARTESIAN_POINT('Ctrl Pts',(-16.1221657941448,-1.97416548574584,
-26.7972996440034)) ;
#61793=CARTESIAN_POINT('Ctrl Pts',(-16.1217733987392,-1.97025065777981,
-26.7965915517745)) ;
#61794=CARTESIAN_POINT('Ctrl Pts',(-16.1209932609488,-1.96244449983124,
-26.7951782349933)) ;
#61795=CARTESIAN_POINT('Ctrl Pts',(-16.1206055170121,-1.95855316983527,
-26.7944730113718)) ;
#61796=CARTESIAN_POINT('Ctrl Pts',(-16.1198350276745,-1.95079003648729,
-26.7930642660979)) ;
#61797=CARTESIAN_POINT('Ctrl Pts',(-16.1194317942876,-1.94671197274391,
-26.7923233252232)) ;
#61798=CARTESIAN_POINT('Ctrl Pts',(-16.1186114723841,-1.93836188167317,
-26.7908029991712)) ;
#61799=CARTESIAN_POINT('Ctrl Pts',(-16.1181943211566,-1.93408985366662,
-26.790023651562)) ;
#61800=CARTESIAN_POINT('Ctrl Pts',(-16.1175756613713,-1.92768207458426,
-26.7888504414553)) ;
#61801=CARTESIAN_POINT('Ctrl Pts',(-16.1173706349253,-1.92554620531401,
-26.7884586670944)) ;
#61802=CARTESIAN_POINT('Ctrl Pts',(-16.1169663635938,-1.9212988524359,-26.7876775211226)) ;
#61803=CARTESIAN_POINT('Ctrl Pts',(-16.116767087912,-1.91918736837177,-26.7872881679312)) ;
#61804=CARTESIAN_POINT('Ctrl Pts',(-16.1164757073549,-1.91605664477523,
-26.7867084094797)) ;
#61805=CARTESIAN_POINT('Ctrl Pts',(-16.1163798463686,-1.91501915780667,
-26.7865158632312)) ;
#61806=CARTESIAN_POINT('Ctrl Pts',(-16.1161914095241,-1.91295939154775,
-26.7861324619666)) ;
#61807=CARTESIAN_POINT('Ctrl Pts',(-16.1160988314997,-1.91193711221481,
-26.7859416082438)) ;
#61808=CARTESIAN_POINT('Ctrl Pts',(-16.1159180875877,-1.909910801112,-26.7855616470997)) ;
#61809=CARTESIAN_POINT('Ctrl Pts',(-16.1158298882342,-1.90890677116962,
-26.785372560255)) ;
#61810=CARTESIAN_POINT('Ctrl Pts',(-16.1157024897718,-1.90741670584362,
-26.7850898354139)) ;
#61811=CARTESIAN_POINT('Ctrl Pts',(-16.1156608488991,-1.90692268117004,
-26.7849957396996)) ;
#61812=CARTESIAN_POINT('Ctrl Pts',(-16.1155797830039,-1.90594034815389,
-26.7848075937183)) ;
#61813=CARTESIAN_POINT('Ctrl Pts',(-16.1155403371682,-1.90545203916062,
-26.7847135558172)) ;
#61814=CARTESIAN_POINT('Ctrl Pts',(-16.1154831306131,-1.90471721919977,
-26.7845707500099)) ;
#61815=CARTESIAN_POINT('Ctrl Pts',(-16.1154631181873,-1.90445522508891,
-26.7845196026446)) ;
#61816=CARTESIAN_POINT('Ctrl Pts',(-16.1154234811987,-1.90391896261954,
-26.7844141142082)) ;
#61817=CARTESIAN_POINT('Ctrl Pts',(-16.1154038522064,-1.90364469407305,
-26.7843597757572)) ;
#61818=CARTESIAN_POINT('Ctrl Pts',(-16.1153669532182,-1.9030964699622,-26.7842497549801)) ;
#61819=CARTESIAN_POINT('Ctrl Pts',(-16.1153496049406,-1.9028225532317,-26.7841941291205)) ;
#61820=CARTESIAN_POINT('Ctrl Pts',(-16.1153351246656,-1.90163369613048,
-26.783916109868)) ;
#61821=CARTESIAN_POINT('Ctrl Pts',(-16.1153345317066,-1.90158501311153,
-26.7839047251385)) ;
#61822=CARTESIAN_POINT('Ctrl Pts',(-16.1153339387476,-1.90153633009259,
-26.783893340409)) ;
#61823=CARTESIAN_POINT('',(-3.68783779512238,-15.0366437072151,-33.7720311090634)) ;
#61824=CARTESIAN_POINT('',(-3.65837019749682,-15.0366437072151,-33.7752359034359)) ;
#61825=CARTESIAN_POINT('Origin',(0.147684368304155,-21.6462763158694,1.35793534153108)) ;
#61826=CARTESIAN_POINT('',(-3.37961604955383,-1.90153624239224,-31.0750563097204)) ;
#61827=CARTESIAN_POINT('Ctrl Pts',(-3.37961605183184,-1.90153633321405,
-31.0750563283525)) ;
#61828=CARTESIAN_POINT('Ctrl Pts',(-3.37962354756522,-1.9015848895933,-31.0750656069308)) ;
#61829=CARTESIAN_POINT('Ctrl Pts',(-3.37975139855505,-1.90241309156327,
-31.0752238670187)) ;
#61830=CARTESIAN_POINT('Ctrl Pts',(-3.37978465679827,-1.90281047596646,
-31.0753028573227)) ;
#61831=CARTESIAN_POINT('Ctrl Pts',(-3.37980438554198,-1.90308179329851,
-31.0753571125156)) ;
#61832=CARTESIAN_POINT('Ctrl Pts',(-3.3798413566566,-1.90362481830771,-31.0754659744547)) ;
#61833=CARTESIAN_POINT('Ctrl Pts',(-3.37985850315228,-1.90389648719278,
-31.075520583564)) ;
#61834=CARTESIAN_POINT('Ctrl Pts',(-3.37989057697063,-1.90442766834731,
-31.075627516043)) ;
#61835=CARTESIAN_POINT('Ctrl Pts',(-3.37990549913902,-1.90468718080719,
-31.0756798400127)) ;
#61836=CARTESIAN_POINT('Ctrl Pts',(-3.37994610388543,-1.90541496999656,
-31.0758267151235)) ;
#61837=CARTESIAN_POINT('Ctrl Pts',(-3.37997143437742,-1.90589858257301,
-31.0759244925368)) ;
#61838=CARTESIAN_POINT('Ctrl Pts',(-3.38002041476513,-1.9068714680578,-31.0761214067959)) ;
#61839=CARTESIAN_POINT('Ctrl Pts',(-3.38004404067381,-1.90736074161815,
-31.0762205463861)) ;
#61840=CARTESIAN_POINT('Ctrl Pts',(-3.38011322017132,-1.9088364770218,-31.0765197951444)) ;
#61841=CARTESIAN_POINT('Ctrl Pts',(-3.38015711441919,-1.90983085157814,
-31.0767217296534)) ;
#61842=CARTESIAN_POINT('Ctrl Pts',(-3.38024253489509,-1.91183767688721,
-31.0771296138472)) ;
#61843=CARTESIAN_POINT('Ctrl Pts',(-3.38028402232049,-1.91285012581093,
-31.0773355673717)) ;
#61844=CARTESIAN_POINT('Ctrl Pts',(-3.38036541672939,-1.91489008539149,
-31.0777507773029)) ;
#61845=CARTESIAN_POINT('Ctrl Pts',(-3.38040532114009,-1.91591759609217,
-31.0779600339982)) ;
#61846=CARTESIAN_POINT('Ctrl Pts',(-3.38052330051655,-1.91901821585069,
-31.078591752673)) ;
#61847=CARTESIAN_POINT('Ctrl Pts',(-3.38059968734525,-1.92110939731572,
-31.0790181550988)) ;
#61848=CARTESIAN_POINT('Ctrl Pts',(-3.38074939599317,-1.92531591161341,
-31.0798763138211)) ;
#61849=CARTESIAN_POINT('Ctrl Pts',(-3.38082268235303,-1.92743124490193,
-31.0803080740687)) ;
#61850=CARTESIAN_POINT('Ctrl Pts',(-3.38103843251987,-1.93377741600093,
-31.0816038372784)) ;
#61851=CARTESIAN_POINT('Ctrl Pts',(-3.3811768517012,-1.9380083719859,-31.0824683046859)) ;
#61852=CARTESIAN_POINT('Ctrl Pts',(-3.38144167913154,-1.94627818587562,
-31.0841586128613)) ;
#61853=CARTESIAN_POINT('Ctrl Pts',(-3.38156801504025,-1.95031704445984,
-31.084984461638)) ;
#61854=CARTESIAN_POINT('Ctrl Pts',(-3.38180517498327,-1.95800520912717,
-31.0865568669311)) ;
#61855=CARTESIAN_POINT('Ctrl Pts',(-3.3819222814648,-1.96185879110988,-31.0873452045946)) ;
#61856=CARTESIAN_POINT('Ctrl Pts',(-3.38215453649361,-1.96958922519025,
-31.0889269301978)) ;
#61857=CARTESIAN_POINT('Ctrl Pts',(-3.38226968324156,-1.97346607730139,
-31.0897203183359)) ;
#61858=CARTESIAN_POINT('Ctrl Pts',(-3.38261296631772,-1.98513040932147,
-31.0921077385685)) ;
#61859=CARTESIAN_POINT('Ctrl Pts',(-3.38283899223427,-1.99295166450382,
-31.0937090213102)) ;
#61860=CARTESIAN_POINT('Ctrl Pts',(-3.38328779588863,-2.00867822988399,
-31.0969294132178)) ;
#61861=CARTESIAN_POINT('Ctrl Pts',(-3.38351054522694,-2.01658353990714,
-31.0985485254358)) ;
#61862=CARTESIAN_POINT('Ctrl Pts',(-3.38395399654487,-2.03247220787073,
-31.1018031969574)) ;
#61863=CARTESIAN_POINT('Ctrl Pts',(-3.38417469770074,-2.04045556581573,
-31.1034387563511)) ;
#61864=CARTESIAN_POINT('Ctrl Pts',(-3.38483479024306,-2.06451370586719,
-31.1083681177909)) ;
#61865=CARTESIAN_POINT('Ctrl Pts',(-3.38527227156083,-2.08069655073069,
-31.1116845914063)) ;
#61866=CARTESIAN_POINT('Ctrl Pts',(-3.3861448836398,-2.11330238314372,-31.1183677145852)) ;
#61867=CARTESIAN_POINT('Ctrl Pts',(-3.38657996664064,-2.1297253708981,-31.1217343693854)) ;
#61868=CARTESIAN_POINT('Ctrl Pts',(-3.38744869755865,-2.16276347024479,
-31.1285077733221)) ;
#61869=CARTESIAN_POINT('Ctrl Pts',(-3.38788232782417,-2.17937857799855,
-31.1319145235804)) ;
#61870=CARTESIAN_POINT('Ctrl Pts',(-3.38874828635231,-2.21275288640396,
-31.1387581193989)) ;
#61871=CARTESIAN_POINT('Ctrl Pts',(-3.38918061235563,-2.22951208706357,
-31.1421949652061)) ;
#61872=CARTESIAN_POINT('Ctrl Pts',(-3.39047522403265,-2.27993379582334,
-31.1525357165685)) ;
#61873=CARTESIAN_POINT('Ctrl Pts',(-3.39133521532922,-2.31374041041457,
-31.159469828178)) ;
#61874=CARTESIAN_POINT('Ctrl Pts',(-3.39304422259448,-2.38135375803524,
-31.1733392696568)) ;
#61875=CARTESIAN_POINT('Ctrl Pts',(-3.39389319440513,-2.41516047740165,
-31.1802746014881)) ;
#61876=CARTESIAN_POINT('Ctrl Pts',(-3.39557350849034,-2.4823898213473,-31.1940673377372)) ;
#61877=CARTESIAN_POINT('Ctrl Pts',(-3.3964048330676,-2.51581244597206,-31.2009247440892)) ;
#61878=CARTESIAN_POINT('Ctrl Pts',(-3.39886118328916,-2.6149279022379,-31.2212614930262)) ;
#61879=CARTESIAN_POINT('Ctrl Pts',(-3.40044870012823,-2.67946831591532,
-31.2345053529434)) ;
#61880=CARTESIAN_POINT('Ctrl Pts',(-3.40360177143294,-2.80821979403678,
-31.2609269969686)) ;
#61881=CARTESIAN_POINT('Ctrl Pts',(-3.40524625729531,-2.87571441798806,
-31.2747787755693)) ;
#61882=CARTESIAN_POINT('Ctrl Pts',(-3.40853282785513,-3.01111106389717,
-31.302567282874)) ;
#61883=CARTESIAN_POINT('Ctrl Pts',(-3.41017487387755,-3.07901308592743,
-31.3165040157991)) ;
#61884=CARTESIAN_POINT('Ctrl Pts',(-3.41345892963355,-3.21521138321956,
-31.3444594420512)) ;
#61885=CARTESIAN_POINT('Ctrl Pts',(-3.41510092368816,-3.28350765846785,
-31.3584781370803)) ;
#61886=CARTESIAN_POINT('Ctrl Pts',(-3.41838635957247,-3.42048131874613,
-31.3865945939094)) ;
#61887=CARTESIAN_POINT('Ctrl Pts',(-3.42002979939743,-3.48915870377952,
-31.4006923559271)) ;
#61888=CARTESIAN_POINT('Ctrl Pts',(-3.42496374500222,-3.69574280972321,
-31.4430999858881)) ;
#61889=CARTESIAN_POINT('Ctrl Pts',(-3.42825798486587,-3.8342014808235,-31.4715241858609)) ;
#61890=CARTESIAN_POINT('Ctrl Pts',(-3.43486056686863,-4.11248555386922,
-31.5286551649569)) ;
#61891=CARTESIAN_POINT('Ctrl Pts',(-3.43816884992288,-4.25231095589393,
-31.5573619505224)) ;
#61892=CARTESIAN_POINT('Ctrl Pts',(-3.44480102513381,-4.53322335765963,
-31.6150360820933)) ;
#61893=CARTESIAN_POINT('Ctrl Pts',(-3.44812489090923,-4.67431035649286,
-31.6440034307791)) ;
#61894=CARTESIAN_POINT('Ctrl Pts',(-3.45478843702903,-4.95764081678049,
-31.702176811003)) ;
#61895=CARTESIAN_POINT('Ctrl Pts',(-3.458128104198,-5.09988427824991,-31.7313828439771)) ;
#61896=CARTESIAN_POINT('Ctrl Pts',(-3.46482268996876,-5.38542253146676,
-31.7900117993526)) ;
#61897=CARTESIAN_POINT('Ctrl Pts',(-3.46817760210812,-5.52871732321187,
-31.8194347224561)) ;
#61898=CARTESIAN_POINT('Ctrl Pts',(-3.47490162628081,-5.81625310512141,
-31.8784757178839)) ;
#61899=CARTESIAN_POINT('Ctrl Pts',(-3.47827073715131,-5.96049409528712,
-31.9080937903341)) ;
#61900=CARTESIAN_POINT('Ctrl Pts',(-3.48839731486342,-6.3944786661344,-31.9972081732342)) ;
#61901=CARTESIAN_POINT('Ctrl Pts',(-3.49517410239131,-6.68548384247647,
-32.0569646400372)) ;
#61902=CARTESIAN_POINT('Ctrl Pts',(-3.50876576219942,-7.27001739496297,
-32.1769979486495)) ;
#61903=CARTESIAN_POINT('Ctrl Pts',(-3.51558059633832,-7.56354577114107,
-32.2372747946138)) ;
#61904=CARTESIAN_POINT('Ctrl Pts',(-3.52923293369486,-8.15228466666954,
-32.3581757011858)) ;
#61905=CARTESIAN_POINT('Ctrl Pts',(-3.53607041801162,-8.44749518601661,
-32.4187997638484)) ;
#61906=CARTESIAN_POINT('Ctrl Pts',(-3.54975155112279,-9.03875731206524,
-32.5402220620514)) ;
#61907=CARTESIAN_POINT('Ctrl Pts',(-3.55659519106777,-9.33480891877373,
-32.6010202985551)) ;
#61908=CARTESIAN_POINT('Ctrl Pts',(-3.57710956616611,-10.2229637870553,
-32.7834168174283)) ;
#61909=CARTESIAN_POINT('Ctrl Pts',(-3.59076391219278,-10.8150670813697,
-32.9050168890259)) ;
#61910=CARTESIAN_POINT('Ctrl Pts',(-3.61788642535806,-11.9925453014778,
-33.1468386026216)) ;
#61911=CARTESIAN_POINT('Ctrl Pts',(-3.6313545159283,-12.5779202273231,-33.2670602529568)) ;
#61912=CARTESIAN_POINT('Ctrl Pts',(-3.65795827616522,-13.7352132469821,
-33.5047423312816)) ;
#61913=CARTESIAN_POINT('Ctrl Pts',(-3.67109390926027,-14.307131340793,-33.622202763248)) ;
#61914=CARTESIAN_POINT('Ctrl Pts',(-3.68527448816673,-14.9249537986604,
-33.7490920441471)) ;
#61915=CARTESIAN_POINT('Ctrl Pts',(-3.68655737279856,-14.9808505489368,
-33.7605722099422)) ;
#61916=CARTESIAN_POINT('Ctrl Pts',(-3.68783779586363,-15.0366437072147,
-33.7720311089823)) ;
#61917=CARTESIAN_POINT('Ctrl Pts',(-3.65837019675635,-15.0366437072147,
-33.775235903516)) ;
#61918=CARTESIAN_POINT('Ctrl Pts',(-3.65715735966888,-14.9808505488501,
-33.7637696540398)) ;
#61919=CARTESIAN_POINT('Ctrl Pts',(-3.65594235487438,-14.9249537984867,
-33.7522821058494)) ;
#61920=CARTESIAN_POINT('Ctrl Pts',(-3.64251395514954,-14.3071313404433,
-33.625311020498)) ;
#61921=CARTESIAN_POINT('Ctrl Pts',(-3.6300919636707,-13.7352132465421,-33.5077729753098)) ;
#61922=CARTESIAN_POINT('Ctrl Pts',(-3.60497912176554,-12.5779202267003,
-33.2699287498069)) ;
#61923=CARTESIAN_POINT('Ctrl Pts',(-3.59228823476317,-11.9925453007625,
-33.1496225734707)) ;
#61924=CARTESIAN_POINT('Ctrl Pts',(-3.56679211841482,-10.8150670804683,
-32.9076239785231)) ;
#61925=CARTESIAN_POINT('Ctrl Pts',(-3.55398681249849,-10.2229637860605,
-32.7859315682295)) ;
#61926=CARTESIAN_POINT('Ctrl Pts',(-3.53481171294889,-9.33480891763853,
-32.6033893943336)) ;
#61927=CARTESIAN_POINT('Ctrl Pts',(-3.52842552872936,-9.03875731088329,
-32.5425414065118)) ;
#61928=CARTESIAN_POINT('Ctrl Pts',(-3.5156845996532,-8.44749518474126,-32.4210168549385)) ;
#61929=CARTESIAN_POINT('Ctrl Pts',(-3.5093298459469,-8.15228466534754,-32.3603402921485)) ;
#61930=CARTESIAN_POINT('Ctrl Pts',(-3.49667287813304,-7.56354576972608,
-32.2393311325957)) ;
#61931=CARTESIAN_POINT('Ctrl Pts',(-3.49037064512079,-7.27001739350161,
-32.1789985378896)) ;
#61932=CARTESIAN_POINT('Ctrl Pts',(-3.47784092628131,-6.68548384092276,
-32.0588497362179)) ;
#61933=CARTESIAN_POINT('Ctrl Pts',(-3.47161340231218,-6.39447866453474,
-31.9990335333934)) ;
#61934=CARTESIAN_POINT('Ctrl Pts',(-3.46234626814233,-5.96049409361887,
-31.9098256803611)) ;
#61935=CARTESIAN_POINT('Ctrl Pts',(-3.45926960099435,-5.81625310343037,
-31.8801758027346)) ;
#61936=CARTESIAN_POINT('Ctrl Pts',(-3.45314435244001,-5.52871732147542,
-31.8210696865245)) ;
#61937=CARTESIAN_POINT('Ctrl Pts',(-3.45009576986793,-5.38542252970768,
-31.7916134480681)) ;
#61938=CARTESIAN_POINT('Ctrl Pts',(-3.44403034759674,-5.09988427644571,
-31.7329160670292)) ;
#61939=CARTESIAN_POINT('Ctrl Pts',(-3.44101350143869,-4.95764081495384,
-31.7036749251497)) ;
#61940=CARTESIAN_POINT('Ctrl Pts',(-3.435015700397,-4.67431035462144,-31.645429140776)) ;
#61941=CARTESIAN_POINT('Ctrl Pts',(-3.43203473233864,-4.53322335576592,
-31.6164244997114)) ;
#61942=CARTESIAN_POINT('Ctrl Pts',(-3.42611361752552,-4.25231095395583,
-31.5586730356528)) ;
#61943=CARTESIAN_POINT('Ctrl Pts',(-3.42317344443355,-4.11248555190906,
-31.5299262157117)) ;
#61944=CARTESIAN_POINT('Ctrl Pts',(-3.41734019001161,-3.83420147881938,
-31.4727115671899)) ;
#61945=CARTESIAN_POINT('Ctrl Pts',(-3.41444704959424,-3.69574280769723,
-31.444243745019)) ;
#61946=CARTESIAN_POINT('Ctrl Pts',(-3.41014925541112,-3.48915870172089,
-31.4017669294148)) ;
#61947=CARTESIAN_POINT('Ctrl Pts',(-3.40872367042118,-3.42048131667665,
-31.3876454742537)) ;
#61948=CARTESIAN_POINT('Ctrl Pts',(-3.40588808753802,-3.28350765637674,
-31.3594800929579)) ;
#61949=CARTESIAN_POINT('Ctrl Pts',(-3.40447808762632,-3.21521138111763,
-31.345436167043)) ;
#61950=CARTESIAN_POINT('Ctrl Pts',(-3.40167577369564,-3.07901308380399,
-31.3174283482056)) ;
#61951=CARTESIAN_POINT('Ctrl Pts',(-3.40028344398735,-3.011111061763,-31.3034644569924)) ;
#61952=CARTESIAN_POINT('Ctrl Pts',(-3.39751946870557,-2.8757144158325,-31.2756191140218)) ;
#61953=CARTESIAN_POINT('Ctrl Pts',(-3.39614778446167,-2.80821979187057,
-31.2617376664548)) ;
#61954=CARTESIAN_POINT('Ctrl Pts',(-3.39354726626481,-2.67946831377512,
-31.2352559286632)) ;
#61955=CARTESIAN_POINT('Ctrl Pts',(-3.39225062944861,-2.61492790013619,
-31.2219804336451)) ;
#61956=CARTESIAN_POINT('Ctrl Pts',(-3.39027775169719,-2.51581244392945,
-31.2015911039206)) ;
#61957=CARTESIAN_POINT('Ctrl Pts',(-3.38961550070132,-2.48238981932461,
-31.1947153097126)) ;
#61958=CARTESIAN_POINT('Ctrl Pts',(-3.38829149939526,-2.41516047541903,
-31.1808838221218)) ;
#61959=CARTESIAN_POINT('Ctrl Pts',(-3.38762973137363,-2.38135375607278,
-31.1739281306557)) ;
#61960=CARTESIAN_POINT('Ctrl Pts',(-3.38631726306021,-2.31374040849244,
-31.1600155629754)) ;
#61961=CARTESIAN_POINT('Ctrl Pts',(-3.38566651923091,-2.27993379392141,
-31.1530586943365)) ;
#61962=CARTESIAN_POINT('Ctrl Pts',(-3.38470790773418,-2.22951208519171,
-31.1426814007587)) ;
#61963=CARTESIAN_POINT('Ctrl Pts',(-3.38439130594481,-2.21275288454212,
-31.1392319691868)) ;
#61964=CARTESIAN_POINT('Ctrl Pts',(-3.38376584803932,-2.17937857615662,
-31.1323622173535)) ;
#61965=CARTESIAN_POINT('Ctrl Pts',(-3.38345698967685,-2.16276346841279,
-31.1289418973351)) ;
#61966=CARTESIAN_POINT('Ctrl Pts',(-3.38284932852388,-2.12972536908577,
-31.1221401003545)) ;
#61967=CARTESIAN_POINT('Ctrl Pts',(-3.38255050824406,-2.11330238134113,
-31.1187586260923)) ;
#61968=CARTESIAN_POINT('Ctrl Pts',(-3.38196604520614,-2.08069654894753,
-31.1120441648207)) ;
#61969=CARTESIAN_POINT('Ctrl Pts',(-3.38168035465867,-2.06451370409367,
-31.1087111829663)) ;
#61970=CARTESIAN_POINT('Ctrl Pts',(-3.38126534760574,-2.04045556405656,
-31.1037551668761)) ;
#61971=CARTESIAN_POINT('Ctrl Pts',(-3.38112929197016,-2.03247220611634,
-31.1021104017283)) ;
#61972=CARTESIAN_POINT('Ctrl Pts',(-3.38086271747385,-2.01658353816223,
-31.098836493695)) ;
#61973=CARTESIAN_POINT('Ctrl Pts',(-3.38073219780292,-2.00867822814386,
-31.0972073508972)) ;
#61974=CARTESIAN_POINT('Ctrl Pts',(-3.38047821961298,-1.99295166277309,
-31.0939657704455)) ;
#61975=CARTESIAN_POINT('Ctrl Pts',(-3.38035473270136,-1.98513040759533,
-31.0923533359159)) ;
#61976=CARTESIAN_POINT('Ctrl Pts',(-3.38017676523144,-1.97346607558221,
-31.0899479365291)) ;
#61977=CARTESIAN_POINT('Ctrl Pts',(-3.38011866495113,-1.96958922347363,
-31.0891483442143)) ;
#61978=CARTESIAN_POINT('Ctrl Pts',(-3.38000546573751,-1.96185878939789,
-31.0875536705118)) ;
#61979=CARTESIAN_POINT('Ctrl Pts',(-3.37995036499538,-1.95800520741715,
-31.0867585893183)) ;
#61980=CARTESIAN_POINT('Ctrl Pts',(-3.37984395961066,-1.9503170426067,-31.0851719635802)) ;
#61981=CARTESIAN_POINT('Ctrl Pts',(-3.37978980878068,-1.94627818386982,
-31.0843382641714)) ;
#61982=CARTESIAN_POINT('Ctrl Pts',(-3.37968507839923,-1.93800836966755,
-31.0826305443277)) ;
#61983=CARTESIAN_POINT('Ctrl Pts',(-3.37963442649015,-1.93377741352282,
-31.0817565316209)) ;
#61984=CARTESIAN_POINT('Ctrl Pts',(-3.37956658174528,-1.9274312421839,-31.0804446826773)) ;
#61985=CARTESIAN_POINT('Ctrl Pts',(-3.37954533904407,-1.9253159088158,-31.0800072623241)) ;
#61986=CARTESIAN_POINT('Ctrl Pts',(-3.37950706883426,-1.9211093943593,-31.0791369839084)) ;
#61987=CARTESIAN_POINT('Ctrl Pts',(-3.37949000588967,-1.91901821281563,
-31.078704129605)) ;
#61988=CARTESIAN_POINT('Ctrl Pts',(-3.37946942613243,-1.91591759293996,
-31.0780618180589)) ;
#61989=CARTESIAN_POINT('Ctrl Pts',(-3.3794634135807,-1.91489008220023,-31.0778488753936)) ;
#61990=CARTESIAN_POINT('Ctrl Pts',(-3.37945364718064,-1.91285012254287,
-31.0774258754311)) ;
#61991=CARTESIAN_POINT('Ctrl Pts',(-3.37944989077964,-1.91183767358176,
-31.0772158184026)) ;
#61992=CARTESIAN_POINT('Ctrl Pts',(-3.37944563114251,-1.90983084819726,
-31.07679910742)) ;
#61993=CARTESIAN_POINT('Ctrl Pts',(-3.37944508902013,-1.90883647359888,
-31.0765924580745)) ;
#61994=CARTESIAN_POINT('Ctrl Pts',(-3.3794483215085,-1.9073607381399,-31.0762853340266)) ;
#61995=CARTESIAN_POINT('Ctrl Pts',(-3.37945008313227,-1.90687146456539,
-31.0761834333729)) ;
#61996=CARTESIAN_POINT('Ctrl Pts',(-3.37945558765507,-1.9058985790443,-31.0759805935151)) ;
#61997=CARTESIAN_POINT('Ctrl Pts',(-3.37945930654473,-1.90541496644589,
-31.0758796567867)) ;
#61998=CARTESIAN_POINT('Ctrl Pts',(-3.37946738816771,-1.9046871772366,-31.07572748671)) ;
#61999=CARTESIAN_POINT('Ctrl Pts',(-3.3794707135693,-1.90442766478295,-31.0756731781987)) ;
#62000=CARTESIAN_POINT('Ctrl Pts',(-3.37947905021081,-1.90389648362564,
-31.0755618508168)) ;
#62001=CARTESIAN_POINT('Ctrl Pts',(-3.37948405653174,-1.90362481474057,
-31.0755048324435)) ;
#62002=CARTESIAN_POINT('Ctrl Pts',(-3.37949676121262,-1.90308178972856,
-31.0753905679354)) ;
#62003=CARTESIAN_POINT('Ctrl Pts',(-3.37950436512425,-1.90281047237712,
-31.0753333401331)) ;
#62004=CARTESIAN_POINT('Ctrl Pts',(-3.37960751752133,-1.9016336939429,-31.0750774956391)) ;
#62005=CARTESIAN_POINT('Ctrl Pts',(-3.37961178467659,-1.90158501357847,
-31.0750669119958)) ;
#62006=CARTESIAN_POINT('Ctrl Pts',(-3.37961605183184,-1.90153633321405,
-31.0750563283525)) ;
#62007=CARTESIAN_POINT('',(-10.8616065908228,-15.0366437072153,-32.189683675067)) ;
#62008=CARTESIAN_POINT('',(-10.8335168660197,-15.0366437072153,-32.1991482053229)) ;
#62009=CARTESIAN_POINT('Origin',(0.436147547989918,-21.6462763158694,1.2944397941978)) ;
#62010=CARTESIAN_POINT('',(-9.98082103895569,-1.90153624240863,-29.6220212119843)) ;
#62011=CARTESIAN_POINT('Ctrl Pts',(-9.98082104518866,-1.90153633324684,
-29.6220212296937)) ;
#62012=CARTESIAN_POINT('Ctrl Pts',(-9.98083034329157,-1.90158489192866,
-29.6220286862145)) ;
#62013=CARTESIAN_POINT('Ctrl Pts',(-9.98098989087541,-1.90241811784944,
-29.6221566338067)) ;
#62014=CARTESIAN_POINT('Ctrl Pts',(-9.98103957355631,-1.90281781834771,
-29.6222270582998)) ;
#62015=CARTESIAN_POINT('Ctrl Pts',(-9.98107064674613,-1.9030907157319,-29.6222761005186)) ;
#62016=CARTESIAN_POINT('Ctrl Pts',(-9.9811304334122,-1.90363690104155,-29.6223750652033)) ;
#62017=CARTESIAN_POINT('Ctrl Pts',(-9.98115905341219,-1.90391015014683,
-29.6224250106994)) ;
#62018=CARTESIAN_POINT('Ctrl Pts',(-9.98121362464133,-1.90444442000563,
-29.622523134212)) ;
#62019=CARTESIAN_POINT('Ctrl Pts',(-9.98123957102262,-1.9047054409468,-29.6225713139028)) ;
#62020=CARTESIAN_POINT('Ctrl Pts',(-9.98131115116327,-1.90543750368787,
-29.6227068400549)) ;
#62021=CARTESIAN_POINT('Ctrl Pts',(-9.98135713841576,-1.90592397086527,
-29.622797431294)) ;
#62022=CARTESIAN_POINT('Ctrl Pts',(-9.98144776083572,-1.90690259879769,
-29.6229803109675)) ;
#62023=CARTESIAN_POINT('Ctrl Pts',(-9.98149237318018,-1.9073947602025,-29.6230726072336)) ;
#62024=CARTESIAN_POINT('Ctrl Pts',(-9.98162494237531,-1.90887920569416,
-29.6233516593688)) ;
#62025=CARTESIAN_POINT('Ctrl Pts',(-9.98171166876545,-1.90987944903977,
-29.6235405655408)) ;
#62026=CARTESIAN_POINT('Ctrl Pts',(-9.98188367149003,-1.91189811830544,
-29.6239228316236)) ;
#62027=CARTESIAN_POINT('Ctrl Pts',(-9.98196891051252,-1.91291654239933,
-29.6241162037079)) ;
#62028=CARTESIAN_POINT('Ctrl Pts',(-9.98213855534324,-1.91496854097824,
-29.6245065325352)) ;
#62029=CARTESIAN_POINT('Ctrl Pts',(-9.98222295877125,-1.91600211550575,
-29.6247034900893)) ;
#62030=CARTESIAN_POINT('Ctrl Pts',(-9.98247532544751,-1.91912103313602,
-29.6252986146565)) ;
#62031=CARTESIAN_POINT('Ctrl Pts',(-9.9826424881391,-1.92122455503296,-29.6257010157422)) ;
#62032=CARTESIAN_POINT('Ctrl Pts',(-9.98297497037919,-1.92545589204945,
-29.6265117366763)) ;
#62033=CARTESIAN_POINT('Ctrl Pts',(-9.98314025600325,-1.92758370762544,
-29.6269200680547)) ;
#62034=CARTESIAN_POINT('Ctrl Pts',(-9.98363219204553,-1.93396732561015,
-29.628146420618)) ;
#62035=CARTESIAN_POINT('Ctrl Pts',(-9.98395498088245,-1.93822324620528,
-29.6289657686947)) ;
#62036=CARTESIAN_POINT('Ctrl Pts',(-9.98458042813596,-1.94654185458999,
-29.6305691084042)) ;
#62037=CARTESIAN_POINT('Ctrl Pts',(-9.98488301743629,-1.95060454305893,
-29.6313531234732)) ;
#62038=CARTESIAN_POINT('Ctrl Pts',(-9.98545584580792,-1.9583382748244,-29.6328466457974)) ;
#62039=CARTESIAN_POINT('Ctrl Pts',(-9.98574128637346,-1.96221480024253,
-29.6335958415099)) ;
#62040=CARTESIAN_POINT('Ctrl Pts',(-9.98631134298126,-1.9699912596771,-29.6350996155706)) ;
#62041=CARTESIAN_POINT('Ctrl Pts',(-9.98659595732225,-1.97389119370685,
-29.6358541944948)) ;
#62042=CARTESIAN_POINT('Ctrl Pts',(-9.98744925814862,-1.9856249725075,-29.6381255234136)) ;
#62043=CARTESIAN_POINT('Ctrl Pts',(-9.98801744723912,-1.99349279357557,
-29.6396498503683)) ;
#62044=CARTESIAN_POINT('Ctrl Pts',(-9.9891545036605,-2.00931299105223,-29.6427167151263)) ;
#62045=CARTESIAN_POINT('Ctrl Pts',(-9.98972334382125,-2.01726536728617,
-29.6442592620461)) ;
#62046=CARTESIAN_POINT('Ctrl Pts',(-9.99086258006404,-2.03324863225896,
-29.6473609532205)) ;
#62047=CARTESIAN_POINT('Ctrl Pts',(-9.99143297537365,-2.04127952100227,
-29.6489200977357)) ;
#62048=CARTESIAN_POINT('Ctrl Pts',(-9.99314710341874,-2.06548089672393,
-29.6536202467501)) ;
#62049=CARTESIAN_POINT('Ctrl Pts',(-9.99429387455137,-2.08176008973396,
-29.6567839335205)) ;
#62050=CARTESIAN_POINT('Ctrl Pts',(-9.9965959799775,-2.11456004793966,-29.6631611025615)) ;
#62051=CARTESIAN_POINT('Ctrl Pts',(-9.99775126858592,-2.13108081334029,
-29.6663746002696)) ;
#62052=CARTESIAN_POINT('Ctrl Pts',(-10.000069122618,-2.16431561158016,-29.6728412905659)) ;
#62053=CARTESIAN_POINT('Ctrl Pts',(-10.001231671007,-2.18102964058034,-29.6760944880565)) ;
#62054=CARTESIAN_POINT('Ctrl Pts',(-10.0035620095714,-2.21460264917897,
-29.6826307269224)) ;
#62055=CARTESIAN_POINT('Ctrl Pts',(-10.0047297976087,-2.23146162878534,
-29.6859137690194)) ;
#62056=CARTESIAN_POINT('Ctrl Pts',(-10.0082373866525,-2.28218353208635,
-29.6957930848408)) ;
#62057=CARTESIAN_POINT('Ctrl Pts',(-10.0105814813601,-2.31619141997308,
-29.7024195248609)) ;
#62058=CARTESIAN_POINT('Ctrl Pts',(-10.0152591829867,-2.38420731419178,
-29.7156759644786)) ;
#62059=CARTESIAN_POINT('Ctrl Pts',(-10.0175927470763,-2.4182153068596,-29.7223059755272)) ;
#62060=CARTESIAN_POINT('Ctrl Pts',(-10.0222257294052,-2.48584491021547,
-29.7354932425945)) ;
#62061=CARTESIAN_POINT('Ctrl Pts',(-10.0245251307189,-2.51946652094906,
-29.7420505043261)) ;
#62062=CARTESIAN_POINT('Ctrl Pts',(-10.0313354853966,-2.61917207395672,
-29.7614990800057)) ;
#62063=CARTESIAN_POINT('Ctrl Pts',(-10.0357586991564,-2.68409673668246,
-29.7741671474126)) ;
#62064=CARTESIAN_POINT('Ctrl Pts',(-10.0445719574544,-2.81365376993385,
-29.7994507167258)) ;
#62065=CARTESIAN_POINT('Ctrl Pts',(-10.0491852821836,-2.8815893713073,-29.8127113376134)) ;
#62066=CARTESIAN_POINT('Ctrl Pts',(-10.0584279811638,-3.01787063373489,
-29.8393165952872)) ;
#62067=CARTESIAN_POINT('Ctrl Pts',(-10.0630573183518,-3.08621629486166,
-29.8526612445772)) ;
#62068=CARTESIAN_POINT('Ctrl Pts',(-10.0723337144261,-3.22330444615647,
-29.8794311103673)) ;
#62069=CARTESIAN_POINT('Ctrl Pts',(-10.0769807582795,-3.29204693631097,
-29.8928563319293)) ;
#62070=CARTESIAN_POINT('Ctrl Pts',(-10.0862933964167,-3.42991551634899,
-29.9197841780547)) ;
#62071=CARTESIAN_POINT('Ctrl Pts',(-10.0909589887703,-3.49904160623596,
-29.9332868032681)) ;
#62072=CARTESIAN_POINT('Ctrl Pts',(-10.104984095758,-3.70697543286987,-29.9739062863256)) ;
#62073=CARTESIAN_POINT('Ctrl Pts',(-10.114372043631,-3.84633872593528,-30.0011347166327)) ;
#62074=CARTESIAN_POINT('Ctrl Pts',(-10.133222992924,-4.1264409723699,-30.0558662853713)) ;
#62075=CARTESIAN_POINT('Ctrl Pts',(-10.1426859377833,-4.26717992581852,
-30.0833694428775)) ;
#62076=CARTESIAN_POINT('Ctrl Pts',(-10.1616835878252,-4.54992767301016,
-30.1386284989711)) ;
#62077=CARTESIAN_POINT('Ctrl Pts',(-10.1712182677189,-4.69193646584414,
-30.1663844058811)) ;
#62078=CARTESIAN_POINT('Ctrl Pts',(-10.1903548491206,-4.97711806982726,
-30.2221274129627)) ;
#62079=CARTESIAN_POINT('Ctrl Pts',(-10.1999567380201,-5.12029088099143,
-30.2501145173859)) ;
#62080=CARTESIAN_POINT('Ctrl Pts',(-10.219222463357,-5.40769470241093,-30.3062986200493)) ;
#62081=CARTESIAN_POINT('Ctrl Pts',(-10.2288862936133,-5.55192571266397,
-30.3344956203714)) ;
#62082=CARTESIAN_POINT('Ctrl Pts',(-10.2482701602761,-5.84134011352206,
-30.3910783729501)) ;
#62083=CARTESIAN_POINT('Ctrl Pts',(-10.2579901955671,-5.98652350412846,
-30.419464125582)) ;
#62084=CARTESIAN_POINT('Ctrl Pts',(-10.2872255418426,-6.4233435188767,-30.5048729525588)) ;
#62085=CARTESIAN_POINT('Ctrl Pts',(-10.3068161653109,-6.71624998125329,
-30.5621475706734)) ;
#62086=CARTESIAN_POINT('Ctrl Pts',(-10.3461475069765,-7.30460259096212,
-30.6772000749509)) ;
#62087=CARTESIAN_POINT('Ctrl Pts',(-10.3658881886828,-7.60004873832798,
-30.7349779734165)) ;
#62088=CARTESIAN_POINT('Ctrl Pts',(-10.4054670152996,-8.1926341663384,-30.8508701605798)) ;
#62089=CARTESIAN_POINT('Ctrl Pts',(-10.4253051421279,-8.48977344697968,
-30.9089844553695)) ;
#62090=CARTESIAN_POINT('Ctrl Pts',(-10.4650251857872,-9.08489859067703,
-31.0253829085238)) ;
#62091=CARTESIAN_POINT('Ctrl Pts',(-10.484907094154,-9.38288445374,-31.0836670697413)) ;
#62092=CARTESIAN_POINT('Ctrl Pts',(-10.5445370048436,-10.2768420911068,
-31.2585248923988)) ;
#62093=CARTESIAN_POINT('Ctrl Pts',(-10.584269340941,-10.8728138981643,-31.3751038395442)) ;
#62094=CARTESIAN_POINT('Ctrl Pts',(-10.6632528657959,-12.0579851834207,
-31.6069469781574)) ;
#62095=CARTESIAN_POINT('Ctrl Pts',(-10.7025039813133,-12.6471846616712,
-31.7222111943129)) ;
#62096=CARTESIAN_POINT('Ctrl Pts',(-10.7800820901393,-13.8120388654271,
-31.9500972327384)) ;
#62097=CARTESIAN_POINT('Ctrl Pts',(-10.8202961136303,-14.4160365127297,
-32.0682641126275)) ;
#62098=CARTESIAN_POINT('Ctrl Pts',(-10.8597565733816,-15.0088506100736,
-32.1842460492104)) ;
#62099=CARTESIAN_POINT('Ctrl Pts',(-10.861606591113,-15.0366437072151,-32.189683674969)) ;
#62100=CARTESIAN_POINT('Ctrl Pts',(-10.8335168657278,-15.0366437072152,
-32.1991482054211)) ;
#62101=CARTESIAN_POINT('Ctrl Pts',(-10.8316989411165,-15.0088506101081,
-32.1936997662387)) ;
#62102=CARTESIAN_POINT('Ctrl Pts',(-10.829879399171,-14.9810324825753,-32.188246413499)) ;
#62103=CARTESIAN_POINT('Ctrl Pts',(-10.7910704227901,-14.3876935910683,
-32.0719305223189)) ;
#62104=CARTESIAN_POINT('Ctrl Pts',(-10.7534264184998,-13.8120388656015,
-31.9590785742631)) ;
#62105=CARTESIAN_POINT('Ctrl Pts',(-10.6772750585336,-12.647184661918,-31.7307118081906)) ;
#62106=CARTESIAN_POINT('Ctrl Pts',(-10.6387676678708,-12.0579851837042,
-31.6151970019631)) ;
#62107=CARTESIAN_POINT('Ctrl Pts',(-10.5613404148593,-10.8728138985215,
-31.3828294943288)) ;
#62108=CARTESIAN_POINT('Ctrl Pts',(-10.5224204792644,-10.2768420915011,
-31.2659768175915)) ;
#62109=CARTESIAN_POINT('Ctrl Pts',(-10.4640719920794,-9.38288445418984,
-31.0906872330967)) ;
#62110=CARTESIAN_POINT('Ctrl Pts',(-10.4446277699413,-9.08489859114541,
-31.0322555982222)) ;
#62111=CARTESIAN_POINT('Ctrl Pts',(-10.405807278733,-8.48977344748511,-30.9155540505654)) ;
#62112=CARTESIAN_POINT('Ctrl Pts',(-10.3864310011991,-8.19263416686229,
-30.857284140634)) ;
#62113=CARTESIAN_POINT('Ctrl Pts',(-10.3478044672062,-7.6000487388887,-30.7410710887349)) ;
#62114=CARTESIAN_POINT('Ctrl Pts',(-10.3285541926651,-7.30460259154122,
-30.6831279528606)) ;
#62115=CARTESIAN_POINT('Ctrl Pts',(-10.2902387920502,-6.716249981869,-30.5677331381953)) ;
#62116=CARTESIAN_POINT('Ctrl Pts',(-10.2711736294812,-6.42334351951061,
-30.5102814716937)) ;
#62117=CARTESIAN_POINT('Ctrl Pts',(-10.2427604660902,-5.98652350478954,
-30.4245956190545)) ;
#62118=CARTESIAN_POINT('Ctrl Pts',(-10.2333201932118,-5.84134011419217,
-30.3961156034926)) ;
#62119=CARTESIAN_POINT('Ctrl Pts',(-10.2145091321644,-5.55192571335207,
-30.3393398502347)) ;
#62120=CARTESIAN_POINT('Ctrl Pts',(-10.2051383428801,-5.40769470310801,
-30.3110441129149)) ;
#62121=CARTESIAN_POINT('Ctrl Pts',(-10.1864744829921,-5.12029088170639,
-30.2546572181743)) ;
#62122=CARTESIAN_POINT('Ctrl Pts',(-10.1771814062092,-4.97711807055114,
-30.2265660628362)) ;
#62123=CARTESIAN_POINT('Ctrl Pts',(-10.1586816754023,-4.69193646658576,
-30.1706084758092)) ;
#62124=CARTESIAN_POINT('Ctrl Pts',(-10.1494750087662,-4.54992767376058,
-30.1427420483666)) ;
#62125=CARTESIAN_POINT('Ctrl Pts',(-10.1311575503266,-4.26717992658653,
-30.0872538090418)) ;
#62126=CARTESIAN_POINT('Ctrl Pts',(-10.1220467333525,-4.12644097314668,
-30.0596320058389)) ;
#62127=CARTESIAN_POINT('Ctrl Pts',(-10.1039317092101,-3.84633872672947,
-30.0046524750503)) ;
#62128=CARTESIAN_POINT('Ctrl Pts',(-10.0949274454705,-3.70697543367274,
-29.9772947665084)) ;
#62129=CARTESIAN_POINT('Ctrl Pts',(-10.0815108721089,-3.49904160705175,
-29.9364702446021)) ;
#62130=CARTESIAN_POINT('Ctrl Pts',(-10.0770536772167,-3.42991551716911,
-29.9228974021094)) ;
#62131=CARTESIAN_POINT('Ctrl Pts',(-10.0681713657158,-3.29204693713965,
-29.8958245620603)) ;
#62132=CARTESIAN_POINT('Ctrl Pts',(-10.0637462471753,-3.22330444698941,
-29.8823245651551)) ;
#62133=CARTESIAN_POINT('Ctrl Pts',(-10.0549306892449,-3.08621629570312,
-29.8553994249173)) ;
#62134=CARTESIAN_POINT('Ctrl Pts',(-10.0505402348198,-3.01787063458062,
-29.8419742866539)) ;
#62135=CARTESIAN_POINT('Ctrl Pts',(-10.0417974674542,-2.88158937216149,
-29.8152005824085)) ;
#62136=CARTESIAN_POINT('Ctrl Pts',(-10.0374451174447,-2.81365377079228,
-29.8018520289007)) ;
#62137=CARTESIAN_POINT('Ctrl Pts',(-10.0291603270341,-2.6840967373633,-29.7763903979855)) ;
#62138=CARTESIAN_POINT('Ctrl Pts',(-10.0250152290655,-2.61917207444665,
-29.7636286224163)) ;
#62139=CARTESIAN_POINT('Ctrl Pts',(-10.0186671286565,-2.51946652114585,
-29.7440242950753)) ;
#62140=CARTESIAN_POINT('Ctrl Pts',(-10.0165293803719,-2.48584491031341,
-29.737412566075)) ;
#62141=CARTESIAN_POINT('Ctrl Pts',(-10.0122370714667,-2.41821530675869,
-29.7241105127231)) ;
#62142=CARTESIAN_POINT('Ctrl Pts',(-10.0100824939169,-2.38420731399091,
-29.7174201940658)) ;
#62143=CARTESIAN_POINT('Ctrl Pts',(-10.0057839242904,-2.31619141957223,
-29.7040360099601)) ;
#62144=CARTESIAN_POINT('Ctrl Pts',(-10.0036398911843,-2.2821835315855,-29.6973421613161)) ;
#62145=CARTESIAN_POINT('Ctrl Pts',(-10.0004535512912,-2.23146162813537,
-29.6873546040206)) ;
#62146=CARTESIAN_POINT('Ctrl Pts',(-9.9993964068386,-2.21460264847951,-29.6840342817486)) ;
#62147=CARTESIAN_POINT('Ctrl Pts',(-9.99729600997807,-2.18102963978215,
-29.6774205664804)) ;
#62148=CARTESIAN_POINT('Ctrl Pts',(-9.99625275543195,-2.16431561073278,
-29.6741271742035)) ;
#62149=CARTESIAN_POINT('Ctrl Pts',(-9.99418450872342,-2.1310808123952,-29.6675763813864)) ;
#62150=CARTESIAN_POINT('Ctrl Pts',(-9.99315950002149,-2.11456004694601,
-29.6643189872563)) ;
#62151=CARTESIAN_POINT('Ctrl Pts',(-9.9911328919117,-2.08176008864388,-29.6578489923406)) ;
#62152=CARTESIAN_POINT('Ctrl Pts',(-9.99013124680192,-2.06548089558601,
-29.6546364069092)) ;
#62153=CARTESIAN_POINT('Ctrl Pts',(-9.98865144325748,-2.0412795197932,-29.6498573047625)) ;
#62154=CARTESIAN_POINT('Ctrl Pts',(-9.9881619769522,-2.03324863102629,-29.6482708920856)) ;
#62155=CARTESIAN_POINT('Ctrl Pts',(-9.98719185150007,-2.0172653660065,-29.6451122208414)) ;
#62156=CARTESIAN_POINT('Ctrl Pts',(-9.98671119156714,-2.00931298974907,
-29.6435399625384)) ;
#62157=CARTESIAN_POINT('Ctrl Pts',(-9.98576040682444,-1.99349279222591,
-29.6404103355341)) ;
#62158=CARTESIAN_POINT('Ctrl Pts',(-9.98529025485661,-1.98562497113475,
-29.6388529760218)) ;
#62159=CARTESIAN_POINT('Ctrl Pts',(-9.98459501202897,-1.97389119229962,
-29.636528391155)) ;
#62160=CARTESIAN_POINT('Ctrl Pts',(-9.98436493981971,-1.96999125825837,
-29.6357554348444)) ;
#62161=CARTESIAN_POINT('Ctrl Pts',(-9.98390871264385,-1.96221479880093,
-29.6342133071775)) ;
#62162=CARTESIAN_POINT('Ctrl Pts',(-9.983682555973,-1.95833827337143,-29.6334441363927)) ;
#62163=CARTESIAN_POINT('Ctrl Pts',(-9.98323473947911,-1.95060454181405,
-29.6319084927081)) ;
#62164=CARTESIAN_POINT('Ctrl Pts',(-9.98300116306043,-1.9465418535758,-29.6311012245421)) ;
#62165=CARTESIAN_POINT('Ctrl Pts',(-9.98252877745729,-1.93822324566284,
-29.6294463124608)) ;
#62166=CARTESIAN_POINT('Ctrl Pts',(-9.98228989910769,-1.93396732530918,
-29.6285986917018)) ;
#62167=CARTESIAN_POINT('Ctrl Pts',(-9.98193936904879,-1.92758370768641,
-29.6273246939941)) ;
#62168=CARTESIAN_POINT('Ctrl Pts',(-9.98182384014075,-1.92545589223065,
-29.6268995976523)) ;
#62169=CARTESIAN_POINT('Ctrl Pts',(-9.98159789955204,-1.92122455545407,
-29.6260529787085)) ;
#62170=CARTESIAN_POINT('Ctrl Pts',(-9.98148745389595,-1.91912103367696,
-29.6256314674547)) ;
#62171=CARTESIAN_POINT('Ctrl Pts',(-9.98132820722381,-1.91600211622353,
-29.6250049671436)) ;
#62172=CARTESIAN_POINT('Ctrl Pts',(-9.98127620657957,-1.91496854175463,
-29.6247970918333)) ;
#62173=CARTESIAN_POINT('Ctrl Pts',(-9.98117504271719,-1.91291654329207,
-29.6243836891066)) ;
#62174=CARTESIAN_POINT('Ctrl Pts',(-9.98112587708293,-1.91189811925535,
-29.624178162495)) ;
#62175=CARTESIAN_POINT('Ctrl Pts',(-9.9810314696815,-1.90987945010399,-29.6237697515287)) ;
#62176=CARTESIAN_POINT('Ctrl Pts',(-9.98098619082925,-1.90887920681535,
-29.6235668800677)) ;
#62177=CARTESIAN_POINT('Ctrl Pts',(-9.98092285308603,-1.90739476140765,
-29.6232645011586)) ;
#62178=CARTESIAN_POINT('Ctrl Pts',(-9.98090251330511,-1.90690260002959,
-29.6231640265195)) ;
#62179=CARTESIAN_POINT('Ctrl Pts',(-9.9808639831162,-1.90592397215236,-29.6229635949418)) ;
#62180=CARTESIAN_POINT('Ctrl Pts',(-9.98084576984047,-1.90543750500457,
-29.6228636455668)) ;
#62181=CARTESIAN_POINT('Ctrl Pts',(-9.98082073735356,-1.90470544204056,
-29.6227124356354)) ;
#62182=CARTESIAN_POINT('Ctrl Pts',(-9.98081223578881,-1.90444442082997,
-29.6226583780428)) ;
#62183=CARTESIAN_POINT('Ctrl Pts',(-9.98079629773457,-1.90391015043467,
-29.622547237381)) ;
#62184=CARTESIAN_POINT('Ctrl Pts',(-9.98078885639857,-1.90363690106332,
-29.6224901559041)) ;
#62185=CARTESIAN_POINT('Ctrl Pts',(-9.98077656125721,-1.90309071520488,
-29.6223751893419)) ;
#62186=CARTESIAN_POINT('Ctrl Pts',(-9.98077161921038,-1.90281781754094,
-29.622317342455)) ;
#62187=CARTESIAN_POINT('Ctrl Pts',(-9.98081728992659,-1.90163369721464,
-29.6220437275998)) ;
#62188=CARTESIAN_POINT('Ctrl Pts',(-9.98081916755763,-1.90158501523074,
-29.6220324786468)) ;
#62189=CARTESIAN_POINT('Ctrl Pts',(-9.98082104518866,-1.90153633324684,
-29.6220212296937)) ;
#62190=CARTESIAN_POINT('',(-23.3738245177975,-15.0366437072153,-24.6538954375548)) ;
#62191=CARTESIAN_POINT('',(-23.3523050271304,-15.0366437072153,-24.674279781881)) ;
#62192=CARTESIAN_POINT('Origin',(0.939357956114989,-21.6462763158693,0.99166813738465)) ;
#62193=CARTESIAN_POINT('',(-21.4963117156553,-1.90153624017924,-22.6933803539597)) ;
#62194=CARTESIAN_POINT('Ctrl Pts',(-21.4963117284258,-1.90153632878805,
-22.693380367086)) ;
#62195=CARTESIAN_POINT('Ctrl Pts',(-21.4963232866611,-1.90158488951342,
-22.6933832416551)) ;
#62196=CARTESIAN_POINT('Ctrl Pts',(-21.4965226828145,-1.90242263174387,
-22.6934328320992)) ;
#62197=CARTESIAN_POINT('Ctrl Pts',(-21.4965976870093,-1.90282441414894,
-22.6934761542018)) ;
#62198=CARTESIAN_POINT('Ctrl Pts',(-21.4966467084764,-1.90309873182999,
-22.6935078048281)) ;
#62199=CARTESIAN_POINT('Ctrl Pts',(-21.4967429748708,-1.9036477578842,-22.6935729001217)) ;
#62200=CARTESIAN_POINT('Ctrl Pts',(-21.4967901444201,-1.90392242741489,
-22.693606405134)) ;
#62201=CARTESIAN_POINT('Ctrl Pts',(-21.4968813060532,-1.90445947365899,
-22.6936729257873)) ;
#62202=CARTESIAN_POINT('Ctrl Pts',(-21.4969252944931,-1.90472185055691,
-22.6937059449324)) ;
#62203=CARTESIAN_POINT('Ctrl Pts',(-21.4970477581099,-1.90545775489615,
-22.6937994209599)) ;
#62204=CARTESIAN_POINT('Ctrl Pts',(-21.4971279264057,-1.90594678820076,
-22.6938626878748)) ;
#62205=CARTESIAN_POINT('Ctrl Pts',(-21.497287749129,-1.9069305782757,-22.6939913376866)) ;
#62206=CARTESIAN_POINT('Ctrl Pts',(-21.4973673860617,-1.90742533569666,
-22.6940567373406)) ;
#62207=CARTESIAN_POINT('Ctrl Pts',(-21.497606056854,-1.90891761107545,-22.6942554417845)) ;
#62208=CARTESIAN_POINT('Ctrl Pts',(-21.4977648791666,-1.90992313013283,
-22.694391224525)) ;
#62209=CARTESIAN_POINT('Ctrl Pts',(-21.4980830859284,-1.91195244645976,
-22.6946674605282)) ;
#62210=CARTESIAN_POINT('Ctrl Pts',(-21.4982424415412,-1.91297624190247,
-22.6948079405862)) ;
#62211=CARTESIAN_POINT('Ctrl Pts',(-21.4985619093448,-1.91503906287447,
-22.6950925193719)) ;
#62212=CARTESIAN_POINT('Ctrl Pts',(-21.4987220196732,-1.91607808844715,
-22.695236619876)) ;
#62213=CARTESIAN_POINT('Ctrl Pts',(-21.4992033798014,-1.91921345485071,
-22.6956731528048)) ;
#62214=CARTESIAN_POINT('Ctrl Pts',(-21.4995256903791,-1.92132807011153,
-22.6959697823368)) ;
#62215=CARTESIAN_POINT('Ctrl Pts',(-21.5001711350599,-1.92558172137742,
-22.6965692128324)) ;
#62216=CARTESIAN_POINT('Ctrl Pts',(-21.5004942431825,-1.92772075783832,
-22.6968720385356)) ;
#62217=CARTESIAN_POINT('Ctrl Pts',(-21.5014605714309,-1.93413803849897,
-22.6977834024756)) ;
#62218=CARTESIAN_POINT('Ctrl Pts',(-21.5021008361852,-1.93841640089627,
-22.6983947738345)) ;
#62219=CARTESIAN_POINT('Ctrl Pts',(-21.5033480901722,-1.94677887282856,
-22.6995937415208)) ;
#62220=CARTESIAN_POINT('Ctrl Pts',(-21.5039550263826,-1.95086298304285,
-22.7001813882667)) ;
#62221=CARTESIAN_POINT('Ctrl Pts',(-21.5051079743681,-1.95863767898893,
-22.7013023732685)) ;
#62222=CARTESIAN_POINT('Ctrl Pts',(-21.5056846047152,-1.96253483117455,
-22.7018655084924)) ;
#62223=CARTESIAN_POINT('Ctrl Pts',(-21.5068393899876,-1.97035266864422,
-22.7029970336256)) ;
#62224=CARTESIAN_POINT('Ctrl Pts',(-21.5074175436022,-1.97427335394165,
-22.7035654247798)) ;
#62225=CARTESIAN_POINT('Ctrl Pts',(-21.5091547200953,-1.98606956727156,
-22.7052777489694)) ;
#62226=CARTESIAN_POINT('Ctrl Pts',(-21.510316493032,-1.99397925232716,-22.7064288000193)) ;
#62227=CARTESIAN_POINT('Ctrl Pts',(-21.5126483548276,-2.00988362758461,
-22.7087472221003)) ;
#62228=CARTESIAN_POINT('Ctrl Pts',(-21.513818422781,-2.01787831761191,-22.7099146128845)) ;
#62229=CARTESIAN_POINT('Ctrl Pts',(-21.5161669917595,-2.03394662784809,
-22.7122638741884)) ;
#62230=CARTESIAN_POINT('Ctrl Pts',(-21.5173454921875,-2.0420202480614,-22.7134457452744)) ;
#62231=CARTESIAN_POINT('Ctrl Pts',(-21.5208932751436,-2.06635039651484,
-22.7170108341686)) ;
#62232=CARTESIAN_POINT('Ctrl Pts',(-21.5232749130048,-2.08271620910784,
-22.7194134568504)) ;
#62233=CARTESIAN_POINT('Ctrl Pts',(-21.5280670365947,-2.11569069163832,
-22.7242605069101)) ;
#62234=CARTESIAN_POINT('Ctrl Pts',(-21.5304774872622,-2.13229936178073,
-22.7267049675577)) ;
#62235=CARTESIAN_POINT('Ctrl Pts',(-21.5353217952499,-2.16571099763217,
-22.73162702433)) ;
#62236=CARTESIAN_POINT('Ctrl Pts',(-21.5377556391222,-2.18251395950177,
-22.7341046321001)) ;
#62237=CARTESIAN_POINT('Ctrl Pts',(-21.5426407161461,-2.21626560493476,
-22.7390848562231)) ;
#62238=CARTESIAN_POINT('Ctrl Pts',(-21.5450919476502,-2.23321428850602,
-22.7415874741381)) ;
#62239=CARTESIAN_POINT('Ctrl Pts',(-21.5524622515727,-2.28420607479834,
-22.7491210791498)) ;
#62240=CARTESIAN_POINT('Ctrl Pts',(-21.5573979862509,-2.31839491280777,
-22.7541777673676)) ;
#62241=CARTESIAN_POINT('Ctrl Pts',(-21.5672614105418,-2.38677270727805,
-22.7642987982121)) ;
#62242=CARTESIAN_POINT('Ctrl Pts',(-21.5721890660041,-2.42096165007377,
-22.7693631692978)) ;
#62243=CARTESIAN_POINT('Ctrl Pts',(-21.581982528211,-2.48895109743765,-22.7794399263397)) ;
#62244=CARTESIAN_POINT('Ctrl Pts',(-21.5868483219591,-2.52275160205135,
-22.7844523246197)) ;
#62245=CARTESIAN_POINT('Ctrl Pts',(-21.6012713504402,-2.62298766794955,
-22.7993229231962)) ;
#62246=CARTESIAN_POINT('Ctrl Pts',(-21.6106543166059,-2.68825778093597,
-22.809014447373)) ;
#62247=CARTESIAN_POINT('Ctrl Pts',(-21.6293728962788,-2.81853945706393,
-22.8283687527329)) ;
#62248=CARTESIAN_POINT('Ctrl Pts',(-21.6391845503111,-2.88687193745379,
-22.8385259240375)) ;
#62249=CARTESIAN_POINT('Ctrl Pts',(-21.6588580128413,-3.02394935341697,
-22.8589101657353)) ;
#62250=CARTESIAN_POINT('Ctrl Pts',(-21.6687197928116,-3.09269428906301,
-22.869137263172)) ;
#62251=CARTESIAN_POINT('Ctrl Pts',(-21.6884935733421,-3.23058330762132,
-22.8896575063169)) ;
#62252=CARTESIAN_POINT('Ctrl Pts',(-21.6984055623305,-3.29972739051995,
-22.8999506629822)) ;
#62253=CARTESIAN_POINT('Ctrl Pts',(-21.7182791782898,-3.43840139699515,
-22.9205997886577)) ;
#62254=CARTESIAN_POINT('Ctrl Pts',(-21.7282408037747,-3.50793132057516,
-22.930955759075)) ;
#62255=CARTESIAN_POINT('Ctrl Pts',(-21.758198695169,-3.71707989379933,-22.9621135734917)) ;
#62256=CARTESIAN_POINT('Ctrl Pts',(-21.7782680553984,-3.85725734527214,
-22.9830052452732)) ;
#62257=CARTESIAN_POINT('Ctrl Pts',(-21.8185913442818,-4.13899594502097,
-23.0250076342015)) ;
#62258=CARTESIAN_POINT('Ctrl Pts',(-21.8388452294421,-4.28055709337647,
-23.0461183925702)) ;
#62259=CARTESIAN_POINT('Ctrl Pts',(-21.8795252773123,-4.56495664868979,
-23.0885402989146)) ;
#62260=CARTESIAN_POINT('Ctrl Pts',(-21.8999514204951,-4.70779505473742,
-23.1098514651284)) ;
#62261=CARTESIAN_POINT('Ctrl Pts',(-21.9409627358116,-4.99464268526103,
-23.1526564380478)) ;
#62262=CARTESIAN_POINT('Ctrl Pts',(-21.9615478982523,-5.13865190975205,
-23.1741502539394)) ;
#62263=CARTESIAN_POINT('Ctrl Pts',(-22.0028634384497,-5.42773473974678,
-23.217303313115)) ;
#62264=CARTESIAN_POINT('Ctrl Pts',(-22.023593811453,-5.57280834524819,-23.2389625609007)) ;
#62265=CARTESIAN_POINT('Ctrl Pts',(-22.0651855999471,-5.86391350033323,
-23.2824296111504)) ;
#62266=CARTESIAN_POINT('Ctrl Pts',(-22.0860470145812,-6.00994504991818,
-23.3042374144253)) ;
#62267=CARTESIAN_POINT('Ctrl Pts',(-22.1488062119652,-6.4493169599107,-23.3698586798306)) ;
#62268=CARTESIAN_POINT('Ctrl Pts',(-22.1908790031683,-6.7439345768575,-23.4138699441313)) ;
#62269=CARTESIAN_POINT('Ctrl Pts',(-22.2753741970227,-7.33572433231973,
-23.502288463561)) ;
#62270=CARTESIAN_POINT('Ctrl Pts',(-22.3177965716302,-7.63289647086886,
-23.5466957452641)) ;
#62271=CARTESIAN_POINT('Ctrl Pts',(-22.4028723995403,-8.22894377232508,
-23.6357761957328)) ;
#62272=CARTESIAN_POINT('Ctrl Pts',(-22.4455258389439,-8.52781893522888,
-23.6804493776631)) ;
#62273=CARTESIAN_POINT('Ctrl Pts',(-22.5309444631914,-9.12642078899722,
-23.7699322833272)) ;
#62274=CARTESIAN_POINT('Ctrl Pts',(-22.5737096415316,-9.42614747986867,
-23.8147420132228)) ;
#62275=CARTESIAN_POINT('Ctrl Pts',(-22.7019930343727,-10.3253276006806,
-23.9491827183168)) ;
#62276=CARTESIAN_POINT('Ctrl Pts',(-22.7874992191758,-10.9247810633858,
-24.0388250979726)) ;
#62277=CARTESIAN_POINT('Ctrl Pts',(-22.9575171690251,-12.1168760956996,
-24.2171127741637)) ;
#62278=CARTESIAN_POINT('Ctrl Pts',(-23.0420288777932,-12.7095176653597,
-24.3057581240216)) ;
#62279=CARTESIAN_POINT('Ctrl Pts',(-23.2094672465774,-13.8838032558862,
-24.4814197413028)) ;
#62280=CARTESIAN_POINT('Ctrl Pts',(-23.2923850750004,-14.4653860626283,
-24.5684269494759)) ;
#62281=CARTESIAN_POINT('Ctrl Pts',(-23.3738245177983,-15.0366437072153,
-24.6538954375541)) ;
#62282=CARTESIAN_POINT('Ctrl Pts',(-23.3523050271281,-15.0366437072153,
-24.6742797818832)) ;
#62283=CARTESIAN_POINT('Ctrl Pts',(-23.3519438108906,-15.0340941324353,
-24.6738961918291)) ;
#62284=CARTESIAN_POINT('Ctrl Pts',(-23.3515825656427,-15.0315443519866,
-24.6735125707103)) ;
#62285=CARTESIAN_POINT('Ctrl Pts',(-23.2706354764949,-14.4601946119446,
-24.58755148494)) ;
#62286=CARTESIAN_POINT('Ctrl Pts',(-23.1886083812775,-13.8811769235724,
-24.500430706285)) ;
#62287=CARTESIAN_POINT('Ctrl Pts',(-23.0226413408112,-12.7095176655682,
-24.324122974606)) ;
#62288=CARTESIAN_POINT('Ctrl Pts',(-22.9387013686766,-12.116876095939,-24.2349360470503)) ;
#62289=CARTESIAN_POINT('Ctrl Pts',(-22.7698797529755,-10.9247810636875,
-24.0555151429776)) ;
#62290=CARTESIAN_POINT('Ctrl Pts',(-22.6849980531189,-10.3253276010136,
-23.965281219768)) ;
#62291=CARTESIAN_POINT('Ctrl Pts',(-22.5576996397855,-9.42614748024864,
-23.8299074925378)) ;
#62292=CARTESIAN_POINT('Ctrl Pts',(-22.5152708873019,-9.12642078939284,
-23.7847790831478)) ;
#62293=CARTESIAN_POINT('Ctrl Pts',(-22.430543687122,-8.52781893565576,-23.6946412258264)) ;
#62294=CARTESIAN_POINT('Ctrl Pts',(-22.3882452329189,-8.22894377276754,
-23.6496317840573)) ;
#62295=CARTESIAN_POINT('Ctrl Pts',(-22.3039013390795,-7.63289647134248,
-23.5598580088181)) ;
#62296=CARTESIAN_POINT('Ctrl Pts',(-22.2618558855447,-7.33572433280887,
-23.5150936885143)) ;
#62297=CARTESIAN_POINT('Ctrl Pts',(-22.1781415170712,-6.74393457737753,
-23.4259355320049)) ;
#62298=CARTESIAN_POINT('Ctrl Pts',(-22.1364725740781,-6.44931696044613,
-23.3815417223642)) ;
#62299=CARTESIAN_POINT('Ctrl Pts',(-22.0743452623651,-6.00994505047655,
-23.3153219030641)) ;
#62300=CARTESIAN_POINT('Ctrl Pts',(-22.053698856334,-5.86391350089923,-23.2933104328244)) ;
#62301=CARTESIAN_POINT('Ctrl Pts',(-22.0125472882954,-5.5728083458294,-23.2494263836136)) ;
#62302=CARTESIAN_POINT('Ctrl Pts',(-21.9920421254311,-5.42773474033559,
-23.2275538054548)) ;
#62303=CARTESIAN_POINT('Ctrl Pts',(-21.9511891321905,-5.13865191035594,
-23.1839625985327)) ;
#62304=CARTESIAN_POINT('Ctrl Pts',(-21.9308412970635,-4.99464268587244,
-23.1622439742704)) ;
#62305=CARTESIAN_POINT('Ctrl Pts',(-21.8903194091775,-4.70779505536381,
-23.1189753910673)) ;
#62306=CARTESIAN_POINT('Ctrl Pts',(-21.8701453467194,-4.56495664932364,
-23.0974254413096)) ;
#62307=CARTESIAN_POINT('Ctrl Pts',(-21.82998802915,-4.28055709402517,-23.0545083785269)) ;
#62308=CARTESIAN_POINT('Ctrl Pts',(-21.8100047547694,-4.13899594567707,
-23.0331412840139)) ;
#62309=CARTESIAN_POINT('Ctrl Pts',(-21.7702470248157,-3.85725734594295,
-22.9906031692151)) ;
#62310=CARTESIAN_POINT('Ctrl Pts',(-21.7504725257305,-3.71707989447745,
-22.9694321901238)) ;
#62311=CARTESIAN_POINT('Ctrl Pts',(-21.720982294478,-3.50793132126421,-22.9378313844934)) ;
#62312=CARTESIAN_POINT('Ctrl Pts',(-21.7111808235151,-3.43840139768783,
-22.9273237076555)) ;
#62313=CARTESIAN_POINT('Ctrl Pts',(-21.69163791744,-3.29972739121987,-22.9063613169399)) ;
#62314=CARTESIAN_POINT('Ctrl Pts',(-21.681896480842,-3.23058330832484,-22.8959066044699)) ;
#62315=CARTESIAN_POINT('Ctrl Pts',(-21.6624768632991,-3.09269428977375,
-22.8750508803254)) ;
#62316=CARTESIAN_POINT('Ctrl Pts',(-21.6527986707855,-3.02394935413129,
-22.8646498796134)) ;
#62317=CARTESIAN_POINT('Ctrl Pts',(-21.6335094241247,-2.88687193817528,
-22.843901689314)) ;
#62318=CARTESIAN_POINT('Ctrl Pts',(-21.6238983414308,-2.81853945778899,
-22.8335545267469)) ;
#62319=CARTESIAN_POINT('Ctrl Pts',(-21.6055858243229,-2.68825778181904,
-22.8138155785391)) ;
#62320=CARTESIAN_POINT('Ctrl Pts',(-21.5964164971659,-2.62298766899475,
-22.80392168479)) ;
#62321=CARTESIAN_POINT('Ctrl Pts',(-21.582348554658,-2.5227516033456,-22.7887147309843)) ;
#62322=CARTESIAN_POINT('Ctrl Pts',(-21.5776069362756,-2.48895109881591,
-22.7835847075738)) ;
#62323=CARTESIAN_POINT('Ctrl Pts',(-21.5680751650442,-2.42096165162096,
-22.7732600637207)) ;
#62324=CARTESIAN_POINT('Ctrl Pts',(-21.5632849991904,-2.38677270891016,
-22.7680654555843)) ;
#62325=CARTESIAN_POINT('Ctrl Pts',(-21.5537128067588,-2.31839491460977,
-22.7576685553175)) ;
#62326=CARTESIAN_POINT('Ctrl Pts',(-21.5489307499096,-2.28420607668529,
-22.7524662957519)) ;
#62327=CARTESIAN_POINT('Ctrl Pts',(-21.5418072138063,-2.23321429051965,
-22.7446989398817)) ;
#62328=CARTESIAN_POINT('Ctrl Pts',(-21.5394409731948,-2.21626560699046,
-22.7421158143287)) ;
#62329=CARTESIAN_POINT('Ctrl Pts',(-21.5347325257493,-2.18251396164137,
-22.7369682778057)) ;
#62330=CARTESIAN_POINT('Ctrl Pts',(-21.5323903172678,-2.16571099981351,
-22.7344038683946)) ;
#62331=CARTESIAN_POINT('Ctrl Pts',(-21.5277377446746,-2.13229936404508,
-22.729300190233)) ;
#62332=CARTESIAN_POINT('Ctrl Pts',(-21.5254273682071,-2.11569069394391,
-22.7267609342797)) ;
#62333=CARTESIAN_POINT('Ctrl Pts',(-21.5208468671157,-2.08271621149533,
-22.7217134247648)) ;
#62334=CARTESIAN_POINT('Ctrl Pts',(-21.5185767073711,-2.06635039894304,
-22.7192052044134)) ;
#62335=CARTESIAN_POINT('Ctrl Pts',(-21.5152089200917,-2.04202025055005,
-22.7154696145748)) ;
#62336=CARTESIAN_POINT('Ctrl Pts',(-21.5140925850502,-2.03394663035677,
-22.7142288573126)) ;
#62337=CARTESIAN_POINT('Ctrl Pts',(-21.5118739181062,-2.01787832016053,
-22.7117565462768)) ;
#62338=CARTESIAN_POINT('Ctrl Pts',(-21.5107715856034,-2.00988363015303,
-22.7105249930715)) ;
#62339=CARTESIAN_POINT('Ctrl Pts',(-21.5085828081459,-1.9939792549351,-22.7080710343171)) ;
#62340=CARTESIAN_POINT('Ctrl Pts',(-21.5074963423416,-1.98606956989922,
-22.706848648568)) ;
#62341=CARTESIAN_POINT('Ctrl Pts',(-21.5058805782652,-1.97427335659861,
-22.7050213164367)) ;
#62342=CARTESIAN_POINT('Ctrl Pts',(-21.5053443213055,-1.97035267131085,
-22.7044132386656)) ;
#62343=CARTESIAN_POINT('Ctrl Pts',(-21.5042769744681,-1.96253483386059,
-22.7031988874529)) ;
#62344=CARTESIAN_POINT('Ctrl Pts',(-21.5037458832862,-1.95863768168481,
-22.7025926152431)) ;
#62345=CARTESIAN_POINT('Ctrl Pts',(-21.5026889616459,-1.95086298569985,
-22.7013806692445)) ;
#62346=CARTESIAN_POINT('Ctrl Pts',(-21.502135035599,-1.9467788754347,-22.7007428085899)) ;
#62347=CARTESIAN_POINT('Ctrl Pts',(-21.5010053512569,-1.93841640339806,
-22.6994324729907)) ;
#62348=CARTESIAN_POINT('Ctrl Pts',(-21.5004295397412,-1.93413804094723,
-22.6987600482659)) ;
#62349=CARTESIAN_POINT('Ctrl Pts',(-21.4995718283387,-1.92772076020648,
-22.6977457969615)) ;
#62350=CARTESIAN_POINT('Ctrl Pts',(-21.4992869394374,-1.92558172371826,
-22.6974067680811)) ;
#62351=CARTESIAN_POINT('Ctrl Pts',(-21.4987233317185,-1.92132807239916,
-22.6967298174825)) ;
#62352=CARTESIAN_POINT('Ctrl Pts',(-21.4984445867594,-1.91921345711195,
-22.696391920397)) ;
#62353=CARTESIAN_POINT('Ctrl Pts',(-21.4980347543484,-1.91607809066923,
-22.6958876328044)) ;
#62354=CARTESIAN_POINT('Ctrl Pts',(-21.4978995333845,-1.91503906508375,
-22.6957199558382)) ;
#62355=CARTESIAN_POINT('Ctrl Pts',(-21.4976326675899,-1.9129762440859,-22.6953855497755)) ;
#62356=CARTESIAN_POINT('Ctrl Pts',(-21.4975010209054,-1.91195244863063,
-22.6952188224229)) ;
#62357=CARTESIAN_POINT('Ctrl Pts',(-21.4972424173842,-1.90992313227818,
-22.694886127224)) ;
#62358=CARTESIAN_POINT('Ctrl Pts',(-21.4971154322506,-1.90891761320832,
-22.6947201867021)) ;
#62359=CARTESIAN_POINT('Ctrl Pts',(-21.4969299405941,-1.90742533781066,
-22.6944711082995)) ;
#62360=CARTESIAN_POINT('Ctrl Pts',(-21.4968689482557,-1.90693058038146,
-22.6943880475454)) ;
#62361=CARTESIAN_POINT('Ctrl Pts',(-21.4967491397467,-1.90594679029413,
-22.694221494253)) ;
#62362=CARTESIAN_POINT('Ctrl Pts',(-21.4966903059277,-1.90545775698652,
-22.6941380182473)) ;
#62363=CARTESIAN_POINT('Ctrl Pts',(-21.4966035970227,-1.90472185252296,
-22.6940106735224)) ;
#62364=CARTESIAN_POINT('Ctrl Pts',(-21.4965730077366,-1.9044594754992,-22.6939649619888)) ;
#62365=CARTESIAN_POINT('Ctrl Pts',(-21.4965115200034,-1.90392242900148,
-22.6938703326523)) ;
#62366=CARTESIAN_POINT('Ctrl Pts',(-21.4964806178287,-1.90364775934146,
-22.6938214183275)) ;
#62367=CARTESIAN_POINT('Ctrl Pts',(-21.4964208297127,-1.90309873302708,
-22.693721768899)) ;
#62368=CARTESIAN_POINT('Ctrl Pts',(-21.4963918793817,-1.90282441521009,
-22.693671105844)) ;
#62369=CARTESIAN_POINT('Ctrl Pts',(-21.4963177870611,-1.90163369563563,
-22.6934023441179)) ;
#62370=CARTESIAN_POINT('Ctrl Pts',(-21.4963147577435,-1.90158501221184,
-22.6933913556019)) ;
#62371=CARTESIAN_POINT('Ctrl Pts',(-21.4963117284258,-1.90153632878805,
-22.693380367086)) ;
#62372=CARTESIAN_POINT('',(-31.5654106012916,-15.0366437072153,-12.5608553214559)) ;
#62373=CARTESIAN_POINT('',(-31.5544392045422,-15.0366437072153,-12.5883914509173)) ;
#62374=CARTESIAN_POINT('Origin',(1.26892883449471,-21.6462763158693,0.505587457724594)) ;
#62375=CARTESIAN_POINT('',(-29.0382272152461,-1.90153624159665,-11.5698871852821)) ;
#62376=CARTESIAN_POINT('Ctrl Pts',(-29.0382272326218,-1.90153633162286,
-11.5698871919368)) ;
#62377=CARTESIAN_POINT('Ctrl Pts',(-29.0382389339435,-1.90158489075259,
-11.5698849358364)) ;
#62378=CARTESIAN_POINT('Ctrl Pts',(-29.038439954612,-1.9024191032399,-11.5698461775814)) ;
#62379=CARTESIAN_POINT('Ctrl Pts',(-29.0385258858908,-1.90281925831921,
-11.5698539247859)) ;
#62380=CARTESIAN_POINT('Ctrl Pts',(-29.0385834427646,-1.90309246582992,
-11.5698620077834)) ;
#62381=CARTESIAN_POINT('Ctrl Pts',(-29.0386976993411,-1.90363927141272,
-11.569880543178)) ;
#62382=CARTESIAN_POINT('Ctrl Pts',(-29.0387543560843,-1.90391283065899,
-11.5698910817176)) ;
#62383=CARTESIAN_POINT('Ctrl Pts',(-29.0388645914481,-1.90444770673756,
-11.569913048999)) ;
#62384=CARTESIAN_POINT('Ctrl Pts',(-29.0389181682581,-1.90470902375223,
-11.5699244823868)) ;
#62385=CARTESIAN_POINT('Ctrl Pts',(-29.0390679674835,-1.90544192542839,
-11.5699577154286)) ;
#62386=CARTESIAN_POINT('Ctrl Pts',(-29.0391668949579,-1.90592895304488,
-11.5699813481566)) ;
#62387=CARTESIAN_POINT('Ctrl Pts',(-29.0393651689924,-1.90690870838148,
-11.5700307443233)) ;
#62388=CARTESIAN_POINT('Ctrl Pts',(-29.0394645067144,-1.90740143675332,
-11.570056530308)) ;
#62389=CARTESIAN_POINT('Ctrl Pts',(-29.0397633492989,-1.90888759228089,
-11.5701362566965)) ;
#62390=CARTESIAN_POINT('Ctrl Pts',(-29.0399636978026,-1.90988898783355,
-11.5701925287128)) ;
#62391=CARTESIAN_POINT('Ctrl Pts',(-29.0403668539109,-1.91190998240188,
-11.5703090644009)) ;
#62392=CARTESIAN_POINT('Ctrl Pts',(-29.0405696466344,-1.91292957959075,
-11.5703693644013)) ;
#62393=CARTESIAN_POINT('Ctrl Pts',(-29.0409774276981,-1.91498394176463,
-11.570492922451)) ;
#62394=CARTESIAN_POINT('Ctrl Pts',(-29.0411824151165,-1.91601870679206,
-11.5705561828368)) ;
#62395=CARTESIAN_POINT('Ctrl Pts',(-29.0418000753912,-1.91914121681058,
-11.5707493624156)) ;
#62396=CARTESIAN_POINT('Ctrl Pts',(-29.0422154605921,-1.9212471614821,-11.5708826355584)) ;
#62397=CARTESIAN_POINT('Ctrl Pts',(-29.043049553386,-1.92548337189837,-11.5711544224452)) ;
#62398=CARTESIAN_POINT('Ctrl Pts',(-29.0434682478049,-1.92761363809929,
-11.5712929695085)) ;
#62399=CARTESIAN_POINT('Ctrl Pts',(-29.044722827206,-1.93400460796368,-11.5717124807114)) ;
#62400=CARTESIAN_POINT('Ctrl Pts',(-29.0455572226705,-1.93826542981638,
-11.5719972492473)) ;
#62401=CARTESIAN_POINT('Ctrl Pts',(-29.0471859897073,-1.94659361793648,
-11.5725592267218)) ;
#62402=CARTESIAN_POINT('Ctrl Pts',(-29.0479803343802,-1.95066098488323,
-11.5728365035519)) ;
#62403=CARTESIAN_POINT('Ctrl Pts',(-29.0494912134324,-1.95840366317408,
-11.5733674500498)) ;
#62404=CARTESIAN_POINT('Ctrl Pts',(-29.0502478839205,-1.96228469345615,
-11.5736352446663)) ;
#62405=CARTESIAN_POINT('Ctrl Pts',(-29.0517647982348,-1.97007018980902,
-11.5741749503929)) ;
#62406=CARTESIAN_POINT('Ctrl Pts',(-29.0525250413989,-1.97397465589319,
-11.5744468631722)) ;
#62407=CARTESIAN_POINT('Ctrl Pts',(-29.0548112132387,-1.98572207032782,
-11.5752679344914)) ;
#62408=CARTESIAN_POINT('Ctrl Pts',(-29.0563426017227,-1.99359903444582,
-11.5758223819579)) ;
#62409=CARTESIAN_POINT('Ctrl Pts',(-29.0594197151388,-2.00943761625919,
-11.5769425597229)) ;
#62410=CARTESIAN_POINT('Ctrl Pts',(-29.0609654294151,-2.01739923378007,
-11.5775083166679)) ;
#62411=CARTESIAN_POINT('Ctrl Pts',(-29.0640705317916,-2.03340107254685,
-11.5786493986402)) ;
#62412=CARTESIAN_POINT('Ctrl Pts',(-29.0656299195902,-2.04144129379721,
-11.5792247244255)) ;
#62413=CARTESIAN_POINT('Ctrl Pts',(-29.070327323818,-2.06567079334489,-11.5809631771912)) ;
#62414=CARTESIAN_POINT('Ctrl Pts',(-29.073484618138,-2.08196890397857,-11.5821386846341)) ;
#62415=CARTESIAN_POINT('Ctrl Pts',(-29.0798427548892,-2.11480697810897,
-11.5845154356313)) ;
#62416=CARTESIAN_POINT('Ctrl Pts',(-29.0830435795052,-2.13134694181059,
-11.5857167240125)) ;
#62417=CARTESIAN_POINT('Ctrl Pts',(-29.0894802354408,-2.16462036119451,
-11.5881394728866)) ;
#62418=CARTESIAN_POINT('Ctrl Pts',(-29.09271605946,-2.18135381303769,-11.5893609495587)) ;
#62419=CARTESIAN_POINT('Ctrl Pts',(-29.0992138781996,-2.21496583572871,
-11.5918192436418)) ;
#62420=CARTESIAN_POINT('Ctrl Pts',(-29.1024758720817,-2.23184440658444,
-11.5930560631602)) ;
#62421=CARTESIAN_POINT('Ctrl Pts',(-29.1122876293211,-2.2826252520403,-11.5967828618532)) ;
#62422=CARTESIAN_POINT('Ctrl Pts',(-29.1188631951064,-2.31667265923911,
-11.5992891136516)) ;
#62423=CARTESIAN_POINT('Ctrl Pts',(-29.1320102476389,-2.38476759208326,
-11.6043119209944)) ;
#62424=CARTESIAN_POINT('Ctrl Pts',(-29.138581715377,-2.41881510406427,-11.6068285166186)) ;
#62425=CARTESIAN_POINT('Ctrl Pts',(-29.1516470060032,-2.48652329696422,
-11.6118406024886)) ;
#62426=CARTESIAN_POINT('Ctrl Pts',(-29.1581408222881,-2.52018397792869,
-11.6143361093325)) ;
#62427=CARTESIAN_POINT('Ctrl Pts',(-29.1773950156982,-2.62000539438071,
-11.6217449858488)) ;
#62428=CARTESIAN_POINT('Ctrl Pts',(-29.1899281801797,-2.68500550307164,
-11.6265806038851)) ;
#62429=CARTESIAN_POINT('Ctrl Pts',(-29.2149343835133,-2.81472076277575,
-11.6362436435832)) ;
#62430=CARTESIAN_POINT('Ctrl Pts',(-29.2280443982007,-2.88274300721894,
-11.6413188248167)) ;
#62431=CARTESIAN_POINT('Ctrl Pts',(-29.2543389486577,-3.0191980787507,-11.6515113939421)) ;
#62432=CARTESIAN_POINT('Ctrl Pts',(-29.2675234699474,-3.08763090591191,
-11.6566288182163)) ;
#62433=CARTESIAN_POINT('Ctrl Pts',(-29.2939654853015,-3.22489389536975,
-11.6669023629037)) ;
#62434=CARTESIAN_POINT('Ctrl Pts',(-29.3072229734857,-3.29372405765274,
-11.6720584980668)) ;
#62435=CARTESIAN_POINT('Ctrl Pts',(-29.3338090447939,-3.43176847117171,
-11.6824067818085)) ;
#62436=CARTESIAN_POINT('Ctrl Pts',(-29.3471376271619,-3.50098272241108,
-11.6875989322834)) ;
#62437=CARTESIAN_POINT('Ctrl Pts',(-29.3872269113491,-3.70918174163314,
-11.7032261047598)) ;
#62438=CARTESIAN_POINT('Ctrl Pts',(-29.4140911905175,-3.84872277446492,
-11.7137117463827)) ;
#62439=CARTESIAN_POINT('Ctrl Pts',(-29.4680780422506,-4.1291822548889,-11.7348038136094)) ;
#62440=CARTESIAN_POINT('Ctrl Pts',(-29.4952005927186,-4.27010070256046,
-11.7454102947159)) ;
#62441=CARTESIAN_POINT('Ctrl Pts',(-29.5496850877767,-4.5532090576965,-11.7667323167097)) ;
#62442=CARTESIAN_POINT('Ctrl Pts',(-29.5770470223282,-4.69539896425168,
-11.7774478822838)) ;
#62443=CARTESIAN_POINT('Ctrl Pts',(-29.6319908991029,-4.98094428021694,
-11.7989775706329)) ;
#62444=CARTESIAN_POINT('Ctrl Pts',(-29.6595728364002,-5.12429968964207,
-11.8097917057789)) ;
#62445=CARTESIAN_POINT('Ctrl Pts',(-29.7149370452325,-5.41207005716519,
-11.8315087525043)) ;
#62446=CARTESIAN_POINT('Ctrl Pts',(-29.742719314352,-5.55648501526087,-11.8424116701445)) ;
#62447=CARTESIAN_POINT('Ctrl Pts',(-29.7984643308215,-5.846268526428,-11.8642969595879)) ;
#62448=CARTESIAN_POINT('Ctrl Pts',(-29.8264270777348,-5.99163707950077,
-11.875279332486)) ;
#62449=CARTESIAN_POINT('Ctrl Pts',(-29.9105560733675,-6.42901420114677,
-11.9083320971568)) ;
#62450=CARTESIAN_POINT('Ctrl Pts',(-29.966963104371,-6.72229422745249,-11.9305080635348)) ;
#62451=CARTESIAN_POINT('Ctrl Pts',(-30.0802585252516,-7.31139720401595,
-11.9750716664965)) ;
#62452=CARTESIAN_POINT('Ctrl Pts',(-30.137146900872,-7.60722015430732,-11.9974593388803)) ;
#62453=CARTESIAN_POINT('Ctrl Pts',(-30.2512435436636,-8.20056134750055,
-12.0423783485521)) ;
#62454=CARTESIAN_POINT('Ctrl Pts',(-30.3084518037675,-8.49807959039912,
-12.0649097035758)) ;
#62455=CARTESIAN_POINT('Ctrl Pts',(-30.4230263411922,-9.0939637382783,-12.1100490952004)) ;
#62456=CARTESIAN_POINT('Ctrl Pts',(-30.4803926152054,-9.39232964326583,
-12.1326571401055)) ;
#62457=CARTESIAN_POINT('Ctrl Pts',(-30.6524852649241,-10.2874274064106,
-12.2004967930873)) ;
#62458=CARTESIAN_POINT('Ctrl Pts',(-30.7672055236576,-10.8841592973239,
-12.2457437718867)) ;
#62459=CARTESIAN_POINT('Ctrl Pts',(-30.9953308302806,-12.0708421129822,
-12.3357526452282)) ;
#62460=CARTESIAN_POINT('Ctrl Pts',(-31.1087358495527,-12.6607930377786,
-12.3805146116206)) ;
#62461=CARTESIAN_POINT('Ctrl Pts',(-31.3329303683718,-13.8271328599994,
-12.4690309217136)) ;
#62462=CARTESIAN_POINT('Ctrl Pts',(-31.4480866112795,-14.4262400709299,
-12.5145098743794)) ;
#62463=CARTESIAN_POINT('Ctrl Pts',(-31.5611271543905,-15.0143581154364,
-12.5591632555183)) ;
#62464=CARTESIAN_POINT('Ctrl Pts',(-31.5654106013656,-15.0366437072152,
-12.5608553212698)) ;
#62465=CARTESIAN_POINT('Ctrl Pts',(-31.554439204468,-15.0366437072152,-12.5883914511032)) ;
#62466=CARTESIAN_POINT('Ctrl Pts',(-31.5501658085698,-15.014358115422,-12.5866741590429)) ;
#62467=CARTESIAN_POINT('Ctrl Pts',(-31.5458893477546,-14.9920565141722,
-12.5849556207893)) ;
#62468=CARTESIAN_POINT('Ctrl Pts',(-31.4330345428413,-14.4035217573628,
-12.5396034090853)) ;
#62469=CARTESIAN_POINT('Ctrl Pts',(-31.3225120134546,-13.8271328599263,
-12.4951790208008)) ;
#62470=CARTESIAN_POINT('Ctrl Pts',(-31.0988751849215,-12.6607930376751,
-12.4052630136179)) ;
#62471=CARTESIAN_POINT('Ctrl Pts',(-30.9857608721003,-12.0708421128632,
-12.3597714290424)) ;
#62472=CARTESIAN_POINT('Ctrl Pts',(-30.7582438744036,-10.8841592971741,
-12.2682358154036)) ;
#62473=CARTESIAN_POINT('Ctrl Pts',(-30.6438411608924,-10.2874274062452,
-12.2221918581842)) ;
#62474=CARTESIAN_POINT('Ctrl Pts',(-30.4722493803547,-9.39232964307708,
-12.1530951183366)) ;
#62475=CARTESIAN_POINT('Ctrl Pts',(-30.4150541837849,-9.09396373808178,
-12.1300577014212)) ;
#62476=CARTESIAN_POINT('Ctrl Pts',(-30.3008312509292,-8.49807959018708,
-12.0840358488622)) ;
#62477=CARTESIAN_POINT('Ctrl Pts',(-30.2438035113338,-8.20056134728074,
-12.0610514215222)) ;
#62478=CARTESIAN_POINT('Ctrl Pts',(-30.130079084377,-7.60722015407205,-12.0151982205396)) ;
#62479=CARTESIAN_POINT('Ctrl Pts',(-30.0733823899492,-7.31139720377296,
-11.9923294646345)) ;
#62480=CARTESIAN_POINT('Ctrl Pts',(-29.9604840594901,-6.72229422719415,
-11.9467692398571)) ;
#62481=CARTESIAN_POINT('Ctrl Pts',(-29.9042824091886,-6.42901420088078,
-11.9240778067818)) ;
#62482=CARTESIAN_POINT('Ctrl Pts',(-29.8204747692394,-5.99163707922339,
-11.890218500157)) ;
#62483=CARTESIAN_POINT('Ctrl Pts',(-29.7926213691401,-5.84626852614684,
-11.878961687448)) ;
#62484=CARTESIAN_POINT('Ctrl Pts',(-29.7371002367776,-5.55648501497217,
-11.8565144912627)) ;
#62485=CARTESIAN_POINT('Ctrl Pts',(-29.7094325040801,-5.41207005687272,
-11.8453241088778)) ;
#62486=CARTESIAN_POINT('Ctrl Pts',(-29.6543035367715,-5.12429968934209,
-11.8230166504439)) ;
#62487=CARTESIAN_POINT('Ctrl Pts',(-29.6268422997454,-4.98094427991323,
-11.8118995804582)) ;
#62488=CARTESIAN_POINT('Ctrl Pts',(-29.5721473378698,-4.69539896394052,
-11.7897451628163)) ;
#62489=CARTESIAN_POINT('Ctrl Pts',(-29.5449136080874,-4.55320905738164,
-11.7787078275328)) ;
#62490=CARTESIAN_POINT('Ctrl Pts',(-29.4906949673073,-4.27010070223822,
-11.7567185616112)) ;
#62491=CARTESIAN_POINT('Ctrl Pts',(-29.4637100466217,-4.129182254563,-11.7457666557959)) ;
#62492=CARTESIAN_POINT('Ctrl Pts',(-29.4100108324211,-3.84872277413171,
-11.723952672795)) ;
#62493=CARTESIAN_POINT('Ctrl Pts',(-29.3832965167786,-3.70918174129627,
-11.7130906511012)) ;
#62494=CARTESIAN_POINT('Ctrl Pts',(-29.3434450791279,-3.5009827220688,-11.6968665288286)) ;
#62495=CARTESIAN_POINT('Ctrl Pts',(-29.3301979493458,-3.43176847082764,
-11.6914699477771)) ;
#62496=CARTESIAN_POINT('Ctrl Pts',(-29.3037800722982,-3.29372405730508,
-11.6806995282709)) ;
#62497=CARTESIAN_POINT('Ctrl Pts',(-29.2906093242772,-3.22489389502025,
-11.6753256917129)) ;
#62498=CARTESIAN_POINT('Ctrl Pts',(-29.2643474292101,-3.08763090555886,
-11.6646000791918)) ;
#62499=CARTESIAN_POINT('Ctrl Pts',(-29.2512562762877,-3.01919807839586,
-11.6592483179852)) ;
#62500=CARTESIAN_POINT('Ctrl Pts',(-29.2251571269213,-2.88274300686055,
-11.6485653291006)) ;
#62501=CARTESIAN_POINT('Ctrl Pts',(-29.2121491159705,-2.81472076241558,
-11.6432341377916)) ;
#62502=CARTESIAN_POINT('Ctrl Pts',(-29.1873494579291,-2.68500550281629,
-11.6330527085583)) ;
#62503=CARTESIAN_POINT('Ctrl Pts',(-29.1749249851303,-2.62000539423729,
-11.6279442950313)) ;
#62504=CARTESIAN_POINT('Ctrl Pts',(-29.1558514471759,-2.52018397795713,
-11.6200820076069)) ;
#62505=CARTESIAN_POINT('Ctrl Pts',(-29.1494208071324,-2.48652329705063,
-11.6174279403858)) ;
#62506=CARTESIAN_POINT('Ctrl Pts',(-29.1364886563188,-2.41881510426724,
-11.6120816988483)) ;
#62507=CARTESIAN_POINT('Ctrl Pts',(-29.1299871389251,-2.38476759234486,
-11.6093895411308)) ;
#62508=CARTESIAN_POINT('Ctrl Pts',(-29.1169882561854,-2.31667265961795,
-11.6039948557154)) ;
#62509=CARTESIAN_POINT('Ctrl Pts',(-29.1104908770745,-2.28262525247775,
-11.601292370194)) ;
#62510=CARTESIAN_POINT('Ctrl Pts',(-29.1008046681233,-2.23184440710932,
-11.5972504691071)) ;
#62511=CARTESIAN_POINT('Ctrl Pts',(-29.0975859151669,-2.2149658362827,-11.5959051230648)) ;
#62512=CARTESIAN_POINT('Ctrl Pts',(-29.0911779605547,-2.18135381364955,
-11.5932212870612)) ;
#62513=CARTESIAN_POINT('Ctrl Pts',(-29.0879887580595,-2.16462036183514,
-11.5918827992034)) ;
#62514=CARTESIAN_POINT('Ctrl Pts',(-29.0816496517882,-2.13134694250851,
-11.5892152191654)) ;
#62515=CARTESIAN_POINT('Ctrl Pts',(-29.0784997421844,-2.1148069788354,-11.5878861437555)) ;
#62516=CARTESIAN_POINT('Ctrl Pts',(-29.0722492732017,-2.08196890476153,
-11.5852391670673)) ;
#62517=CARTESIAN_POINT('Ctrl Pts',(-29.0691486959344,-2.06567079415595,
-11.5839213105721)) ;
#62518=CARTESIAN_POINT('Ctrl Pts',(-29.0645428686228,-2.04144129464998,
-11.5819530171012)) ;
#62519=CARTESIAN_POINT('Ctrl Pts',(-29.06301510888,-2.03340107341341,-11.5812983108891)) ;
#62520=CARTESIAN_POINT('Ctrl Pts',(-29.0599760971031,-2.0173992346742,-11.5799913540353)) ;
#62521=CARTESIAN_POINT('Ctrl Pts',(-29.0584648447653,-2.00943761716704,
-11.5793391041545)) ;
#62522=CARTESIAN_POINT('Ctrl Pts',(-29.0554605286591,-1.99359903538093,
-11.5780362189339)) ;
#62523=CARTESIAN_POINT('Ctrl Pts',(-29.0539674543051,-1.98572207127651,
-11.5773856102598)) ;
#62524=CARTESIAN_POINT('Ctrl Pts',(-29.0517430535571,-1.9739746568621,-11.5764095052018)) ;
#62525=CARTESIAN_POINT('Ctrl Pts',(-29.0510041261744,-1.97007019078463,
-11.576084093849)) ;
#62526=CARTESIAN_POINT('Ctrl Pts',(-29.049531697887,-1.96228469444513,-11.5754327366215)) ;
#62527=CARTESIAN_POINT('Ctrl Pts',(-29.0487981963141,-1.9584036641698,-11.5751067924166)) ;
#62528=CARTESIAN_POINT('Ctrl Pts',(-29.047336173308,-1.95066098584731,-11.5744532264714)) ;
#62529=CARTESIAN_POINT('Ctrl Pts',(-29.0465687995152,-1.9465936188602,-11.574108257814)) ;
#62530=CARTESIAN_POINT('Ctrl Pts',(-29.0449998503682,-1.93826543065782,
-11.573396148711)) ;
#62531=CARTESIAN_POINT('Ctrl Pts',(-29.0441982478596,-1.93400460876335,
-11.5730290760388)) ;
#62532=CARTESIAN_POINT('Ctrl Pts',(-29.0429989312286,-1.92761363883573,
-11.5724708657062)) ;
#62533=CARTESIAN_POINT('Ctrl Pts',(-29.0425996822224,-1.92548337261373,
-11.5722835143255)) ;
#62534=CARTESIAN_POINT('Ctrl Pts',(-29.0418072269102,-1.92124716215557,
-11.5719072252163)) ;
#62535=CARTESIAN_POINT('Ctrl Pts',(-29.0414140072555,-1.91914121746326,
-11.5717183207359)) ;
#62536=CARTESIAN_POINT('Ctrl Pts',(-29.0408327391823,-1.91601870741386,
-11.5714338036012)) ;
#62537=CARTESIAN_POINT('Ctrl Pts',(-29.0406404150943,-1.91498394237568,
-11.5713387606467)) ;
#62538=CARTESIAN_POINT('Ctrl Pts',(-29.0402593970723,-1.91292958018145,
-11.5711480324161)) ;
#62539=CARTESIAN_POINT('Ctrl Pts',(-29.0400707021886,-1.91190998298244,
-11.5710523495)) ;
#62540=CARTESIAN_POINT('Ctrl Pts',(-29.0396978711363,-1.90988898839402,
-11.5708597036493)) ;
#62541=CARTESIAN_POINT('Ctrl Pts',(-29.0395137207856,-1.90888759283122,
-11.5707627773289)) ;
#62542=CARTESIAN_POINT('Ctrl Pts',(-29.039241934621,-1.90740143728902,-11.570615144439)) ;
#62543=CARTESIAN_POINT('Ctrl Pts',(-29.0391520828946,-1.90690870891373,
-11.5705655503985)) ;
#62544=CARTESIAN_POINT('Ctrl Pts',(-29.0389741671165,-1.90592895356708,
-11.5704650588555)) ;
#62545=CARTESIAN_POINT('Ctrl Pts',(-29.0388860939987,-1.90544192594556,
-11.570414183744)) ;
#62546=CARTESIAN_POINT('Ctrl Pts',(-29.0387544860605,-1.90470902409679,
-11.5703352939177)) ;
#62547=CARTESIAN_POINT('Ctrl Pts',(-29.0387077267517,-1.90444770690439,
-11.5703067497927)) ;
#62548=CARTESIAN_POINT('Ctrl Pts',(-29.0386125894249,-1.90391283046634,
-11.5702468890951)) ;
#62549=CARTESIAN_POINT('Ctrl Pts',(-29.0385642095461,-1.90363927104027,
-11.5702155770922)) ;
#62550=CARTESIAN_POINT('Ctrl Pts',(-29.0384685129407,-1.90309246508965,
-11.5701504594772)) ;
#62551=CARTESIAN_POINT('Ctrl Pts',(-29.0384211681404,-1.90281925738603,
-11.5701167460003)) ;
#62552=CARTESIAN_POINT('Ctrl Pts',(-29.0382419508967,-1.90163369622182,
-11.5699046133964)) ;
#62553=CARTESIAN_POINT('Ctrl Pts',(-29.0382345917593,-1.90158501392234,
-11.5698959026666)) ;
#62554=CARTESIAN_POINT('Ctrl Pts',(-29.0382272326218,-1.90153633162286,
-11.5698871919368)) ;
#62555=CARTESIAN_POINT('',(-33.9221570292818,-15.0366437072151,1.85404835843691)) ;
#62556=CARTESIAN_POINT('',(-33.9237617799843,-15.0366437072151,1.82445047330719)) ;
#62557=CARTESIAN_POINT('Origin',(1.36393928288322,-21.6462763158694,-0.0739506391351341)) ;
#62558=CARTESIAN_POINT('',(-31.2124507867215,-1.90153624137795,1.69228991844779)) ;
#62559=CARTESIAN_POINT('Ctrl Pts',(-31.2124508052405,-1.90153633118548,
1.69228991969808)) ;
#62560=CARTESIAN_POINT('Ctrl Pts',(-31.2124604755823,-1.90158488686852,
1.69229690755422)) ;
#62561=CARTESIAN_POINT('Ctrl Pts',(-31.2126251204459,-1.90241158399461,
1.69241588107553)) ;
#62562=CARTESIAN_POINT('Ctrl Pts',(-31.212705653647,-1.90280827544799,1.69244478471387)) ;
#62563=CARTESIAN_POINT('Ctrl Pts',(-31.212760800475,-1.90307912005623,1.69246152971225)) ;
#62564=CARTESIAN_POINT('Ctrl Pts',(-31.2128713104034,-1.90362119954096,
1.69249252053007)) ;
#62565=CARTESIAN_POINT('Ctrl Pts',(-31.212926670686,-1.90389239564668,1.69250667032759)) ;
#62566=CARTESIAN_POINT('Ctrl Pts',(-31.2130349930476,-1.90442265270014,
1.69253287984097)) ;
#62567=CARTESIAN_POINT('Ctrl Pts',(-31.2130879554519,-1.90468171384137,
1.69254493429805)) ;
#62568=CARTESIAN_POINT('Ctrl Pts',(-31.2132365506487,-1.90540822375625,
1.69257749175176)) ;
#62569=CARTESIAN_POINT('Ctrl Pts',(-31.2133353803456,-1.90589098158148,
1.69259746904939)) ;
#62570=CARTESIAN_POINT('Ctrl Pts',(-31.2135343040682,-1.90686214761777,
1.69263567313032)) ;
#62571=CARTESIAN_POINT('Ctrl Pts',(-31.2136343995226,-1.90735055647549,
1.69265387603227)) ;
#62572=CARTESIAN_POINT('Ctrl Pts',(-31.2139364182847,-1.90882368383591,
1.69270669141445)) ;
#62573=CARTESIAN_POINT('Ctrl Pts',(-31.2141400714612,-1.90981630111776,
1.69273954957263)) ;
#62574=CARTESIAN_POINT('Ctrl Pts',(-31.214551252172,-1.91181958001539,1.69280268642164)) ;
#62575=CARTESIAN_POINT('Ctrl Pts',(-31.2147587814458,-1.91283023980567,
1.69283292605898)) ;
#62576=CARTESIAN_POINT('Ctrl Pts',(-31.2151770468983,-1.91486659457386,
1.69289164979098)) ;
#62577=CARTESIAN_POINT('Ctrl Pts',(-31.2153877832248,-1.91589228959527,
1.69292013132606)) ;
#62578=CARTESIAN_POINT('Ctrl Pts',(-31.2160238344561,-1.91898743046011,
1.69300363239075)) ;
#62579=CARTESIAN_POINT('Ctrl Pts',(-31.2164529859612,-1.9210749168561,1.69305675441327)) ;
#62580=CARTESIAN_POINT('Ctrl Pts',(-31.2173164601078,-1.92527399853841,
1.69315965094693)) ;
#62581=CARTESIAN_POINT('Ctrl Pts',(-31.2177507847721,-1.92738559428033,
1.69320938988903)) ;
#62582=CARTESIAN_POINT('Ctrl Pts',(-31.2190540178841,-1.93372055273571,
1.69335448116223)) ;
#62583=CARTESIAN_POINT('Ctrl Pts',(-31.2199231709228,-1.93794403361868,
1.69344577335652)) ;
#62584=CARTESIAN_POINT('Ctrl Pts',(-31.2216223264932,-1.94619923707333,
1.69361846627839)) ;
#62585=CARTESIAN_POINT('Ctrl Pts',(-31.2224523331006,-1.95023096032421,
1.69369979442831)) ;
#62586=CARTESIAN_POINT('Ctrl Pts',(-31.2240324597143,-1.95790548170987,
1.69385126692986)) ;
#62587=CARTESIAN_POINT('Ctrl Pts',(-31.2248245652681,-1.96175219457053,
1.69392541697728)) ;
#62588=CARTESIAN_POINT('Ctrl Pts',(-31.2264137045607,-1.96946884894499,
1.69407149049838)) ;
#62589=CARTESIAN_POINT('Ctrl Pts',(-31.2272107384001,-1.97333879047229,
1.69414341216294)) ;
#62590=CARTESIAN_POINT('Ctrl Pts',(-31.2296089557526,-1.9849823305565,1.69435663218088)) ;
#62591=CARTESIAN_POINT('Ctrl Pts',(-31.2312172524603,-1.99278964420127,
1.69449543265273)) ;
#62592=CARTESIAN_POINT('Ctrl Pts',(-31.2344514391384,-2.00848817671179,
1.69476882808044)) ;
#62593=CARTESIAN_POINT('Ctrl Pts',(-31.2360773306178,-2.01637939540296,
1.69490339453578)) ;
#62594=CARTESIAN_POINT('Ctrl Pts',(-31.2393453968111,-2.03223974160802,
1.69516959452397)) ;
#62595=CARTESIAN_POINT('Ctrl Pts',(-31.2409875715695,-2.0402088691264,1.69530122724354)) ;
#62596=CARTESIAN_POINT('Ctrl Pts',(-31.2459365970091,-2.06422412530555,
1.69569289120128)) ;
#62597=CARTESIAN_POINT('Ctrl Pts',(-31.2492659426475,-2.08037812413097,
1.6959497894869)) ;
#62598=CARTESIAN_POINT('Ctrl Pts',(-31.2559745203328,-2.1129258364843,1.69645852467273)) ;
#62599=CARTESIAN_POINT('Ctrl Pts',(-31.259353755023,-2.12931955021719,1.69671031360131)) ;
#62600=CARTESIAN_POINT('Ctrl Pts',(-31.2661521113103,-2.16229875913384,
1.69721028915278)) ;
#62601=CARTESIAN_POINT('Ctrl Pts',(-31.2695712330708,-2.17888425047914,
1.69745845810773)) ;
#62602=CARTESIAN_POINT('Ctrl Pts',(-31.2764394040602,-2.21219906927763,
1.6979518677282)) ;
#62603=CARTESIAN_POINT('Ctrl Pts',(-31.2798884534117,-2.22892839673869,
1.69819710615362)) ;
#62604=CARTESIAN_POINT('Ctrl Pts',(-31.2902655897258,-2.27926022911249,
1.69892882490881)) ;
#62605=CARTESIAN_POINT('Ctrl Pts',(-31.2972236609703,-2.31300658372593,
1.6994113809596)) ;
#62606=CARTESIAN_POINT('Ctrl Pts',(-31.3111404252094,-2.38049941138889,
1.70036547765197)) ;
#62607=CARTESIAN_POINT('Ctrl Pts',(-31.3180991177708,-2.41424587077575,
1.70083697412828)) ;
#62608=CARTESIAN_POINT('Ctrl Pts',(-31.331937876193,-2.48135537953355,1.70176659803113)) ;
#62609=CARTESIAN_POINT('Ctrl Pts',(-31.3388179430265,-2.51471842895004,
1.70222470769067)) ;
#62610=CARTESIAN_POINT('Ctrl Pts',(-31.3592214051958,-2.61365721390697,
1.70357425000709)) ;
#62611=CARTESIAN_POINT('Ctrl Pts',(-31.3725080558855,-2.67808258579967,
1.70444101111377)) ;
#62612=CARTESIAN_POINT('Ctrl Pts',(-31.399011920675,-2.80659298322074,1.70615604528631)) ;
#62613=CARTESIAN_POINT('Ctrl Pts',(-31.412905198914,-2.87395567908353,1.70704657648263)) ;
#62614=CARTESIAN_POINT('Ctrl Pts',(-31.4407762858584,-3.00908767251738,
1.7088206467358)) ;
#62615=CARTESIAN_POINT('Ctrl Pts',(-31.4547540966814,-3.07685697016082,
1.7097041470078)) ;
#62616=CARTESIAN_POINT('Ctrl Pts',(-31.4827913969966,-3.21278904806916,
1.71146667551889)) ;
#62617=CARTESIAN_POINT('Ctrl Pts',(-31.4968508873389,-3.28095182832054,
1.7123456880226)) ;
#62618=CARTESIAN_POINT('Ctrl Pts',(-31.5250487430717,-3.41765775368248,
1.71410087761831)) ;
#62619=CARTESIAN_POINT('Ctrl Pts',(-31.5391871085716,-3.48620089879647,
1.71497705268787)) ;
#62620=CARTESIAN_POINT('Ctrl Pts',(-31.5817163544578,-3.69238120612899,
1.71760300564436)) ;
#62621=CARTESIAN_POINT('Ctrl Pts',(-31.6102213782223,-3.83056923968495,
1.71935031957216)) ;
#62622=CARTESIAN_POINT('Ctrl Pts',(-31.6675138017569,-4.10830936619815,
1.72284371778677)) ;
#62623=CARTESIAN_POINT('Ctrl Pts',(-31.6963012047564,-4.24786145923466,
1.72458974280963)) ;
#62624=CARTESIAN_POINT('Ctrl Pts',(-31.7541365245639,-4.52822477707554,
1.72808325781092)) ;
#62625=CARTESIAN_POINT('Ctrl Pts',(-31.7831844426181,-4.66903600097254,
1.72983072133869)) ;
#62626=CARTESIAN_POINT('Ctrl Pts',(-31.8415190007151,-4.95181265093575,
1.73332850241756)) ;
#62627=CARTESIAN_POINT('Ctrl Pts',(-31.8708056414777,-5.09377807701703,
1.7350788067485)) ;
#62628=CARTESIAN_POINT('Ctrl Pts',(-31.9295958955513,-5.3787582045011,1.73858288735192)) ;
#62629=CARTESIAN_POINT('Ctrl Pts',(-31.9590995092129,-5.52177290590162,
1.74033665714628)) ;
#62630=CARTESIAN_POINT('Ctrl Pts',(-32.0183019863142,-5.80874665766087,
1.74384779656397)) ;
#62631=CARTESIAN_POINT('Ctrl Pts',(-32.0480008498168,-5.95270570802092,
1.74560516501718)) ;
#62632=CARTESIAN_POINT('Ctrl Pts',(-32.1373577569072,-6.38584199350258,
1.75088238301387)) ;
#62633=CARTESIAN_POINT('Ctrl Pts',(-32.1972761119937,-6.67627835833736,
1.75440742104842)) ;
#62634=CARTESIAN_POINT('Ctrl Pts',(-32.3176334772365,-7.25966935591344,
1.76146731493516)) ;
#62635=CARTESIAN_POINT('Ctrl Pts',(-32.3780724894743,-7.55262398868834,
1.76500213252553)) ;
#62636=CARTESIAN_POINT('Ctrl Pts',(-32.4992977674486,-8.14021210947855,
1.77207558219639)) ;
#62637=CARTESIAN_POINT('Ctrl Pts',(-32.5600840342126,-8.43484559749056,
1.77561419531164)) ;
#62638=CARTESIAN_POINT('Ctrl Pts',(-32.6818304790745,-9.02495201690094,
1.78268814011636)) ;
#62639=CARTESIAN_POINT('Ctrl Pts',(-32.7427906576548,-9.32042494830625,
1.7862234629264)) ;
#62640=CARTESIAN_POINT('Ctrl Pts',(-32.9256721036102,-10.2068437906719,
1.79681282728755)) ;
#62641=CARTESIAN_POINT('Ctrl Pts',(-33.0475942695293,-10.7977897343697,
1.80385042107764)) ;
#62642=CARTESIAN_POINT('Ctrl Pts',(-33.2900548260716,-11.9729664049461,
1.81781450787256)) ;
#62643=CARTESIAN_POINT('Ctrl Pts',(-33.4105932208701,-12.5571971318763,
1.82474092404302)) ;
#62644=CARTESIAN_POINT('Ctrl Pts',(-33.6489002671063,-13.7122280571188,
1.83841163542805)) ;
#62645=CARTESIAN_POINT('Ctrl Pts',(-33.766668920533,-14.2830282554284,1.84515589394605)) ;
#62646=CARTESIAN_POINT('Ctrl Pts',(-33.8956533090018,-14.9081862857511,
1.85253287884652)) ;
#62647=CARTESIAN_POINT('Ctrl Pts',(-33.9089194116541,-14.9724840414645,
1.85329148954973)) ;
#62648=CARTESIAN_POINT('Ctrl Pts',(-33.9221570292297,-15.0366437072146,
1.85404835938948)) ;
#62649=CARTESIAN_POINT('Ctrl Pts',(-33.9237617800355,-15.0366437072146,
1.82445047235329)) ;
#62650=CARTESIAN_POINT('Ctrl Pts',(-33.910519929938,-14.972484041565,1.82377166717211)) ;
#62651=CARTESIAN_POINT('Ctrl Pts',(-33.897249573524,-14.9081862859525,1.82309151287087)) ;
#62652=CARTESIAN_POINT('Ctrl Pts',(-33.7682237047426,-14.2830282558342,
1.81647958809875)) ;
#62653=CARTESIAN_POINT('Ctrl Pts',(-33.6504162336189,-13.7122280576294,
1.81045128027728)) ;
#62654=CARTESIAN_POINT('Ctrl Pts',(-33.4120280896458,-12.557197132599,1.7982763294461)) ;
#62655=CARTESIAN_POINT('Ctrl Pts',(-33.2914474187869,-11.9729664057762,
1.79212964973725)) ;
#62656=CARTESIAN_POINT('Ctrl Pts',(-33.0488983931026,-10.7977897354156,
1.77979728107933)) ;
#62657=CARTESIAN_POINT('Ctrl Pts',(-32.9269300424333,-10.2068437918263,
1.77361151529792)) ;
#62658=CARTESIAN_POINT('Ctrl Pts',(-32.7439757437029,-9.3204249496235,1.76436584192825)) ;
#62659=CARTESIAN_POINT('Ctrl Pts',(-32.6829906806809,-9.02495201827243,
1.76128948584647)) ;
#62660=CARTESIAN_POINT('Ctrl Pts',(-32.5611930907488,-8.43484559897041,
1.75515885676957)) ;
#62661=CARTESIAN_POINT('Ctrl Pts',(-32.5003805643192,-8.14021211101255,
1.75210457489359)) ;
#62662=CARTESIAN_POINT('Ctrl Pts',(-32.3791011397054,-7.55262399033026,
1.74602980163758)) ;
#62663=CARTESIAN_POINT('Ctrl Pts',(-32.31863424255,-7.25966935760917,1.74300929129468)) ;
#62664=CARTESIAN_POINT('Ctrl Pts',(-32.1982191085639,-6.67627836014022,
1.73701487959174)) ;
#62665=CARTESIAN_POINT('Ctrl Pts',(-32.1382708738013,-6.38584199535877,
1.7340409399602)) ;
#62666=CARTESIAN_POINT('Ctrl Pts',(-32.0488672131155,-5.95270570995667,
1.729626041596)) ;
#62667=CARTESIAN_POINT('Ctrl Pts',(-32.0191524406759,-5.80874665962307,
1.72816209632065)) ;
#62668=CARTESIAN_POINT('Ctrl Pts',(-31.9599173900955,-5.52177290791652,
1.72525173957642)) ;
#62669=CARTESIAN_POINT('Ctrl Pts',(-31.9303971120183,-5.37875820654228,
1.72380532694195)) ;
#62670=CARTESIAN_POINT('Ctrl Pts',(-31.8715726311884,-5.09377807911053,
1.7209325219118)) ;
#62671=CARTESIAN_POINT('Ctrl Pts',(-31.8422684287877,-4.95181265305536,
1.71950612303628)) ;
#62672=CARTESIAN_POINT('Ctrl Pts',(-31.7838976537235,-4.66903600314406,
1.71667632481136)) ;
#62673=CARTESIAN_POINT('Ctrl Pts',(-31.7548310817732,-4.52822477927292,
1.71527291224978)) ;
#62674=CARTESIAN_POINT('Ctrl Pts',(-31.6969570796863,-4.24786146148353,
1.71249285010884)) ;
#62675=CARTESIAN_POINT('Ctrl Pts',(-31.6681496511704,-4.10830936847265,
1.71111617410036)) ;
#62676=CARTESIAN_POINT('Ctrl Pts',(-31.610815375502,-3.83056924201046,1.70839469326928)) ;
#62677=CARTESIAN_POINT('Ctrl Pts',(-31.5822885315467,-3.6923812084799,1.70704982917742)) ;
#62678=CARTESIAN_POINT('Ctrl Pts',(-31.5397246784737,-3.48620090118523,
1.70506216836613)) ;
#62679=CARTESIAN_POINT('Ctrl Pts',(-31.5255744614924,-3.41765775608383,
1.70440458105773)) ;
#62680=CARTESIAN_POINT('Ctrl Pts',(-31.497352133427,-3.28095183074698,1.70310075717327)) ;
#62681=CARTESIAN_POINT('Ctrl Pts',(-31.4832800224533,-3.21278905050812,
1.70245451856732)) ;
#62682=CARTESIAN_POINT('Ctrl Pts',(-31.4552165151465,-3.07685697262473,
1.70117534967155)) ;
#62683=CARTESIAN_POINT('Ctrl Pts',(-31.4412251196694,-3.00908767499377,
1.70054240364651)) ;
#62684=CARTESIAN_POINT('Ctrl Pts',(-31.4133256035017,-2.87395568158474,
1.69929267966148)) ;
#62685=CARTESIAN_POINT('Ctrl Pts',(-31.3994174848983,-2.80659298573433,
1.69867586292556)) ;
#62686=CARTESIAN_POINT('Ctrl Pts',(-31.3728835590771,-2.67808258825811,
1.69751527164832)) ;
#62687=CARTESIAN_POINT('Ctrl Pts',(-31.3595810819296,-2.61365721629451,
1.6969404121094)) ;
#62688=CARTESIAN_POINT('Ctrl Pts',(-31.3391513145168,-2.51471843122878,
1.69607604104657)) ;
#62689=CARTESIAN_POINT('Ctrl Pts',(-31.3322620485548,-2.48135538177564,
1.69578759918871)) ;
#62690=CARTESIAN_POINT('Ctrl Pts',(-31.3184039034883,-2.41424587294404,
1.69521554061912)) ;
#62691=CARTESIAN_POINT('Ctrl Pts',(-31.3114350253373,-2.38049941352006,
1.69493190614639)) ;
#62692=CARTESIAN_POINT('Ctrl Pts',(-31.2974966857533,-2.31300658578286,
1.69437574299248)) ;
#62693=CARTESIAN_POINT('Ctrl Pts',(-31.2905272295257,-2.27926023113236,
1.69410317045799)) ;
#62694=CARTESIAN_POINT('Ctrl Pts',(-31.2801318117043,-2.2289283987032,1.69370863405332)) ;
#62695=CARTESIAN_POINT('Ctrl Pts',(-31.276676465886,-2.21219907122377,1.69357952705449)) ;
#62696=CARTESIAN_POINT('Ctrl Pts',(-31.2697952094378,-2.17888425238866,
1.69332746438019)) ;
#62697=CARTESIAN_POINT('Ctrl Pts',(-31.2663692989285,-2.16229876102506,
1.69320450646045)) ;
#62698=CARTESIAN_POINT('Ctrl Pts',(-31.2595567380237,-2.12931955207216,
1.69296651952424)) ;
#62699=CARTESIAN_POINT('Ctrl Pts',(-31.2561700893765,-2.11292583832124,
1.69285147291781)) ;
#62700=CARTESIAN_POINT('Ctrl Pts',(-31.2494458337047,-2.08037812593213,
1.69263190104062)) ;
#62701=CARTESIAN_POINT('Ctrl Pts',(-31.246108229238,-2.06422412708902,1.69252732781365)) ;
#62702=CARTESIAN_POINT('Ctrl Pts',(-31.2411458688696,-2.04020887088343,
1.69238161204554)) ;
#62703=CARTESIAN_POINT('Ctrl Pts',(-31.2394990886085,-2.0322397433562,1.69233492279027)) ;
#62704=CARTESIAN_POINT('Ctrl Pts',(-31.2362213986742,-2.01637939713371,
1.69224622219386)) ;
#62705=CARTESIAN_POINT('Ctrl Pts',(-31.234590489045,-2.00848817843392,1.69220421003294)) ;
#62706=CARTESIAN_POINT('Ctrl Pts',(-31.2313457020589,-1.99278964590612,
1.6921263257159)) ;
#62707=CARTESIAN_POINT('Ctrl Pts',(-31.2297318262819,-1.98498233225289,
1.69209042508881)) ;
#62708=CARTESIAN_POINT('Ctrl Pts',(-31.2273246142407,-1.97333879215588,
1.6920431022953)) ;
#62709=CARTESIAN_POINT('Ctrl Pts',(-31.2265244765495,-1.96946885062398,
1.69202842779028)) ;
#62710=CARTESIAN_POINT('Ctrl Pts',(-31.2249288595321,-1.96175219624107,
1.69200182884216)) ;
#62711=CARTESIAN_POINT('Ctrl Pts',(-31.2241333803023,-1.95790548337636,
1.69198990257096)) ;
#62712=CARTESIAN_POINT('Ctrl Pts',(-31.2225461393377,-1.95023096168779,
1.69196964539493)) ;
#62713=CARTESIAN_POINT('Ctrl Pts',(-31.2217122050812,-1.94619923812308,
1.69196075727152)) ;
#62714=CARTESIAN_POINT('Ctrl Pts',(-31.2200043385117,-1.93794403402632,
1.6919487268236)) ;
#62715=CARTESIAN_POINT('Ctrl Pts',(-31.2191304099921,-1.93372055281537,
1.69194551194037)) ;
#62716=CARTESIAN_POINT('Ctrl Pts',(-31.2178191292608,-1.92738559386717,
1.6919488483903)) ;
#62717=CARTESIAN_POINT('Ctrl Pts',(-31.2173819728692,-1.92527399796036,
1.69195133695555)) ;
#62718=CARTESIAN_POINT('Ctrl Pts',(-31.2165124353052,-1.92107491595138,
1.69196027232917)) ;
#62719=CARTESIAN_POINT('Ctrl Pts',(-31.2160800559731,-1.91898742939227,
1.69196668344944)) ;
#62720=CARTESIAN_POINT('Ctrl Pts',(-31.2154387051982,-1.91589228828676,
1.69198092579564)) ;
#62721=CARTESIAN_POINT('Ctrl Pts',(-31.2152261248002,-1.91486659318724,
1.69198645586048)) ;
#62722=CARTESIAN_POINT('Ctrl Pts',(-31.2148039620526,-1.91283023826074,
1.69199961290183)) ;
#62723=CARTESIAN_POINT('Ctrl Pts',(-31.2145943798285,-1.91181957839179,
1.6920072374057)) ;
#62724=CARTESIAN_POINT('Ctrl Pts',(-31.2141787831505,-1.90981629933822,
1.69202554768463)) ;
#62725=CARTESIAN_POINT('Ctrl Pts',(-31.2139727711923,-1.90882368197796,
1.69203619439398)) ;
#62726=CARTESIAN_POINT('Ctrl Pts',(-31.2136668125056,-1.90735055450323,
1.69205604620806)) ;
#62727=CARTESIAN_POINT('Ctrl Pts',(-31.2135653357217,-1.90686214561062,
1.69206332029631)) ;
#62728=CARTESIAN_POINT('Ctrl Pts',(-31.2133634474945,-1.90589097949916,
1.69207979299927)) ;
#62729=CARTESIAN_POINT('Ctrl Pts',(-31.2132630372143,-1.90540822163286,
1.69208896768993)) ;
#62730=CARTESIAN_POINT('Ctrl Pts',(-31.2131117930028,-1.90468171168872,
1.6921052683243)) ;
#62731=CARTESIAN_POINT('Ctrl Pts',(-31.2130578377534,-1.9044226505553,1.69211152584795)) ;
#62732=CARTESIAN_POINT('Ctrl Pts',(-31.2129473166385,-1.90389239352006,
1.69212587002178)) ;
#62733=CARTESIAN_POINT('Ctrl Pts',(-31.2128907510105,-1.90362119743088,
1.69213395157609)) ;
#62734=CARTESIAN_POINT('Ctrl Pts',(-31.212777538204,-1.90307911796257,1.69215281247392)) ;
#62735=CARTESIAN_POINT('Ctrl Pts',(-31.2127209042014,-1.90280827335977,
1.69216349681887)) ;
#62736=CARTESIAN_POINT('Ctrl Pts',(-31.2124714797407,-1.90163369094096,
1.69228024276397)) ;
#62737=CARTESIAN_POINT('Ctrl Pts',(-31.2124611424906,-1.90158501106322,
1.69228508123103)) ;
#62738=CARTESIAN_POINT('Ctrl Pts',(-31.2124508052405,-1.90153633118548,
1.69228991969808)) ;
#62739=CARTESIAN_POINT('',(-30.0084212027444,-15.0366437072153,15.9262327545894)) ;
#62740=CARTESIAN_POINT('',(-30.0223054639863,-15.0366437072153,15.9000442597427)) ;
#62741=CARTESIAN_POINT('Origin',(1.20682669964218,-21.6462763158694,-0.639819022420596)) ;
#62742=CARTESIAN_POINT('',(-27.6170790284909,-1.90153624302636,14.6416486516027)) ;
#62743=CARTESIAN_POINT('Ctrl Pts',(-27.617079045072,-1.9015363344823,14.6416486606773)) ;
#62744=CARTESIAN_POINT('Ctrl Pts',(-27.6170849036807,-1.90158489434699,
14.6416590345023)) ;
#62745=CARTESIAN_POINT('Ctrl Pts',(-27.6171857446532,-1.90242072828766,
14.641837593382)) ;
#62746=CARTESIAN_POINT('Ctrl Pts',(-27.6172474058173,-1.90282163229673,
14.6418981646337)) ;
#62747=CARTESIAN_POINT('Ctrl Pts',(-27.617290915074,-1.90309535072763,14.6419368604685)) ;
#62748=CARTESIAN_POINT('Ctrl Pts',(-27.6173791857354,-1.90364317822138,
14.642012062681)) ;
#62749=CARTESIAN_POINT('Ctrl Pts',(-27.6174239850381,-1.90391724844841,
14.6420484804412)) ;
#62750=CARTESIAN_POINT('Ctrl Pts',(-27.6175122659352,-1.90445312328647,
14.6421183899042)) ;
#62751=CARTESIAN_POINT('Ctrl Pts',(-27.6175557499699,-1.90471492808516,
14.6421518770866)) ;
#62752=CARTESIAN_POINT('Ctrl Pts',(-27.6176782981338,-1.90544921113751,
14.6422446881917)) ;
#62753=CARTESIAN_POINT('Ctrl Pts',(-27.6177605162274,-1.90593716129565,
14.6423048892218)) ;
#62754=CARTESIAN_POINT('Ctrl Pts',(-27.6179268505096,-1.9069187724624,14.6424242306893)) ;
#62755=CARTESIAN_POINT('Ctrl Pts',(-27.6180109781392,-1.90741243412097,
14.6424833498336)) ;
#62756=CARTESIAN_POINT('Ctrl Pts',(-27.6182657067604,-1.90890140455296,
14.6426598058831)) ;
#62757=CARTESIAN_POINT('Ctrl Pts',(-27.6184386345518,-1.90990469676427,
14.6427762762253)) ;
#62758=CARTESIAN_POINT('Ctrl Pts',(-27.6187891319733,-1.91192951903267,
14.6430085079058)) ;
#62759=CARTESIAN_POINT('Ctrl Pts',(-27.6189667196568,-1.912951047262,14.6431242343853)) ;
#62760=CARTESIAN_POINT('Ctrl Pts',(-27.6193255770666,-1.91500930016886,
14.6433554468608)) ;
#62761=CARTESIAN_POINT('Ctrl Pts',(-27.6195068479783,-1.91604602488884,
14.6434709306392)) ;
#62762=CARTESIAN_POINT('Ctrl Pts',(-27.6200550047461,-1.91917444836702,
14.6438172397545)) ;
#62763=CARTESIAN_POINT('Ctrl Pts',(-27.6204262100252,-1.9212843811877,14.6440479625586)) ;
#62764=CARTESIAN_POINT('Ctrl Pts',(-27.6211747756337,-1.92552861374704,
14.6445085490547)) ;
#62765=CARTESIAN_POINT('Ctrl Pts',(-27.621552152844,-1.92766291394181,14.6447383811071)) ;
#62766=CARTESIAN_POINT('Ctrl Pts',(-27.6226862623404,-1.93406598579517,
14.645424222177)) ;
#62767=CARTESIAN_POINT('Ctrl Pts',(-27.6234449317066,-1.9383348756467,14.6458766296199)) ;
#62768=CARTESIAN_POINT('Ctrl Pts',(-27.6249305344079,-1.94667883304679,
14.6467557917244)) ;
#62769=CARTESIAN_POINT('Ctrl Pts',(-27.6256575020925,-1.95075390127448,
14.6471824818955)) ;
#62770=CARTESIAN_POINT('Ctrl Pts',(-27.6270429511285,-1.95851130668981,
14.6479917704875)) ;
#62771=CARTESIAN_POINT('Ctrl Pts',(-27.6277382519714,-1.96239975264163,
14.6483958539826)) ;
#62772=CARTESIAN_POINT('Ctrl Pts',(-27.6291343137498,-1.97020012509417,
14.649204081629)) ;
#62773=CARTESIAN_POINT('Ctrl Pts',(-27.6298350755349,-1.97411205160832,
14.6496082241834)) ;
#62774=CARTESIAN_POINT('Ctrl Pts',(-27.6319449619627,-1.98588191230647,
14.6508213511136)) ;
#62775=CARTESIAN_POINT('Ctrl Pts',(-27.633361665421,-1.99377392723216,14.6516310765538)) ;
#62776=CARTESIAN_POINT('Ctrl Pts',(-27.6362129847788,-2.00964277237373,
14.6532541610047)) ;
#62777=CARTESIAN_POINT('Ctrl Pts',(-27.6376476141085,-2.01761960241516,
14.6540674946062)) ;
#62778=CARTESIAN_POINT('Ctrl Pts',(-27.6405330465774,-2.03365201638472,
14.6556984005312)) ;
#62779=CARTESIAN_POINT('Ctrl Pts',(-27.6419838501062,-2.04170760031738,
14.656515972121)) ;
#62780=CARTESIAN_POINT('Ctrl Pts',(-27.6463582652038,-2.06598339582831,
14.6589752914403)) ;
#62781=CARTESIAN_POINT('Ctrl Pts',(-27.6493038328558,-2.08231264765909,
14.660623733535)) ;
#62782=CARTESIAN_POINT('Ctrl Pts',(-27.6552428635702,-2.11521346622004,
14.6639371853392)) ;
#62783=CARTESIAN_POINT('Ctrl Pts',(-27.6582363492858,-2.13178503315512,
14.6656021524101)) ;
#62784=CARTESIAN_POINT('Ctrl Pts',(-27.6642614280585,-2.16512202863509,
14.6689457391089)) ;
#62785=CARTESIAN_POINT('Ctrl Pts',(-27.6672930287337,-2.1818874533408,14.6706243426738)) ;
#62786=CARTESIAN_POINT('Ctrl Pts',(-27.6733849174245,-2.21556369897872,
14.6739915877195)) ;
#62787=CARTESIAN_POINT('Ctrl Pts',(-27.6764452065005,-2.23247451991884,
14.6756802272031)) ;
#62788=CARTESIAN_POINT('Ctrl Pts',(-27.6856552674657,-2.28335239284995,
14.6807552345299)) ;
#62789=CARTESIAN_POINT('Ctrl Pts',(-27.6918341989637,-2.31746485466174,
14.6841507554935)) ;
#62790=CARTESIAN_POINT('Ctrl Pts',(-27.704197279302,-2.38568989673412,14.6909320087283)) ;
#62791=CARTESIAN_POINT('Ctrl Pts',(-27.7103814464014,-2.41980246332999,
14.69431770053)) ;
#62792=CARTESIAN_POINT('Ctrl Pts',(-27.7226832977556,-2.48764002620402,
14.7010434902844)) ;
#62793=CARTESIAN_POINT('Ctrl Pts',(-27.7288009903973,-2.5213650225277,14.7043835724376)) ;
#62794=CARTESIAN_POINT('Ctrl Pts',(-27.7469473693318,-2.62137716728801,
14.7142806543689)) ;
#62795=CARTESIAN_POINT('Ctrl Pts',(-27.7587693022826,-2.68650147115872,
14.7207145919794)) ;
#62796=CARTESIAN_POINT('Ctrl Pts',(-27.7823702026186,-2.81647723714774,
14.733543132641)) ;
#62797=CARTESIAN_POINT('Ctrl Pts',(-27.7947515322033,-2.88464215120766,
14.7402634360118)) ;
#62798=CARTESIAN_POINT('Ctrl Pts',(-27.8195947676845,-3.02138342310543,
14.753733586337)) ;
#62799=CARTESIAN_POINT('Ctrl Pts',(-27.8320566919655,-3.08995978101598,
14.7604833986468)) ;
#62800=CARTESIAN_POINT('Ctrl Pts',(-27.857057432086,-3.22751066532536,14.7740136600503)) ;
#62801=CARTESIAN_POINT('Ctrl Pts',(-27.8695962553744,-3.29648519171056,
14.7807940950877)) ;
#62802=CARTESIAN_POINT('Ctrl Pts',(-27.8947475269405,-3.43481913900766,
14.7943859069561)) ;
#62803=CARTESIAN_POINT('Ctrl Pts',(-27.9073599761762,-3.50417855992295,
14.8011972819796)) ;
#62804=CARTESIAN_POINT('Ctrl Pts',(-27.9453032278437,-3.71281425486547,
14.8216775868742)) ;
#62805=CARTESIAN_POINT('Ctrl Pts',(-27.9707398829137,-3.85264796043412,
14.8353927930809)) ;
#62806=CARTESIAN_POINT('Ctrl Pts',(-28.0218730017821,-4.13369567528339,
14.8629421363133)) ;
#62807=CARTESIAN_POINT('Ctrl Pts',(-28.047569493618,-4.27490968464348,14.8767762204895)) ;
#62808=CARTESIAN_POINT('Ctrl Pts',(-28.0992010723601,-4.5586118298814,14.9045564880959)) ;
#62809=CARTESIAN_POINT('Ctrl Pts',(-28.125136171597,-4.70109996484956,14.9185026478667)) ;
#62810=CARTESIAN_POINT('Ctrl Pts',(-28.1772243679445,-4.98724418213772,
14.946499071459)) ;
#62811=CARTESIAN_POINT('Ctrl Pts',(-28.2033774713037,-5.13090026447277,
14.9605493235009)) ;
#62812=CARTESIAN_POINT('Ctrl Pts',(-28.255881443487,-5.41927420008585,14.9887452495852)) ;
#62813=CARTESIAN_POINT('Ctrl Pts',(-28.2822323153732,-5.56399205336157,
15.0028909178505)) ;
#62814=CARTESIAN_POINT('Ctrl Pts',(-28.3351118237506,-5.85438335493212,
15.0312685577992)) ;
#62815=CARTESIAN_POINT('Ctrl Pts',(-28.361640460793,-6.00005680322832,15.0455005284421)) ;
#62816=CARTESIAN_POINT('Ctrl Pts',(-28.4414632438374,-6.43835127726969,
15.0883117910004)) ;
#62817=CARTESIAN_POINT('Ctrl Pts',(-28.4949942250459,-6.73224642747102,
15.1170065007152)) ;
#62818=CARTESIAN_POINT('Ctrl Pts',(-28.602530121798,-7.32258498527443,15.17462626168)) ;
#62819=CARTESIAN_POINT('Ctrl Pts',(-28.6565350554198,-7.61902839291019,
15.2035512788457)) ;
#62820=CARTESIAN_POINT('Ctrl Pts',(-28.7648621679001,-8.21361405642605,
15.2615524472652)) ;
#62821=CARTESIAN_POINT('Ctrl Pts',(-28.819184355712,-8.5117563123029,15.2906285816295)) ;
#62822=CARTESIAN_POINT('Ctrl Pts',(-28.9279898034778,-9.10889026395786,
15.3488518040726)) ;
#62823=CARTESIAN_POINT('Ctrl Pts',(-28.9824730676241,-9.40788195974288,
15.3779988842453)) ;
#62824=CARTESIAN_POINT('Ctrl Pts',(-29.145930698864,-10.3048570952872,15.4654253604834)) ;
#62825=CARTESIAN_POINT('Ctrl Pts',(-29.2549128280494,-10.9028405678066,
15.5236901301374)) ;
#62826=CARTESIAN_POINT('Ctrl Pts',(-29.4716533430531,-12.0920123241697,
15.6395298961061)) ;
#62827=CARTESIAN_POINT('Ctrl Pts',(-29.5794117651472,-12.683200608065,15.6971048240178)) ;
#62828=CARTESIAN_POINT('Ctrl Pts',(-29.7949448266547,-13.8656062560031,
15.8122369207257)) ;
#62829=CARTESIAN_POINT('Ctrl Pts',(-29.9026613337374,-14.4565031969479,
15.8697623699)) ;
#62830=CARTESIAN_POINT('Ctrl Pts',(-30.00842120271,-15.0366437072152,15.9262327546544)) ;
#62831=CARTESIAN_POINT('Ctrl Pts',(-30.0223054640204,-15.0366437072153,
15.9000442596783)) ;
#62832=CARTESIAN_POINT('Ctrl Pts',(-30.0198892745065,-15.0234311858862,
15.8987723880774)) ;
#62833=CARTESIAN_POINT('Ctrl Pts',(-30.017472062495,-15.0102130853408,15.8974999835935)) ;
#62834=CARTESIAN_POINT('Ctrl Pts',(-29.9112916285261,-14.4295845144665,
15.8416075390388)) ;
#62835=CARTESIAN_POINT('Ctrl Pts',(-29.8056613310825,-13.8519867028476,
15.7860145804868)) ;
#62836=CARTESIAN_POINT('Ctrl Pts',(-29.5919042492259,-12.6832006072026,
15.6735414990053)) ;
#62837=CARTESIAN_POINT('Ctrl Pts',(-29.4837774821379,-12.0920123231792,
15.6166613433989)) ;
#62838=CARTESIAN_POINT('Ctrl Pts',(-29.2662662086894,-10.9028405665586,
15.5022753819669)) ;
#62839=CARTESIAN_POINT('Ctrl Pts',(-29.1568817385884,-10.3048570939097,
15.4447695077282)) ;
#62840=CARTESIAN_POINT('Ctrl Pts',(-28.9927894976363,-9.40788195817102,
15.3585400323025)) ;
#62841=CARTESIAN_POINT('Ctrl Pts',(-28.9380894769186,-9.10889026232123,
15.3298017983665)) ;
#62842=CARTESIAN_POINT('Ctrl Pts',(-28.8288385463144,-8.51175631053695,
15.2724188456376)) ;
#62843=CARTESIAN_POINT('Ctrl Pts',(-28.7742876406181,-8.21361405459552,
15.2437741189394)) ;
#62844=CARTESIAN_POINT('Ctrl Pts',(-28.6654889372615,-7.61902839095087,
15.186662465218)) ;
#62845=CARTESIAN_POINT('Ctrl Pts',(-28.6112411485568,-7.32258498325092,
15.158195521304)) ;
#62846=CARTESIAN_POINT('Ctrl Pts',(-28.503202151987,-6.73224642531964,15.1015247072058)) ;
#62847=CARTESIAN_POINT('Ctrl Pts',(-28.4494109621869,-6.43835127505464,
15.0733208029325)) ;
#62848=CARTESIAN_POINT('Ctrl Pts',(-28.369181037787,-6.00005680091835,15.0312774903949)) ;
#62849=CARTESIAN_POINT('Ctrl Pts',(-28.3425138642898,-5.85438335259064,
15.0173068272121)) ;
#62850=CARTESIAN_POINT('Ctrl Pts',(-28.289350707775,-5.56399205095715,14.9894642043788)) ;
#62851=CARTESIAN_POINT('Ctrl Pts',(-28.2628547253106,-5.41927419765009,
14.9755922436859)) ;
#62852=CARTESIAN_POINT('Ctrl Pts',(-28.2100527174169,-5.13090026197456,
14.9479584725587)) ;
#62853=CARTESIAN_POINT('Ctrl Pts',(-28.1837466950485,-4.9872441796084,14.9341966563524)) ;
#62854=CARTESIAN_POINT('Ctrl Pts',(-28.1313431411937,-4.70109996225825,
14.9067950600924)) ;
#62855=CARTESIAN_POINT('Ctrl Pts',(-28.1052456159516,-4.55861182725925,
14.8931552682541)) ;
#62856=CARTESIAN_POINT('Ctrl Pts',(-28.0532772199223,-4.27490968195984,
14.866010305419)) ;
#62857=CARTESIAN_POINT('Ctrl Pts',(-28.0274063617978,-4.13369567256921,
14.8525051109391)) ;
#62858=CARTESIAN_POINT('Ctrl Pts',(-27.975908828566,-3.85264795765906,14.825643126086)) ;
#62859=CARTESIAN_POINT('Ctrl Pts',(-27.9502821814665,-3.71281425206012,
14.8122862828497)) ;
#62860=CARTESIAN_POINT('Ctrl Pts',(-27.9120375963644,-3.50417855707243,
14.7923743530876)) ;
#62861=CARTESIAN_POINT('Ctrl Pts',(-27.8993219528192,-3.43481913614209,
14.7857576231735)) ;
#62862=CARTESIAN_POINT('Ctrl Pts',(-27.8739575913849,-3.29648518881505,
14.7725677414212)) ;
#62863=CARTESIAN_POINT('Ctrl Pts',(-27.8613088744532,-3.22751066241491,
14.7659945877775)) ;
#62864=CARTESIAN_POINT('Ctrl Pts',(-27.8360799339616,-3.08995977807574,
14.7528947579221)) ;
#62865=CARTESIAN_POINT('Ctrl Pts',(-27.823499717855,-3.02138342015034,14.7463680676582)) ;
#62866=CARTESIAN_POINT('Ctrl Pts',(-27.7984089202078,-2.88464214822294,
14.7333648691004)) ;
#62867=CARTESIAN_POINT('Ctrl Pts',(-27.7858983570277,-2.81647723414827,
14.7268883261428)) ;
#62868=CARTESIAN_POINT('Ctrl Pts',(-27.7620357951218,-2.68650146849467,
14.7145533317067)) ;
#62869=CARTESIAN_POINT('Ctrl Pts',(-27.7500761799523,-2.62137716499163,
14.7083790904721)) ;
#62870=CARTESIAN_POINT('Ctrl Pts',(-27.7317009610864,-2.52136502079594,
14.6989136466899)) ;
#62871=CARTESIAN_POINT('Ctrl Pts',(-27.7255032418861,-2.48764002466267,
14.695724510723)) ;
#62872=CARTESIAN_POINT('Ctrl Pts',(-27.7130327399128,-2.41980246217161,
14.6893168299511)) ;
#62873=CARTESIAN_POINT('Ctrl Pts',(-27.7067599655119,-2.3856898957683,14.6860982693346)) ;
#62874=CARTESIAN_POINT('Ctrl Pts',(-27.6942091961128,-2.31746485408108,
14.6796710353937)) ;
#62875=CARTESIAN_POINT('Ctrl Pts',(-27.687931224366,-2.28335239246188,14.6764623242415)) ;
#62876=CARTESIAN_POINT('Ctrl Pts',(-27.6785621296037,-2.232474519818,14.6716872866043)) ;
#62877=CARTESIAN_POINT('Ctrl Pts',(-27.675447066653,-2.21556369897336,14.6701019616504)) ;
#62878=CARTESIAN_POINT('Ctrl Pts',(-27.6692413458727,-2.18188745352556,
14.6669494267863)) ;
#62879=CARTESIAN_POINT('Ctrl Pts',(-27.6661506891041,-2.16512202891445,
14.6653822148722)) ;
#62880=CARTESIAN_POINT('Ctrl Pts',(-27.6600020429387,-2.13178503362268,
14.6622717010839)) ;
#62881=CARTESIAN_POINT('Ctrl Pts',(-27.6569440625584,-2.11521346678123,
14.660728383897)) ;
#62882=CARTESIAN_POINT('Ctrl Pts',(-27.6508686477712,-2.08231264840602,
14.6576721798256)) ;
#62883=CARTESIAN_POINT('Ctrl Pts',(-27.6478512359416,-2.06598339666736,
14.6561592502659)) ;
#62884=CARTESIAN_POINT('Ctrl Pts',(-27.6433608192526,-2.04170760129347,
14.6539187332194)) ;
#62885=CARTESIAN_POINT('Ctrl Pts',(-27.641869952078,-2.03365201740627,14.6531767297022)) ;
#62886=CARTESIAN_POINT('Ctrl Pts',(-27.6389008018245,-2.01761960352721,
14.6517037323102)) ;
#62887=CARTESIAN_POINT('Ctrl Pts',(-27.637422519138,-2.00964277353076,14.6509727376943)) ;
#62888=CARTESIAN_POINT('Ctrl Pts',(-27.6344789864692,-1.99377392847877,
14.6495235860387)) ;
#62889=CARTESIAN_POINT('Ctrl Pts',(-27.6330137499688,-1.98588191359784,
14.6488054036467)) ;
#62890=CARTESIAN_POINT('Ctrl Pts',(-27.6308256171952,-1.97411205296613,
14.6477398650107)) ;
#62891=CARTESIAN_POINT('Ctrl Pts',(-27.6300978544014,-1.97020012647409,
14.647386651771)) ;
#62892=CARTESIAN_POINT('Ctrl Pts',(-27.628645441466,-1.96239975406557,14.6466847137016)) ;
#62893=CARTESIAN_POINT('Ctrl Pts',(-27.6279207921727,-1.95851130813563,
14.6463359872661)) ;
#62894=CARTESIAN_POINT('Ctrl Pts',(-27.6264734567956,-1.95075390253628,
14.6456434286151)) ;
#62895=CARTESIAN_POINT('Ctrl Pts',(-27.6257123251301,-1.9466788340925,14.6452811784527)) ;
#62896=CARTESIAN_POINT('Ctrl Pts',(-27.6241509512269,-1.93833487624977,
14.644544935801)) ;
#62897=CARTESIAN_POINT('Ctrl Pts',(-27.6233507430922,-1.93406598617168,
14.6441708786873)) ;
#62898=CARTESIAN_POINT('Ctrl Pts',(-27.6221466323401,-1.92766291397871,
14.6436170738425)) ;
#62899=CARTESIAN_POINT('Ctrl Pts',(-27.6217446236619,-1.92552861367038,
14.6434337016171)) ;
#62900=CARTESIAN_POINT('Ctrl Pts',(-27.6209433159066,-1.92128438088597,
14.643072597264)) ;
#62901=CARTESIAN_POINT('Ctrl Pts',(-27.6205440335406,-1.91917444795388,
14.6428948334146)) ;
#62902=CARTESIAN_POINT('Ctrl Pts',(-27.6199497787747,-1.91604602430983,
14.6426354742745)) ;
#62903=CARTESIAN_POINT('Ctrl Pts',(-27.6197524672339,-1.91500929953434,
14.6425502463075)) ;
#62904=CARTESIAN_POINT('Ctrl Pts',(-27.6193597090545,-1.91295104651823,
14.6423829774186)) ;
#62905=CARTESIAN_POINT('Ctrl Pts',(-27.619164263621,-1.91192951823391,14.6423009342046)) ;
#62906=CARTESIAN_POINT('Ctrl Pts',(-27.6187753533729,-1.9099046958582,14.6421411567538)) ;
#62907=CARTESIAN_POINT('Ctrl Pts',(-27.6185819073017,-1.90890140359366,
14.6420633879694)) ;
#62908=CARTESIAN_POINT('Ctrl Pts',(-27.6182929061471,-1.90741243308273,
14.6419515767408)) ;
#62909=CARTESIAN_POINT('Ctrl Pts',(-27.6181967625174,-1.9069187713992,14.6419151221661)) ;
#62910=CARTESIAN_POINT('Ctrl Pts',(-27.6180046402354,-1.90593716018056,
14.6418444220033)) ;
#62911=CARTESIAN_POINT('Ctrl Pts',(-27.617908672781,-1.90544920999584,14.641810155007)) ;
#62912=CARTESIAN_POINT('Ctrl Pts',(-27.617763081606,-1.90471492694364,14.6417608076318)) ;
#62913=CARTESIAN_POINT('Ctrl Pts',(-27.6177109619107,-1.90445312217609,
14.6417436090468)) ;
#62914=CARTESIAN_POINT('Ctrl Pts',(-27.6176035565294,-1.90391724739378,
14.6417097722123)) ;
#62915=CARTESIAN_POINT('Ctrl Pts',(-27.6175482731852,-1.90364317719369,
14.6416931294639)) ;
#62916=CARTESIAN_POINT('Ctrl Pts',(-27.6174364927896,-1.90309534975757,
14.6416622713397)) ;
#62917=CARTESIAN_POINT('Ctrl Pts',(-27.617380047885,-1.90282163135034,14.6416479747356)) ;
#62918=CARTESIAN_POINT('Ctrl Pts',(-27.6171018470644,-1.90163370011507,
14.6416486087149)) ;
#62919=CARTESIAN_POINT('Ctrl Pts',(-27.6170904460682,-1.90158501729869,
14.6416486346961)) ;
#62920=CARTESIAN_POINT('Ctrl Pts',(-27.617079045072,-1.9015363344823,14.6416486606773)) ;
#62921=CARTESIAN_POINT('',(-20.5476539041775,-15.0366437072153,27.0544663940876)) ;
#62922=CARTESIAN_POINT('',(-20.5712511819771,-15.0366437072153,27.0365282098624)) ;
#62923=CARTESIAN_POINT('Origin',(0.826633213912537,-21.6462763158694,-1.08741739643853)) ;
#62924=CARTESIAN_POINT('',(-18.9167133915938,-1.90153624328746,24.8845109207828)) ;
#62925=CARTESIAN_POINT('Ctrl Pts',(-18.9167134028615,-1.9015363350045,24.8845109360263)) ;
#62926=CARTESIAN_POINT('Ctrl Pts',(-18.9167143685661,-1.90158489556102,
24.8845228078318)) ;
#62927=CARTESIAN_POINT('Ctrl Pts',(-18.9167310208152,-1.90242225567914,
24.8847275208156)) ;
#62928=CARTESIAN_POINT('Ctrl Pts',(-18.9167616201006,-1.90282386086443,
24.8848085131963)) ;
#62929=CARTESIAN_POINT('Ctrl Pts',(-18.9167849102915,-1.90309805764489,
24.8848619876481)) ;
#62930=CARTESIAN_POINT('Ctrl Pts',(-18.9168335480839,-1.90364684188482,
24.8849674739658)) ;
#62931=CARTESIAN_POINT('Ctrl Pts',(-18.9168589674186,-1.90392139050459,
24.8850194212191)) ;
#62932=CARTESIAN_POINT('Ctrl Pts',(-18.9169098374949,-1.90445820041271,
24.8851201021622)) ;
#62933=CARTESIAN_POINT('Ctrl Pts',(-18.9169352923059,-1.90472046188661,
24.8851688328067)) ;
#62934=CARTESIAN_POINT('Ctrl Pts',(-18.9170076880584,-1.90545603941596,
24.8853047487709)) ;
#62935=CARTESIAN_POINT('Ctrl Pts',(-18.9170571270611,-1.9059448544838,24.8853940585281)) ;
#62936=CARTESIAN_POINT('Ctrl Pts',(-18.9171581757274,-1.90692820554584,
24.8855725130536)) ;
#62937=CARTESIAN_POINT('Ctrl Pts',(-18.9172098047175,-1.90742274218952,
24.885661643299)) ;
#62938=CARTESIAN_POINT('Ctrl Pts',(-18.9173672021873,-1.90891435167757,
24.8859292022212)) ;
#62939=CARTESIAN_POINT('Ctrl Pts',(-18.9174754494137,-1.90991942206317,
24.8861078226986)) ;
#62940=CARTESIAN_POINT('Ctrl Pts',(-18.9176964604024,-1.9119478329134,24.8864663730323)) ;
#62941=CARTESIAN_POINT('Ctrl Pts',(-18.9178092552605,-1.91297117155114,
24.8866462787757)) ;
#62942=CARTESIAN_POINT('Ctrl Pts',(-18.9180382923743,-1.91503307213536,
24.8870074214629)) ;
#62943=CARTESIAN_POINT('Ctrl Pts',(-18.9181545367088,-1.91607163412574,
24.8871886568378)) ;
#62944=CARTESIAN_POINT('Ctrl Pts',(-18.9185072774196,-1.91920560164744,
24.8877340621205)) ;
#62945=CARTESIAN_POINT('Ctrl Pts',(-18.9187477425563,-1.92131927347479,
24.888099956833)) ;
#62946=CARTESIAN_POINT('Ctrl Pts',(-18.9192346278442,-1.92557102703072,
24.8888335559801)) ;
#62947=CARTESIAN_POINT('Ctrl Pts',(-18.9194810765899,-1.92770910921484,
24.8892012387961)) ;
#62948=CARTESIAN_POINT('Ctrl Pts',(-18.9202237554663,-1.93412352704139,
24.8903017982988)) ;
#62949=CARTESIAN_POINT('Ctrl Pts',(-18.920723258853,-1.93839998088127,24.8910322174041)) ;
#62950=CARTESIAN_POINT('Ctrl Pts',(-18.9217041965976,-1.94675872244878,
24.8924563874319)) ;
#62951=CARTESIAN_POINT('Ctrl Pts',(-18.9221856892737,-1.95084101085567,
24.8931500941983)) ;
#62952=CARTESIAN_POINT('Ctrl Pts',(-18.9231049569439,-1.95861222293703,
24.8944686268492)) ;
#62953=CARTESIAN_POINT('Ctrl Pts',(-18.9235671715973,-1.96250762084814,
24.8951284731753)) ;
#62954=CARTESIAN_POINT('Ctrl Pts',(-18.9244965379162,-1.97032193918007,
24.8964505190558)) ;
#62955=CARTESIAN_POINT('Ctrl Pts',(-18.9249636910165,-1.97424085961422,
24.8971127175227)) ;
#62956=CARTESIAN_POINT('Ctrl Pts',(-18.9263717650827,-1.98603176298418,
24.8991031475054)) ;
#62957=CARTESIAN_POINT('Ctrl Pts',(-18.9273192629094,-1.99393788757247,
24.9004352423095)) ;
#62958=CARTESIAN_POINT('Ctrl Pts',(-18.9292290124779,-2.00983510364014,
24.9031102729783)) ;
#62959=CARTESIAN_POINT('Ctrl Pts',(-18.9301912870776,-2.01782619494491,
24.9044531914216)) ;
#62960=CARTESIAN_POINT('Ctrl Pts',(-18.9321287558131,-2.03388727221324,
24.9071496875273)) ;
#62961=CARTESIAN_POINT('Ctrl Pts',(-18.9331039506085,-2.04195725818132,
24.9085032646887)) ;
#62962=CARTESIAN_POINT('Ctrl Pts',(-18.9360467601344,-2.0662764547135,24.9125792593993)) ;
#62963=CARTESIAN_POINT('Ctrl Pts',(-18.9380315183021,-2.08263490044522,
24.9153170013827)) ;
#62964=CARTESIAN_POINT('Ctrl Pts',(-18.9420376064851,-2.11559453995239,
24.9208276995194)) ;
#62965=CARTESIAN_POINT('Ctrl Pts',(-18.944058974998,-2.13219573393279,24.9236006264605)) ;
#62966=CARTESIAN_POINT('Ctrl Pts',(-18.9481306122324,-2.16559233001946,
24.9291749257832)) ;
#62967=CARTESIAN_POINT('Ctrl Pts',(-18.950180894613,-2.18238772828634,24.9319762867846)) ;
#62968=CARTESIAN_POINT('Ctrl Pts',(-18.9543033162345,-2.21612418093343,
24.9376002047454)) ;
#62969=CARTESIAN_POINT('Ctrl Pts',(-18.9563754572838,-2.23306523532159,
24.9404227603317)) ;
#62970=CARTESIAN_POINT('Ctrl Pts',(-18.9626145961174,-2.28403406848378,
24.9489109737907)) ;
#62971=CARTESIAN_POINT('Ctrl Pts',(-18.9668042516112,-2.31820751696578,
24.95459722236)) ;
#62972=CARTESIAN_POINT('Ctrl Pts',(-18.975192415737,-2.38655453238059,24.965963020267)) ;
#62973=CARTESIAN_POINT('Ctrl Pts',(-18.97939095797,-2.42072808564842,24.9716425405143)) ;
#62974=CARTESIAN_POINT('Ctrl Pts',(-18.9877467683852,-2.48868692883717,
24.9829321668039)) ;
#62975=CARTESIAN_POINT('Ctrl Pts',(-18.991904050825,-2.52247221880362,24.9885422620198)) ;
#62976=CARTESIAN_POINT('Ctrl Pts',(-19.004239767148,-2.62266316540279,25.0051736273985)) ;
#62977=CARTESIAN_POINT('Ctrl Pts',(-19.0122819776285,-2.68790389838004,
25.0159960474464)) ;
#62978=CARTESIAN_POINT('Ctrl Pts',(-19.0283453367079,-2.81812392893152,
25.0375890319205)) ;
#62979=CARTESIAN_POINT('Ctrl Pts',(-19.036777160132,-2.88642263950378,25.0489091013579)) ;
#62980=CARTESIAN_POINT('Ctrl Pts',(-19.053701642929,-3.02343231200211,25.0716100109559)) ;
#62981=CARTESIAN_POINT('Ctrl Pts',(-19.0621943335895,-3.09214327400093,
25.0829908273511)) ;
#62982=CARTESIAN_POINT('Ctrl Pts',(-19.0792367415917,-3.22996414801061,
25.1058126736773)) ;
#62983=CARTESIAN_POINT('Ctrl Pts',(-19.087786471612,-3.29907406000788,25.1172536939666)) ;
#62984=CARTESIAN_POINT('Ctrl Pts',(-19.1049398605727,-3.43767953400148,
25.1401948503665)) ;
#62985=CARTESIAN_POINT('Ctrl Pts',(-19.1135435211405,-3.50717509600125,
25.1516949852397)) ;
#62986=CARTESIAN_POINT('Ctrl Pts',(-19.1394313727074,-3.71622030832927,
25.1862819436808)) ;
#62987=CARTESIAN_POINT('Ctrl Pts',(-19.1567923463698,-3.85632848433072,
25.2094553871857)) ;
#62988=CARTESIAN_POINT('Ctrl Pts',(-19.1917005046174,-4.13792784932362,
25.2560197389565)) ;
#62989=CARTESIAN_POINT('Ctrl Pts',(-19.2092477369008,-4.27941903839452,
25.2794106109836)) ;
#62990=CARTESIAN_POINT('Ctrl Pts',(-19.2445119983007,-4.56367804392642,
25.3263946806514)) ;
#62991=CARTESIAN_POINT('Ctrl Pts',(-19.2622290485708,-4.70644585947729,
25.3499878619754)) ;
#62992=CARTESIAN_POINT('Ctrl Pts',(-19.2978175811806,-4.99315173039635,
25.397360612901)) ;
#62993=CARTESIAN_POINT('Ctrl Pts',(-19.3156890741506,-5.13708978577956,
25.4211401744257)) ;
#62994=CARTESIAN_POINT('Ctrl Pts',(-19.3515717475988,-5.42602975154862,
25.4688692776673)) ;
#62995=CARTESIAN_POINT('Ctrl Pts',(-19.3695829332874,-5.57103166193216,
25.4928188154226)) ;
#62996=CARTESIAN_POINT('Ctrl Pts',(-19.4057306414897,-5.8619929533723,25.5408711637485)) ;
#62997=CARTESIAN_POINT('Ctrl Pts',(-19.4238671649456,-6.00795233443024,
25.5649739736022)) ;
#62998=CARTESIAN_POINT('Ctrl Pts',(-19.4784435994783,-6.44710710762938,
25.6374869588184)) ;
#62999=CARTESIAN_POINT('Ctrl Pts',(-19.5150503131399,-6.74157912509782,
25.686101735427)) ;
#63000=CARTESIAN_POINT('Ctrl Pts',(-19.5885977926232,-7.33307641917909,
25.7837401535482)) ;
#63001=CARTESIAN_POINT('Ctrl Pts',(-19.6255385891958,-7.63010169582556,
25.8327637716931)) ;
#63002=CARTESIAN_POINT('Ctrl Pts',(-19.6996450744351,-8.22585443185994,
25.931081921884)) ;
#63003=CARTESIAN_POINT('Ctrl Pts',(-19.7368107783377,-8.52458189124458,
25.9803764423469)) ;
#63004=CARTESIAN_POINT('Ctrl Pts',(-19.8112587959478,-9.12288791716573,
26.0790977791134)) ;
#63005=CARTESIAN_POINT('Ctrl Pts',(-19.8485411167872,-9.4224664837092,26.1285245899967)) ;
#63006=CARTESIAN_POINT('Ctrl Pts',(-19.9604014044967,-10.3212022315355,
26.2767949056143)) ;
#63007=CARTESIAN_POINT('Ctrl Pts',(-20.0349925689043,-10.9203594455821,
26.3756283863428)) ;
#63008=CARTESIAN_POINT('Ctrl Pts',(-20.1833522435728,-12.1118653470381,
26.5721532765629)) ;
#63009=CARTESIAN_POINT('Ctrl Pts',(-20.2571208155407,-12.7042140344991,
26.6698446391582)) ;
#63010=CARTESIAN_POINT('Ctrl Pts',(-20.4035834685688,-13.8801354421801,
26.8637660032857)) ;
#63011=CARTESIAN_POINT('Ctrl Pts',(-20.4762636531478,-14.4635951118959,
26.9599772216812)) ;
#63012=CARTESIAN_POINT('Ctrl Pts',(-20.5476539041704,-15.0366437072153,
27.0544663940931)) ;
#63013=CARTESIAN_POINT('Ctrl Pts',(-20.5712511819829,-15.0366437072153,
27.036528209858)) ;
#63014=CARTESIAN_POINT('Ctrl Pts',(-20.5706612171046,-15.0319446557972,
27.0357568549883)) ;
#63015=CARTESIAN_POINT('Ctrl Pts',(-20.5700711638574,-15.0272449043228,
27.034985385566)) ;
#63016=CARTESIAN_POINT('Ctrl Pts',(-20.4981035141431,-14.4540257999816,
26.94089087751)) ;
#63017=CARTESIAN_POINT('Ctrl Pts',(-20.4254367995802,-13.8752942607969,
26.84589680268)) ;
#63018=CARTESIAN_POINT('Ctrl Pts',(-20.2783747273307,-12.7042140340873,
26.6536878353541)) ;
#63019=CARTESIAN_POINT('Ctrl Pts',(-20.2039793991207,-12.1118653465652,
26.5564729204515)) ;
#63020=CARTESIAN_POINT('Ctrl Pts',(-20.0543082598726,-10.9203594449863,
26.3609449796542)) ;
#63021=CARTESIAN_POINT('Ctrl Pts',(-19.9790325105307,-10.3212022308778,
26.262631906847)) ;
#63022=CARTESIAN_POINT('Ctrl Pts',(-19.8660924459332,-9.4224664829588,26.1151824162557)) ;
#63023=CARTESIAN_POINT('Ctrl Pts',(-19.8284413200228,-9.12288791638442,
26.0660359636907)) ;
#63024=CARTESIAN_POINT('Ctrl Pts',(-19.7532353311701,-8.5245818904015,25.9678908216667)) ;
#63025=CARTESIAN_POINT('Ctrl Pts',(-19.7156804753596,-8.22585443098604,
25.9188921267852)) ;
#63026=CARTESIAN_POINT('Ctrl Pts',(-19.6407716073414,-7.63010169489019,
25.8211839321094)) ;
#63027=CARTESIAN_POINT('Ctrl Pts',(-19.6034176103687,-7.33307641821306,
25.7724744207345)) ;
#63028=CARTESIAN_POINT('Ctrl Pts',(-19.5290141482999,-6.74157912407075,
25.675486703642)) ;
#63029=CARTESIAN_POINT('Ctrl Pts',(-19.4919647139464,-6.44710710657191,
25.6272084745458)) ;
#63030=CARTESIAN_POINT('Ctrl Pts',(-19.4366955704313,-6.00795233332746,
25.5552220729962)) ;
#63031=CARTESIAN_POINT('Ctrl Pts',(-19.4183233421613,-5.86199295225445,
25.5312984412799)) ;
#63032=CARTESIAN_POINT('Ctrl Pts',(-19.3816930386047,-5.57103166078429,
25.483612952397)) ;
#63033=CARTESIAN_POINT('Ctrl Pts',(-19.36343496426,-5.42602975038579,25.4598510945148)) ;
#63034=CARTESIAN_POINT('Ctrl Pts',(-19.3270452191944,-5.13708978458693,
25.4125074570877)) ;
#63035=CARTESIAN_POINT('Ctrl Pts',(-19.3089135536827,-4.99315172918884,
25.3889256735835)) ;
#63036=CARTESIAN_POINT('Ctrl Pts',(-19.2727884808785,-4.70644585824021,
25.3419607899022)) ;
#63037=CARTESIAN_POINT('Ctrl Pts',(-19.2547950842114,-4.5636780426746,25.3185776816439)) ;
#63038=CARTESIAN_POINT('Ctrl Pts',(-19.2189577734926,-4.27941903711337,
25.2720292327354)) ;
#63039=CARTESIAN_POINT('Ctrl Pts',(-19.2011138808186,-4.13792784802786,
25.2488638760705)) ;
#63040=CARTESIAN_POINT('Ctrl Pts',(-19.1655857215916,-3.8563284830059,25.2027708367835)) ;
#63041=CARTESIAN_POINT('Ctrl Pts',(-19.1479015027164,-3.71622030698998,
25.1798431178972)) ;
#63042=CARTESIAN_POINT('Ctrl Pts',(-19.1215009730845,-3.50717509464039,
25.1456458871834)) ;
#63043=CARTESIAN_POINT('Ctrl Pts',(-19.1127217412279,-3.43767953263345,
25.1342792181322)) ;
#63044=CARTESIAN_POINT('Ctrl Pts',(-19.0952058077974,-3.29907405862555,
25.1116136608695)) ;
#63045=CARTESIAN_POINT('Ctrl Pts',(-19.0864691078549,-3.22996414662115,
25.1003147714182)) ;
#63046=CARTESIAN_POINT('Ctrl Pts',(-19.0690384450932,-3.09214327259721,
25.0777880686832)) ;
#63047=CARTESIAN_POINT('Ctrl Pts',(-19.0603444949595,-3.02343231059132,
25.0665602457601)) ;
#63048=CARTESIAN_POINT('Ctrl Pts',(-19.0429988124476,-2.88642263807886,
25.0441795238575)) ;
#63049=CARTESIAN_POINT('Ctrl Pts',(-19.0343471113395,-2.81812392749956,
25.0330266010882)) ;
#63050=CARTESIAN_POINT('Ctrl Pts',(-19.0178385950926,-2.68790389707261,
25.0117720163273)) ;
#63051=CARTESIAN_POINT('Ctrl Pts',(-19.0095621715615,-2.62266316423356,
25.0011276404477)) ;
#63052=CARTESIAN_POINT('Ctrl Pts',(-18.9968371732943,-2.52247221784659,
24.9847921995644)) ;
#63053=CARTESIAN_POINT('Ctrl Pts',(-18.9925437569551,-2.48868692795171,
24.9792855906672)) ;
#63054=CARTESIAN_POINT('Ctrl Pts',(-18.9839010537239,-2.42072808490687,
24.9682140546636)) ;
#63055=CARTESIAN_POINT('Ctrl Pts',(-18.979551781078,-2.38655453171139,24.9626491167161)) ;
#63056=CARTESIAN_POINT('Ctrl Pts',(-18.9708443382193,-2.31820751644134,
24.9515260282295)) ;
#63057=CARTESIAN_POINT('Ctrl Pts',(-18.9664862050282,-2.28403406803175,
24.9459678530947)) ;
#63058=CARTESIAN_POINT('Ctrl Pts',(-18.9599765334731,-2.23306523497749,
24.9376852932921)) ;
#63059=CARTESIAN_POINT('Ctrl Pts',(-18.9578112165184,-2.2161241806252,24.934933568197)) ;
#63060=CARTESIAN_POINT('Ctrl Pts',(-18.9534951550256,-2.18238772804956,
24.929456851458)) ;
#63061=CARTESIAN_POINT('Ctrl Pts',(-18.9513444122986,-2.16559232981822,
24.9267318584357)) ;
#63062=CARTESIAN_POINT('Ctrl Pts',(-18.9470625745811,-2.1321957338023,24.9213173493843)) ;
#63063=CARTESIAN_POINT('Ctrl Pts',(-18.9449314942107,-2.11559453985707,
24.9186278232381)) ;
#63064=CARTESIAN_POINT('Ctrl Pts',(-18.9406934031869,-2.08263490041971,
24.913293489094)) ;
#63065=CARTESIAN_POINT('Ctrl Pts',(-18.938586430973,-2.06627645472267,24.9106486518222)) ;
#63066=CARTESIAN_POINT('Ctrl Pts',(-18.9354462912493,-2.04195725824198,
24.9067226636415)) ;
#63067=CARTESIAN_POINT('Ctrl Pts',(-18.9344029442324,-2.03388727229097,
24.9054208944563)) ;
#63068=CARTESIAN_POINT('Ctrl Pts',(-18.9323230632261,-2.01782619505665,
24.9028326573533)) ;
#63069=CARTESIAN_POINT('Ctrl Pts',(-18.931286529905,-2.00983510376875,24.9015461889268)) ;
#63070=CARTESIAN_POINT('Ctrl Pts',(-18.9292199162578,-1.99393788773474,
24.8989904032391)) ;
#63071=CARTESIAN_POINT('Ctrl Pts',(-18.928189858838,-1.98603176316325,24.8977210686105)) ;
#63072=CARTESIAN_POINT('Ctrl Pts',(-18.9266486797622,-1.97424085981823,
24.8958318224319)) ;
#63073=CARTESIAN_POINT('Ctrl Pts',(-18.9261355951483,-1.97032193939221,
24.895204540196)) ;
#63074=CARTESIAN_POINT('Ctrl Pts',(-18.9251103696795,-1.96250762107683,
24.8939553645511)) ;
#63075=CARTESIAN_POINT('Ctrl Pts',(-18.924598230256,-1.95861222317414,24.8933334700507)) ;
#63076=CARTESIAN_POINT('Ctrl Pts',(-18.9235736882859,-1.95084101111684,
24.8920949648484)) ;
#63077=CARTESIAN_POINT('Ctrl Pts',(-18.9230340800797,-1.94675872272648,
24.8914454363637)) ;
#63078=CARTESIAN_POINT('Ctrl Pts',(-18.9219242497106,-1.93839998119292,
24.8901192479705)) ;
#63079=CARTESIAN_POINT('Ctrl Pts',(-18.9213540857047,-1.93412352737036,
24.889442543676)) ;
#63080=CARTESIAN_POINT('Ctrl Pts',(-18.9204923292509,-1.92770910956992,
24.888432504601)) ;
#63081=CARTESIAN_POINT('Ctrl Pts',(-18.9202039804729,-1.9255710273949,24.8880966733639)) ;
#63082=CARTESIAN_POINT('Ctrl Pts',(-18.9196273766362,-1.92131927385614,
24.8874312764888)) ;
#63083=CARTESIAN_POINT('Ctrl Pts',(-18.9193391500849,-1.91920560203643,
24.8871016890618)) ;
#63084=CARTESIAN_POINT('Ctrl Pts',(-18.9189079929671,-1.91607163452743,
24.8866158943853)) ;
#63085=CARTESIAN_POINT('Ctrl Pts',(-18.9187644622541,-1.91503307254177,
24.8864554015773)) ;
#63086=CARTESIAN_POINT('Ctrl Pts',(-18.9184777571413,-1.91297117196593,
24.8861380969653)) ;
#63087=CARTESIAN_POINT('Ctrl Pts',(-18.9183345847531,-1.91194783333305,
24.8859812836212)) ;
#63088=CARTESIAN_POINT('Ctrl Pts',(-18.9180482302814,-1.90991942249111,
24.8856724061141)) ;
#63089=CARTESIAN_POINT('Ctrl Pts',(-18.9179050797004,-1.90891435211023,
24.8855203184782)) ;
#63090=CARTESIAN_POINT('Ctrl Pts',(-18.9176893815891,-1.90742274262821,
24.8852970785531)) ;
#63091=CARTESIAN_POINT('Ctrl Pts',(-18.9176173123751,-1.90692820598606,
24.8852234865624)) ;
#63092=CARTESIAN_POINT('Ctrl Pts',(-18.9174723958912,-1.90594485492843,
24.8850783794859)) ;
#63093=CARTESIAN_POINT('Ctrl Pts',(-18.9173995678447,-1.90545603986145,
24.8850068496178)) ;
#63094=CARTESIAN_POINT('Ctrl Pts',(-18.9172879738986,-1.90472046209792,
24.8849007312849)) ;
#63095=CARTESIAN_POINT('Ctrl Pts',(-18.9172478292892,-1.9044582003785,24.8848631674712)) ;
#63096=CARTESIAN_POINT('Ctrl Pts',(-18.9171644272708,-1.90392138996427,
24.8847872165361)) ;
#63097=CARTESIAN_POINT('Ctrl Pts',(-18.9171211738375,-1.9036468410861,24.884748826345)) ;
#63098=CARTESIAN_POINT('Ctrl Pts',(-18.9170325444076,-1.90309805632819,
24.8846737407453)) ;
#63099=CARTESIAN_POINT('Ctrl Pts',(-18.9169872500073,-1.90282385927809,
24.8846369933886)) ;
#63100=CARTESIAN_POINT('Ctrl Pts',(-18.9167341120365,-1.90163370160465,
24.8845204688771)) ;
#63101=CARTESIAN_POINT('Ctrl Pts',(-18.916723757449,-1.90158501830458,24.8845157024517)) ;
#63102=CARTESIAN_POINT('Ctrl Pts',(-18.9167134028615,-1.9015363350045,24.8845109360263)) ;
#63103=CARTESIAN_POINT('',(-7.28867002793326,-15.0366437072153,33.1817046285839)) ;
#63104=CARTESIAN_POINT('',(-7.31761838529145,-15.0366437072153,33.1753326132824)) ;
#63105=CARTESIAN_POINT('Origin',(0.293637272419048,-21.6462763158694,-1.3340075774398)) ;
#63106=CARTESIAN_POINT('',(-6.71960916186913,-1.90153624397926,30.5274922328533)) ;
#63107=CARTESIAN_POINT('Ctrl Pts',(-6.71960916572461,-1.9015363363881,30.527492251559)) ;
#63108=CARTESIAN_POINT('Ctrl Pts',(-6.71960503468368,-1.90158489401769,
30.5275034359727)) ;
#63109=CARTESIAN_POINT('Ctrl Pts',(-6.71953434398448,-1.90241581601747,
30.5276948245448)) ;
#63110=CARTESIAN_POINT('Ctrl Pts',(-6.71952806587547,-1.90281445409125,
30.5277805608094)) ;
#63111=CARTESIAN_POINT('Ctrl Pts',(-6.71952671045772,-1.90308662669026,
30.52783845261)) ;
#63112=CARTESIAN_POINT('Ctrl Pts',(-6.71952647178206,-1.9036313623249,30.5279537746666)) ;
#63113=CARTESIAN_POINT('Ctrl Pts',(-6.71952768038816,-1.90390388655798,
30.5280111764909)) ;
#63114=CARTESIAN_POINT('Ctrl Pts',(-6.71953147217083,-1.90443673958349,
30.5281230969409)) ;
#63115=CARTESIAN_POINT('Ctrl Pts',(-6.71953406034505,-1.90469706856311,
30.5281776145062)) ;
#63116=CARTESIAN_POINT('Ctrl Pts',(-6.71954254288055,-1.90542717101058,
30.5283302416739)) ;
#63117=CARTESIAN_POINT('Ctrl Pts',(-6.71954980436227,-1.90591232878685,
30.5284313057678)) ;
#63118=CARTESIAN_POINT('Ctrl Pts',(-6.71956635780412,-1.90688832266939,
30.5286341885841)) ;
#63119=CARTESIAN_POINT('Ctrl Pts',(-6.71957567329605,-1.90737915942458,
30.5287360022641)) ;
#63120=CARTESIAN_POINT('Ctrl Pts',(-6.71960581785518,-1.9088596096152,30.5290426396081)) ;
#63121=CARTESIAN_POINT('Ctrl Pts',(-6.71962880637323,-1.90985716095924,
30.5292486676527)) ;
#63122=CARTESIAN_POINT('Ctrl Pts',(-6.71967831619922,-1.91187039742389,
30.5296637833386)) ;
#63123=CARTESIAN_POINT('Ctrl Pts',(-6.71970487569611,-1.91288608071834,
30.5298728621872)) ;
#63124=CARTESIAN_POINT('Ctrl Pts',(-6.7197605522653,-1.91493255703098,30.5302936542332)) ;
#63125=CARTESIAN_POINT('Ctrl Pts',(-6.71978967180336,-1.91596335009186,
30.5305053668967)) ;
#63126=CARTESIAN_POINT('Ctrl Pts',(-6.71987994037281,-1.91907387452225,
30.5311437040075)) ;
#63127=CARTESIAN_POINT('Ctrl Pts',(-6.71994395324573,-1.92117173588608,
30.5315735344974)) ;
#63128=CARTESIAN_POINT('Ctrl Pts',(-6.72007660206596,-1.92539168676737,
30.5324373046928)) ;
#63129=CARTESIAN_POINT('Ctrl Pts',(-6.72014527296858,-1.92751377674115,
30.5328712368007)) ;
#63130=CARTESIAN_POINT('Ctrl Pts',(-6.72035534009416,-1.93388021790867,
30.5341721769161)) ;
#63131=CARTESIAN_POINT('Ctrl Pts',(-6.7205007238618,-1.93812468728337,30.5350383322065)) ;
#63132=CARTESIAN_POINT('Ctrl Pts',(-6.7207905249419,-1.94642091372353,30.5367300763717)) ;
#63133=CARTESIAN_POINT('Ctrl Pts',(-6.72093501344642,-1.95047267146818,
30.5375556497196)) ;
#63134=CARTESIAN_POINT('Ctrl Pts',(-6.7212133316577,-1.9581855017446,30.5391264711218)) ;
#63135=CARTESIAN_POINT('Ctrl Pts',(-6.72135457498788,-1.96205150310624,
30.5399134515561)) ;
#63136=CARTESIAN_POINT('Ctrl Pts',(-6.72164053693774,-1.9698068509058,30.5414915874222)) ;
#63137=CARTESIAN_POINT('Ctrl Pts',(-6.72178525732577,-1.97369619735714,
30.5422827424674)) ;
#63138=CARTESIAN_POINT('Ctrl Pts',(-6.72222378915863,-1.98539812121369,
30.5446624157223)) ;
#63139=CARTESIAN_POINT('Ctrl Pts',(-6.72252192512217,-1.99324458270728,
30.5462571521216)) ;
#63140=CARTESIAN_POINT('Ctrl Pts',(-6.72312698742384,-2.0090218315379,30.5494625338965)) ;
#63141=CARTESIAN_POINT('Ctrl Pts',(-6.7234339417142,-2.01695261870037,30.5510731730823)) ;
#63142=CARTESIAN_POINT('Ctrl Pts',(-6.72405505928695,-2.03289249242576,
30.5543094332857)) ;
#63143=CARTESIAN_POINT('Ctrl Pts',(-6.72436922337813,-2.0409015789932,30.5559350541256)) ;
#63144=CARTESIAN_POINT('Ctrl Pts',(-6.72532088665166,-2.06503725311967,
30.5608328391374)) ;
#63145=CARTESIAN_POINT('Ctrl Pts',(-6.72596745733348,-2.08127225164298,
30.564125946969)) ;
#63146=CARTESIAN_POINT('Ctrl Pts',(-6.7272788940997,-2.1139831651699,30.5707591149674)) ;
#63147=CARTESIAN_POINT('Ctrl Pts',(-6.72794380721284,-2.13045908037843,
30.5740991648255)) ;
#63148=CARTESIAN_POINT('Ctrl Pts',(-6.72928783210369,-2.16360365366924,
30.5808169247956)) ;
#63149=CARTESIAN_POINT('Ctrl Pts',(-6.72996696100518,-2.18027230791273,
30.5841946303259)) ;
#63150=CARTESIAN_POINT('Ctrl Pts',(-6.73133608992497,-2.21375417357443,
30.5909782376895)) ;
#63151=CARTESIAN_POINT('Ctrl Pts',(-6.73202609214606,-2.23056738500055,
30.5943841390392)) ;
#63152=CARTESIAN_POINT('Ctrl Pts',(-6.73410801808508,-2.28115159033711,
30.6046298116117)) ;
#63153=CARTESIAN_POINT('Ctrl Pts',(-6.73551179022772,-2.31506715501583,
30.6114975668916)) ;
#63154=CARTESIAN_POINT('Ctrl Pts',(-6.73833014157579,-2.38289840281523,
30.6252307237003)) ;
#63155=CARTESIAN_POINT('Ctrl Pts',(-6.73974476333159,-2.41681407227232,
30.6320961129715)) ;
#63156=CARTESIAN_POINT('Ctrl Pts',(-6.7425657903985,-2.48426007833226,30.645747161211)) ;
#63157=CARTESIAN_POINT('Ctrl Pts',(-6.74397221312697,-2.51779041498063,
30.652532816355)) ;
#63158=CARTESIAN_POINT('Ctrl Pts',(-6.74815180308299,-2.61722529311255,
30.672653870791)) ;
#63159=CARTESIAN_POINT('Ctrl Pts',(-6.75088517916712,-2.68197370242755,
30.6857533838662)) ;
#63160=CARTESIAN_POINT('Ctrl Pts',(-6.75635251277483,-2.81116116865304,
30.7118868210986)) ;
#63161=CARTESIAN_POINT('Ctrl Pts',(-6.75922734717377,-2.87889443305604,
30.7255868111386)) ;
#63162=CARTESIAN_POINT('Ctrl Pts',(-6.76500650404872,-3.01476980026688,
30.7530668132049)) ;
#63163=CARTESIAN_POINT('Ctrl Pts',(-6.76791086463308,-3.08291190314725,
30.7668468168585)) ;
#63164=CARTESIAN_POINT('Ctrl Pts',(-6.77374586998526,-3.21959175607126,
30.7944847600319)) ;
#63165=CARTESIAN_POINT('Ctrl Pts',(-6.77667653020986,-3.28812950610133,
30.8083426961463)) ;
#63166=CARTESIAN_POINT('Ctrl Pts',(-6.78256179851678,-3.42558746340932,
30.8361342274369)) ;
#63167=CARTESIAN_POINT('Ctrl Pts',(-6.78551640858651,-3.49450767069068,
30.8500678221752)) ;
#63168=CARTESIAN_POINT('Ctrl Pts',(-6.79441341605667,-3.70182219488036,
30.8919785127782)) ;
#63169=CARTESIAN_POINT('Ctrl Pts',(-6.80038888440015,-3.84077041348023,
30.9200655382932)) ;
#63170=CARTESIAN_POINT('Ctrl Pts',(-6.81241693001848,-4.12003841381346,
30.9765128478343)) ;
#63171=CARTESIAN_POINT('Ctrl Pts',(-6.81846956547146,-4.26035819562616,
31.0048731190712)) ;
#63172=CARTESIAN_POINT('Ctrl Pts',(-6.83064346250994,-4.54226381754215,
31.0618464617664)) ;
#63173=CARTESIAN_POINT('Ctrl Pts',(-6.83676475000264,-4.68384965673699,
31.0904595273298)) ;
#63174=CARTESIAN_POINT('Ctrl Pts',(-6.84906874931766,-4.96818188660624,
31.1479177180033)) ;
#63175=CARTESIAN_POINT('Ctrl Pts',(-6.85525147411698,-5.11092827729567,
31.1767628402602)) ;
#63176=CARTESIAN_POINT('Ctrl Pts',(-6.8676719030735,-5.39747610609673,31.2346642376376)) ;
#63177=CARTESIAN_POINT('Ctrl Pts',(-6.87390961359172,-5.54127754420606,
31.2637205113573)) ;
#63178=CARTESIAN_POINT('Ctrl Pts',(-6.8864340498454,-5.82982996427431,31.3220231992416)) ;
#63179=CARTESIAN_POINT('Ctrl Pts',(-6.89272077672559,-5.97458094623454,
31.3512696131538)) ;
#63180=CARTESIAN_POINT('Ctrl Pts',(-6.91164600392969,-6.41009995304015,
31.4392624435926)) ;
#63181=CARTESIAN_POINT('Ctrl Pts',(-6.92434947612127,-6.70213403411822,
31.4982624642693)) ;
#63182=CARTESIAN_POINT('Ctrl Pts',(-6.94988691163196,-7.28873431722379,
31.6167695952287)) ;
#63183=CARTESIAN_POINT('Ctrl Pts',(-6.96272091249833,-7.58330051928491,
31.6762766972538)) ;
#63184=CARTESIAN_POINT('Ctrl Pts',(-6.98847858561803,-8.17412101401313,
31.7956283738327)) ;
#63185=CARTESIAN_POINT('Ctrl Pts',(-7.00140227647572,-8.47037530667691,
31.8554729442908)) ;
#63186=CARTESIAN_POINT('Ctrl Pts',(-7.02729958170605,-9.0637279530796,31.9753297048947)) ;
#63187=CARTESIAN_POINT('Ctrl Pts',(-7.04027320479137,-9.36082630682544,
32.0353418931237)) ;
#63188=CARTESIAN_POINT('Ctrl Pts',(-7.07921035581026,-10.2521214162309,
32.2153748841193)) ;
#63189=CARTESIAN_POINT('Ctrl Pts',(-7.10519001132179,-10.8463182046384,
32.335392143864)) ;
#63190=CARTESIAN_POINT('Ctrl Pts',(-7.15688461897129,-12.0279596232458,
32.574056129412)) ;
#63191=CARTESIAN_POINT('Ctrl Pts',(-7.18259964647311,-12.6154042534972,
32.6927028386364)) ;
#63192=CARTESIAN_POINT('Ctrl Pts',(-7.23346099536655,-13.7767891025737,
32.9272638195374)) ;
#63193=CARTESIAN_POINT('Ctrl Pts',(-7.25860735275444,-14.3507293213961,
33.0431780832901)) ;
#63194=CARTESIAN_POINT('Ctrl Pts',(-7.28510452610227,-14.9552953856552,
33.1652756333742)) ;
#63195=CARTESIAN_POINT('Ctrl Pts',(-7.28688844246384,-14.995996643595,33.173495608376)) ;
#63196=CARTESIAN_POINT('Ctrl Pts',(-7.28867002731916,-15.036643707215,33.1817046287187)) ;
#63197=CARTESIAN_POINT('Ctrl Pts',(-7.31761838590095,-15.036643707215,33.175332613148)) ;
#63198=CARTESIAN_POINT('Ctrl Pts',(-7.31578843034696,-14.9959966435885,
33.1671342399998)) ;
#63199=CARTESIAN_POINT('Ctrl Pts',(-7.31395599106881,-14.9552953856421,
33.1589249456982)) ;
#63200=CARTESIAN_POINT('Ctrl Pts',(-7.28673674368188,-14.3507293213698,
33.0369863361262)) ;
#63201=CARTESIAN_POINT('Ctrl Pts',(-7.26088782347941,-13.7767891025407,
32.9212267181418)) ;
#63202=CARTESIAN_POINT('Ctrl Pts',(-7.20855873401436,-12.6154042534504,
32.6869888113683)) ;
#63203=CARTESIAN_POINT('Ctrl Pts',(-7.18207860074982,-12.0279596231921,
32.5685105146561)) ;
#63204=CARTESIAN_POINT('Ctrl Pts',(-7.12878294951492,-10.8463182045707,
32.3301989454477)) ;
#63205=CARTESIAN_POINT('Ctrl Pts',(-7.10196750690673,-10.2521214161561,
32.2103656563531)) ;
#63206=CARTESIAN_POINT('Ctrl Pts',(-7.06171201724267,-9.36082630674012,
32.030622853635)) ;
#63207=CARTESIAN_POINT('Ctrl Pts',(-7.04828809485541,-9.06372795299079,
31.9707097837769)) ;
#63208=CARTESIAN_POINT('Ctrl Pts',(-7.02146530499196,-8.47037530658109,
31.851056737744)) ;
#63209=CARTESIAN_POINT('Ctrl Pts',(-7.00806644622269,-8.17412101391379,
31.7913167596517)) ;
#63210=CARTESIAN_POINT('Ctrl Pts',(-6.98132900896538,-7.5833005191786,31.6721807454662)) ;
#63211=CARTESIAN_POINT('Ctrl Pts',(-6.96799044908368,-7.28873431711399,
31.6127847052781)) ;
#63212=CARTESIAN_POINT('Ctrl Pts',(-6.94140774508735,-6.70213403400147,
31.4945076553094)) ;
#63213=CARTESIAN_POINT('Ctrl Pts',(-6.92816363851496,-6.41009995291992,
31.4356266372581)) ;
#63214=CARTESIAN_POINT('Ctrl Pts',(-6.90839247902012,-5.9745809461092,31.347820010596)) ;
#63215=CARTESIAN_POINT('Ctrl Pts',(-6.90181790735092,-5.82982996414724,
31.3186369561127)) ;
#63216=CARTESIAN_POINT('Ctrl Pts',(-6.88870411460551,-5.54127754407557,
31.2604639954013)) ;
#63217=CARTESIAN_POINT('Ctrl Pts',(-6.88216489467994,-5.39747610596454,
31.2314740889205)) ;
#63218=CARTESIAN_POINT('Ctrl Pts',(-6.86912520497875,-5.11092827716008,
31.1737090011399)) ;
#63219=CARTESIAN_POINT('Ctrl Pts',(-6.86262474155889,-4.96818188646899,
31.1449338184418)) ;
#63220=CARTESIAN_POINT('Ctrl Pts',(-6.84966548084162,-4.68384965659638,
31.087619861709)) ;
#63221=CARTESIAN_POINT('Ctrl Pts',(-6.84320669651301,-4.54226381739987,
31.0590810848165)) ;
#63222=CARTESIAN_POINT('Ctrl Pts',(-6.83033294054922,-4.26035819548053,
31.0022617927193)) ;
#63223=CARTESIAN_POINT('Ctrl Pts',(-6.82391799490403,-4.12003841366617,
30.973981271986)) ;
#63224=CARTESIAN_POINT('Ctrl Pts',(-6.81113274336521,-3.84077041332965,
30.917700636071)) ;
#63225=CARTESIAN_POINT('Ctrl Pts',(-6.80476249564617,-3.70182219472812,
30.8897005080674)) ;
#63226=CARTESIAN_POINT('Ctrl Pts',(-6.7952393587118,-3.494507670536,30.8479276389809)) ;
#63227=CARTESIAN_POINT('Ctrl Pts',(-6.79207032560784,-3.42558746325382,
30.8340412423213)) ;
#63228=CARTESIAN_POINT('Ctrl Pts',(-6.78574228935676,-3.28812950594421,
30.8063471716248)) ;
#63229=CARTESIAN_POINT('Ctrl Pts',(-6.78258328820021,-3.21959175591332,
30.7925394971501)) ;
#63230=CARTESIAN_POINT('Ctrl Pts',(-6.77627412450336,-3.08291190298769,
30.7650059241204)) ;
#63231=CARTESIAN_POINT('Ctrl Pts',(-6.77312397742212,-3.01476980010652,
30.7512800221658)) ;
#63232=CARTESIAN_POINT('Ctrl Pts',(-6.76683044476954,-2.87889443289408,
30.7239132427695)) ;
#63233=CARTESIAN_POINT('Ctrl Pts',(-6.763687097298,-2.81116116849028,30.7102723569261)) ;
#63234=CARTESIAN_POINT('Ctrl Pts',(-6.75767596940615,-2.68197370215285,
30.6842586178435)) ;
#63235=CARTESIAN_POINT('Ctrl Pts',(-6.75465637157047,-2.61722529272117,
30.6712221069152)) ;
#63236=CARTESIAN_POINT('Ctrl Pts',(-6.7500010532002,-2.51779041441006,30.6512057681838)) ;
#63237=CARTESIAN_POINT('Ctrl Pts',(-6.74842826525773,-2.48426007770124,
30.6444567327798)) ;
#63238=CARTESIAN_POINT('Ctrl Pts',(-6.74525663369543,-2.41681407151976,
30.6308828583998)) ;
#63239=CARTESIAN_POINT('Ctrl Pts',(-6.74365780749008,-2.38289840200156,
30.6240580155811)) ;
#63240=CARTESIAN_POINT('Ctrl Pts',(-6.74044927101749,-2.31506715407992,
30.6104107449871)) ;
#63241=CARTESIAN_POINT('Ctrl Pts',(-6.73883960450799,-2.28115158934011,
30.6035883104715)) ;
#63242=CARTESIAN_POINT('Ctrl Pts',(-6.7364270630604,-2.23056738391237,30.5934154118563)) ;
#63243=CARTESIAN_POINT('Ctrl Pts',(-6.7356231912688,-2.2137541724559,30.5900345750881)) ;
#63244=CARTESIAN_POINT('Ctrl Pts',(-6.73401741621857,-2.18027230673386,
30.583303057464)) ;
#63245=CARTESIAN_POINT('Ctrl Pts',(-6.73321551517332,-2.16360365246034,
30.5799523761197)) ;
#63246=CARTESIAN_POINT('Ctrl Pts',(-6.73161460492591,-2.13045907910981,
30.5732911608798)) ;
#63247=CARTESIAN_POINT('Ctrl Pts',(-6.73081561316648,-2.11398316387167,
30.5699806239572)) ;
#63248=CARTESIAN_POINT('Ctrl Pts',(-6.72922064598632,-2.0812722502858,30.5634098657098)) ;
#63249=CARTESIAN_POINT('Ctrl Pts',(-6.72842471756409,-2.06503725173321,
30.5601496339967)) ;
#63250=CARTESIAN_POINT('Ctrl Pts',(-6.727231897208,-2.04090157756323,30.5553049316637)) ;
#63251=CARTESIAN_POINT('Ctrl Pts',(-6.72683444433809,-2.03289249098137,
30.5536976440673)) ;
#63252=CARTESIAN_POINT('Ctrl Pts',(-6.72603928498888,-2.01695261722727,
30.5504996933498)) ;
#63253=CARTESIAN_POINT('Ctrl Pts',(-6.72564157932666,-2.00902183005043,
30.5489090300484)) ;
#63254=CARTESIAN_POINT('Ctrl Pts',(-6.72484481412258,-1.9932445811914,30.5457458452672)) ;
#63255=CARTESIAN_POINT('Ctrl Pts',(-6.72444578254945,-1.98539811968377,
30.544173317668)) ;
#63256=CARTESIAN_POINT('Ctrl Pts',(-6.72384458439613,-1.97369619580611,
30.5418294499734)) ;
#63257=CARTESIAN_POINT('Ctrl Pts',(-6.72364373167107,-1.96980684934784,
30.5410506505884)) ;
#63258=CARTESIAN_POINT('Ctrl Pts',(-6.72324062165561,-1.9620515015343,30.5394983009585)) ;
#63259=CARTESIAN_POINT('Ctrl Pts',(-6.72303836614614,-1.95818550016552,
30.5387247503189)) ;
#63260=CARTESIAN_POINT('Ctrl Pts',(-6.72263139013325,-1.95047267002259,
30.5371822486687)) ;
#63261=CARTESIAN_POINT('Ctrl Pts',(-6.7224158750706,-1.9464209124257,30.5363723094797)) ;
#63262=CARTESIAN_POINT('Ctrl Pts',(-6.72196854648401,-1.93812468628743,
30.5347152398046)) ;
#63263=CARTESIAN_POINT('Ctrl Pts',(-6.72173680408808,-1.93388021706691,
30.5338680935183)) ;
#63264=CARTESIAN_POINT('Ctrl Pts',(-6.72138120528657,-1.92751377613103,
30.5325991873962)) ;
#63265=CARTESIAN_POINT('Ctrl Pts',(-6.72126132591748,-1.9253916862349,30.5321765271407)) ;
#63266=CARTESIAN_POINT('Ctrl Pts',(-6.72101902704608,-1.92117173550713,
30.5313368927791)) ;
#63267=CARTESIAN_POINT('Ctrl Pts',(-6.72089664243418,-1.91907387421947,
30.5309199108966)) ;
#63268=CARTESIAN_POINT('Ctrl Pts',(-6.72071053717591,-1.91596334990232,
30.5303026690603)) ;
#63269=CARTESIAN_POINT('Ctrl Pts',(-6.72064806954126,-1.91493255687844,
30.5300982968757)) ;
#63270=CARTESIAN_POINT('Ctrl Pts',(-6.72052191423922,-1.91288608064014,
30.5296930183877)) ;
#63271=CARTESIAN_POINT('Ctrl Pts',(-6.72045822910459,-1.91187039738182,
30.5294921115175)) ;
#63272=CARTESIAN_POINT('Ctrl Pts',(-6.72032886046213,-1.90985716099034,
30.5290945741019)) ;
#63273=CARTESIAN_POINT('Ctrl Pts',(-6.7202632152564,-1.90885960968473,30.5288979355123)) ;
#63274=CARTESIAN_POINT('Ctrl Pts',(-6.72016182003858,-1.90737915954795,
30.5286069816358)) ;
#63275=CARTESIAN_POINT('Ctrl Pts',(-6.72012752413129,-1.90688832280964,
30.5285106665645)) ;
#63276=CARTESIAN_POINT('Ctrl Pts',(-6.72005735934882,-1.90591232896256,
30.5283195845042)) ;
#63277=CARTESIAN_POINT('Ctrl Pts',(-6.72002151396779,-1.90542717120432,
30.5282248122061)) ;
#63278=CARTESIAN_POINT('Ctrl Pts',(-6.7199651260212,-1.90469706871886,30.5280827298087)) ;
#63279=CARTESIAN_POINT('Ctrl Pts',(-6.71994458374831,-1.9044367396773,30.5280321642263)) ;
#63280=CARTESIAN_POINT('Ctrl Pts',(-6.71990103088977,-1.90390388653279,
30.5279289958257)) ;
#63281=CARTESIAN_POINT('Ctrl Pts',(-6.71987802529109,-1.90363136224242,
30.5278763918702)) ;
#63282=CARTESIAN_POINT('Ctrl Pts',(-6.7198293861869,-1.90308662648624,30.5277718286008)) ;
#63283=CARTESIAN_POINT('Ctrl Pts',(-6.71980384794353,-1.90281445382391,
30.5277198565293)) ;
#63284=CARTESIAN_POINT('Ctrl Pts',(-6.71962399593059,-1.90163369887425,
30.5275095897043)) ;
#63285=CARTESIAN_POINT('Ctrl Pts',(-6.7196165808276,-1.90158501763117,30.5275009206317)) ;
#63286=CARTESIAN_POINT('Ctrl Pts',(-6.71960916572461,-1.9015363363881,30.527492251559)) ;
#63287=CARTESIAN_POINT('Origin',(-2.46380912372341E-16,-1.34123521733712,
0.)) ;
#63288=CARTESIAN_POINT('',(1.65824532362911E-15,-1.55431223447522E-15,-27.082990178354)) ;
#63289=CARTESIAN_POINT('Origin',(-3.0463484597791E-31,-1.65835486166302E-15,
0.)) ;
#63290=CARTESIAN_POINT('',(-5.46782640973375E-15,-2.68247043467423,-27.082990178354)) ;
#63291=CARTESIAN_POINT('',(-5.22144549736141E-15,-1.34123521733712,-27.082990178354)) ;
#63292=CARTESIAN_POINT('Origin',(-4.92761824744681E-16,-2.68247043467423,
0.)) ;
#63293=CARTESIAN_POINT('Origin',(-3.49024337756996E-15,-19.,0.)) ;
#63294=CARTESIAN_POINT('',(-7.96115465959473E-16,-20.,-23.5)) ;
#63295=CARTESIAN_POINT('Origin',(-3.67394039744206E-15,-20.,0.)) ;
#63296=CARTESIAN_POINT('',(-2.11260673051038E-15,-19.,-22.5)) ;
#63297=CARTESIAN_POINT('Origin',(-6.36816335556624E-15,-19.,-23.5)) ;
#63298=CARTESIAN_POINT('Origin',(-3.49024337756996E-15,-19.,0.)) ;
#63299=CARTESIAN_POINT('Origin',(-1.83697019872104E-16,-1.,0.)) ;
#63300=CARTESIAN_POINT('',(4.46981319145168E-15,-2.22044604925031E-15,-36.5)) ;
#63301=CARTESIAN_POINT('Origin',(-4.10559240503683E-31,-2.23498040844392E-15,
0.)) ;
#63302=CARTESIAN_POINT('',(2.11236405856052E-15,-1.,-37.5)) ;
#63303=CARTESIAN_POINT('Origin',(-4.65365783675994E-15,-1.,-36.5)) ;
#63304=CARTESIAN_POINT('Origin',(-1.83697019872103E-16,-1.,0.)) ;
#63305=CARTESIAN_POINT('Origin',(-2.80137955304957E-15,-15.25,0.)) ;
#63306=CARTESIAN_POINT('',(-5.05318474616943E-16,-15.25,-37.5)) ;
#63307=CARTESIAN_POINT('Origin',(-2.80137955304957E-15,-15.25,0.)) ;
#63308=CARTESIAN_POINT('',(1.71435485997076E-15,-15.5,-37.25)) ;
#63309=CARTESIAN_POINT('Origin',(-7.36318887987346E-15,-15.25,-37.25)) ;
#63310=CARTESIAN_POINT('Origin',(-2.8473038080176E-15,-15.5,0.)) ;
#63311=CARTESIAN_POINT('Origin',(-1.76808381626899E-15,-9.625,0.)) ;
#63312=CARTESIAN_POINT('',(2.70944004113232E-15,-0.250000000000001,-22.5)) ;
#63313=CARTESIAN_POINT('',(-5.90126676339131E-15,-9.625,-22.5)) ;
#63314=CARTESIAN_POINT('Origin',(-4.59242549680259E-17,-0.250000000000001,
0.)) ;
#63315=CARTESIAN_POINT('Origin',(-4.59242549680255E-17,-0.249999999999999,
0.)) ;
#63316=CARTESIAN_POINT('',(2.78597945494591E-15,-8.60422844084497E-16,-22.75)) ;
#63317=CARTESIAN_POINT('Origin',(-2.83199572302825E-15,-0.249999999999999,
-22.75)) ;
#63318=CARTESIAN_POINT('Origin',(-1.58419846794218E-31,-8.62397478764305E-16,
0.)) ;
#63319=CARTESIAN_POINT('Origin',(-1.49253828646084E-15,-8.125,0.)) ;
#63320=CARTESIAN_POINT('',(-8.3811765316647E-15,-8.125,-37.5)) ;
#63321=CARTESIAN_POINT('Origin',(1.52569529784657E-15,-1.26037617021366E-15,
24.916495089177)) ;
#63322=CARTESIAN_POINT('Origin',(-6.63803155591999E-16,-15.5,35.6592717826207)) ;
#63323=CARTESIAN_POINT('Origin',(2.06246819519177E-15,-2.06246819519177E-15,
33.6826617540297)) ;
#63324=CARTESIAN_POINT('Origin',(-3.58514725819224E-16,-2.169721598032,
29.82442706361)) ;
#63325=CARTESIAN_POINT('Origin',(-4.47836258798674E-16,-2.43790704449357,
28.3905603778595)) ;
#63326=CARTESIAN_POINT('Origin',(-4.47836258798674E-16,-2.43790704449357,
28.3905603778595)) ;
#63327=CARTESIAN_POINT('Origin',(-6.41137021490582,-2.169721598032,29.1271485325977)) ;
#63328=CARTESIAN_POINT('Origin',(-6.10313126226612,-2.43790704449357,27.7268048531459)) ;
#63329=CARTESIAN_POINT('Origin',(-6.10313126226612,-2.43790704449357,27.7268048531459)) ;
#63330=CARTESIAN_POINT('Origin',(-12.5229518842888,-2.169721598032,27.0679169087017)) ;
#63331=CARTESIAN_POINT('Origin',(-11.9208868898519,-2.43790704449357,25.7665747496295)) ;
#63332=CARTESIAN_POINT('Origin',(-11.9208868898519,-2.43790704449357,25.7665747496295)) ;
#63333=CARTESIAN_POINT('Origin',(-18.0489742418239,-2.169721598032,23.7430195739836)) ;
#63334=CARTESIAN_POINT('Origin',(-17.1812350955823,-2.43790704449357,22.6015282483114)) ;
#63335=CARTESIAN_POINT('Origin',(-17.1812350955823,-2.43790704449357,22.6015282483114)) ;
#63336=CARTESIAN_POINT('Origin',(-22.7310466238053,-2.169721598032,19.3079250324571)) ;
#63337=CARTESIAN_POINT('Origin',(-21.6382078438147,-2.43790704449357,18.3796594058966)) ;
#63338=CARTESIAN_POINT('Origin',(-21.6382078438147,-2.43790704449357,18.3796594058966)) ;
#63339=CARTESIAN_POINT('Origin',(-26.3502405294014,-2.169721598032,13.9700133756302)) ;
#63340=CARTESIAN_POINT('Origin',(-25.0834020424109,-2.43790704449357,13.2983781171864)) ;
#63341=CARTESIAN_POINT('Origin',(-25.0834020424109,-2.43790704449357,13.2983781171864)) ;
#63342=CARTESIAN_POINT('Origin',(-28.7373264740315,-2.169721598032,7.97887941991351)) ;
#63343=CARTESIAN_POINT('Origin',(-27.3557242397031,-2.43790704449357,7.59527944780228)) ;
#63344=CARTESIAN_POINT('Origin',(-27.3557242397031,-2.43790704449357,7.59527944780228)) ;
#63345=CARTESIAN_POINT('Origin',(-29.7806869719803,-2.169721598032,1.61466193040923)) ;
#63346=CARTESIAN_POINT('Origin',(-28.3489231752505,-2.43790704449357,1.53703395298571)) ;
#63347=CARTESIAN_POINT('Origin',(-28.3489231752505,-2.43790704449357,1.53703395298571)) ;
#63348=CARTESIAN_POINT('Origin',(-29.4315356459756,-2.169721598032,-4.82505535639315)) ;
#63349=CARTESIAN_POINT('Origin',(-28.0165579706883,-2.43790704449357,-4.59308154118194)) ;
#63350=CARTESIAN_POINT('Origin',(-28.0165579706883,-2.43790704449357,-4.59308154118194)) ;
#63351=CARTESIAN_POINT('Origin',(-27.7061984239676,-2.169721598032,-11.0391584173944)) ;
#63352=CARTESIAN_POINT('Origin',(-26.3741696535845,-2.43790704449357,-10.5084296473274)) ;
#63353=CARTESIAN_POINT('Origin',(-26.3741696535845,-2.43790704449357,-10.5084296473274)) ;
#63354=CARTESIAN_POINT('Origin',(-24.6853501568826,-2.169721598032,-16.7370826999417)) ;
#63355=CARTESIAN_POINT('Origin',(-23.4985544762632,-2.43790704449357,-15.9324152624445)) ;
#63356=CARTESIAN_POINT('Origin',(-23.4985544762632,-2.43790704449357,-15.9324152624445)) ;
#63357=CARTESIAN_POINT('Origin',(-20.510242352258,-2.169721598032,-21.6523995973711)) ;
#63358=CARTESIAN_POINT('Origin',(-19.5241730083994,-2.43790704449357,-20.6114188474975)) ;
#63359=CARTESIAN_POINT('Origin',(-19.5241730083994,-2.43790704449357,-20.6114188474975)) ;
#63360=CARTESIAN_POINT('Origin',(-15.3760984107389,-2.169721598032,-25.5552743545411)) ;
#63361=CARTESIAN_POINT('Origin',(-14.6368629102226,-2.43790704449357,-24.3266553951882)) ;
#63362=CARTESIAN_POINT('Origin',(-14.6368629102226,-2.43790704449357,-24.3266553951882)) ;
#63363=CARTESIAN_POINT('Origin',(-9.52298519683959,-2.169721598032,-28.2632128855402)) ;
#63364=CARTESIAN_POINT('Origin',(-9.06514937006846,-2.43790704449357,-26.9044045737354)) ;
#63365=CARTESIAN_POINT('Origin',(-9.06514937006846,-2.43790704449357,-26.9044045737354)) ;
#63366=CARTESIAN_POINT('Origin',(-3.22458777917394,-2.169721598032,-29.6495949943164)) ;
#63367=CARTESIAN_POINT('Origin',(-3.0695595205598,-2.43790704449357,-28.2241336965128)) ;
#63368=CARTESIAN_POINT('Origin',(-3.0695595205598,-2.43790704449357,-28.2241336965128)) ;
#63369=CARTESIAN_POINT('Origin',(3.22458777917398,-2.169721598032,-29.6495949943164)) ;
#63370=CARTESIAN_POINT('Origin',(3.06955952055985,-2.43790704449357,-28.2241336965128)) ;
#63371=CARTESIAN_POINT('Origin',(3.06955952055985,-2.43790704449357,-28.2241336965128)) ;
#63372=CARTESIAN_POINT('Origin',(9.52298519683963,-2.169721598032,-28.2632128855402)) ;
#63373=CARTESIAN_POINT('Origin',(9.0651493700685,-2.43790704449358,-26.9044045737354)) ;
#63374=CARTESIAN_POINT('Origin',(9.0651493700685,-2.43790704449358,-26.9044045737354)) ;
#63375=CARTESIAN_POINT('Origin',(15.3760984107389,-2.16972159803201,-25.5552743545411)) ;
#63376=CARTESIAN_POINT('Origin',(14.6368629102226,-2.43790704449358,-24.3266553951881)) ;
#63377=CARTESIAN_POINT('Origin',(14.6368629102226,-2.43790704449358,-24.3266553951881)) ;
#63378=CARTESIAN_POINT('Origin',(20.510242352258,-2.16972159803201,-21.6523995973711)) ;
#63379=CARTESIAN_POINT('Origin',(19.5241730083995,-2.43790704449358,-20.6114188474975)) ;
#63380=CARTESIAN_POINT('Origin',(19.5241730083995,-2.43790704449358,-20.6114188474975)) ;
#63381=CARTESIAN_POINT('Origin',(24.6853501568826,-2.16972159803201,-16.7370826999417)) ;
#63382=CARTESIAN_POINT('Origin',(23.4985544762633,-2.43790704449358,-15.9324152624445)) ;
#63383=CARTESIAN_POINT('Origin',(23.4985544762633,-2.43790704449358,-15.9324152624445)) ;
#63384=CARTESIAN_POINT('Origin',(27.7061984239676,-2.16972159803201,-11.0391584173944)) ;
#63385=CARTESIAN_POINT('Origin',(26.3741696535845,-2.43790704449358,-10.5084296473274)) ;
#63386=CARTESIAN_POINT('Origin',(26.3741696535845,-2.43790704449358,-10.5084296473274)) ;
#63387=CARTESIAN_POINT('Origin',(29.4315356459756,-2.16972159803201,-4.82505535639311)) ;
#63388=CARTESIAN_POINT('Origin',(28.0165579706883,-2.43790704449358,-4.5930815411819)) ;
#63389=CARTESIAN_POINT('Origin',(28.0165579706883,-2.43790704449358,-4.5930815411819)) ;
#63390=CARTESIAN_POINT('Origin',(29.7806869719803,-2.16972159803201,1.61466193040926)) ;
#63391=CARTESIAN_POINT('Origin',(28.3489231752505,-2.43790704449358,1.53703395298574)) ;
#63392=CARTESIAN_POINT('Origin',(28.3489231752505,-2.43790704449358,1.53703395298574)) ;
#63393=CARTESIAN_POINT('Origin',(28.7373264740315,-2.16972159803201,7.97887941991354)) ;
#63394=CARTESIAN_POINT('Origin',(27.3557242397031,-2.43790704449358,7.59527944780231)) ;
#63395=CARTESIAN_POINT('Origin',(27.3557242397031,-2.43790704449358,7.59527944780231)) ;
#63396=CARTESIAN_POINT('Origin',(26.3502405294014,-2.16972159803201,13.9700133756302)) ;
#63397=CARTESIAN_POINT('Origin',(25.0834020424109,-2.43790704449358,13.2983781171864)) ;
#63398=CARTESIAN_POINT('Origin',(25.0834020424109,-2.43790704449358,13.2983781171864)) ;
#63399=CARTESIAN_POINT('Origin',(22.7310466238053,-2.169721598032,19.3079250324571)) ;
#63400=CARTESIAN_POINT('Origin',(21.6382078438146,-2.43790704449357,18.3796594058967)) ;
#63401=CARTESIAN_POINT('Origin',(21.6382078438146,-2.43790704449357,18.3796594058967)) ;
#63402=CARTESIAN_POINT('Origin',(18.0489742418238,-2.16972159803201,23.7430195739837)) ;
#63403=CARTESIAN_POINT('Origin',(17.1812350955823,-2.43790704449358,22.6015282483114)) ;
#63404=CARTESIAN_POINT('Origin',(17.1812350955823,-2.43790704449358,22.6015282483114)) ;
#63405=CARTESIAN_POINT('Origin',(12.5229518842888,-2.169721598032,27.0679169087017)) ;
#63406=CARTESIAN_POINT('Origin',(11.9208868898518,-2.43790704449357,25.7665747496295)) ;
#63407=CARTESIAN_POINT('Origin',(11.9208868898518,-2.43790704449357,25.7665747496295)) ;
#63408=CARTESIAN_POINT('Origin',(-2.05716802131569E-15,-20.,26.4038966541541)) ;
#63409=CARTESIAN_POINT('Origin',(6.41137021490578,-2.169721598032,29.1271485325977)) ;
#63410=CARTESIAN_POINT('Origin',(6.10313126226608,-2.43790704449357,27.7268048531459)) ;
#63411=CARTESIAN_POINT('Origin',(6.10313126226608,-2.43790704449357,27.7268048531459)) ;
#63412=CARTESIAN_POINT('Origin',(-5.19563909059739E-16,-2.82837418604547,
0.)) ;
#63413=CARTESIAN_POINT('',(-5.35132983144392E-15,-2.82837418604547,-26.3029085923563)) ;
#63414=CARTESIAN_POINT('Origin',(-1.65855445878407E-15,-9.028749948904,
29.6232887510362)) ;
#63415=CARTESIAN_POINT('Origin',(-2.86927265876946E-15,-15.6195928533144,
30.8560171242128)) ;
#63416=CARTESIAN_POINT('Origin',(-2.86927265876946E-15,-15.6195928533144,
30.8560171242128)) ;
#63417=CARTESIAN_POINT('Origin',(-2.77219341593235E-15,-15.3281150963394,
32.4144172942372)) ;
#63418=CARTESIAN_POINT('Origin',(-2.86927265876946E-15,-15.6195928533144,
30.8560171242128)) ;
#63419=CARTESIAN_POINT('Origin',(-2.86927265876946E-15,-15.6195928533144,
30.8560171242128)) ;
#63420=CARTESIAN_POINT('Origin',(-1.65855445878407E-15,-9.028749948904,
29.6232887510362)) ;
#63421=CARTESIAN_POINT('Origin',(-6.36813142330852,-9.028749948904,28.9307127219973)) ;
#63422=CARTESIAN_POINT('Origin',(-6.63313158435093,-15.6195928533144,30.1346205908487)) ;
#63423=CARTESIAN_POINT('Origin',(-6.63313158435093,-15.6195928533144,30.1346205908487)) ;
#63424=CARTESIAN_POINT('Origin',(-6.968141554926,-15.3281150963394,31.6565862309166)) ;
#63425=CARTESIAN_POINT('Origin',(-6.63313158435093,-15.6195928533144,30.1346205908487)) ;
#63426=CARTESIAN_POINT('Origin',(-6.63313158435093,-15.6195928533144,30.1346205908487)) ;
#63427=CARTESIAN_POINT('Origin',(-6.36813142330852,-9.028749948904,28.9307127219973)) ;
#63428=CARTESIAN_POINT('Origin',(-12.4384960989329,-9.028749948904,26.8853687202556)) ;
#63429=CARTESIAN_POINT('Origin',(-12.9561053080139,-15.6195928533144,28.0041626908817)) ;
#63430=CARTESIAN_POINT('Origin',(-12.9561053080139,-15.6195928533144,28.0041626908817)) ;
#63431=CARTESIAN_POINT('Origin',(-13.6104605552768,-15.3281150963394,29.4185283792068)) ;
#63432=CARTESIAN_POINT('Origin',(-12.9561053080139,-15.6195928533144,28.0041626908817)) ;
#63433=CARTESIAN_POINT('Origin',(-12.9561053080139,-15.6195928533144,28.0041626908817)) ;
#63434=CARTESIAN_POINT('Origin',(-12.4384960989329,-9.028749948904,26.8853687202556)) ;
#63435=CARTESIAN_POINT('Origin',(-17.9272505213666,-9.02874994890399,23.5828947580959)) ;
#63436=CARTESIAN_POINT('Origin',(-18.6732659471509,-15.6195928533144,24.5642612678804)) ;
#63437=CARTESIAN_POINT('Origin',(-18.6732659471509,-15.6195928533144,24.5642612678804)) ;
#63438=CARTESIAN_POINT('Origin',(-19.6163695470032,-15.3281150963394,25.8048928368313)) ;
#63439=CARTESIAN_POINT('Origin',(-18.6732659471509,-15.6195928533144,24.5642612678804)) ;
#63440=CARTESIAN_POINT('Origin',(-18.6732659471509,-15.6195928533144,24.5642612678804)) ;
#63441=CARTESIAN_POINT('Origin',(-17.9272505213666,-9.02874994890399,23.5828947580959)) ;
#63442=CARTESIAN_POINT('Origin',(-22.5777466341291,-9.02874994890399,19.1777108475526)) ;
#63443=CARTESIAN_POINT('Origin',(-23.5172854244436,-15.6195928533144,19.9757622892086)) ;
#63444=CARTESIAN_POINT('Origin',(-23.5172854244436,-15.6195928533144,19.9757622892086)) ;
#63445=CARTESIAN_POINT('Origin',(-24.7050389007406,-15.3281150963394,20.984649185484)) ;
#63446=CARTESIAN_POINT('Origin',(-23.5172854244436,-15.6195928533144,19.9757622892086)) ;
#63447=CARTESIAN_POINT('Origin',(-23.5172854244436,-15.6195928533144,19.9757622892086)) ;
#63448=CARTESIAN_POINT('Origin',(-22.5777466341291,-9.02874994890399,19.1777108475526)) ;
#63449=CARTESIAN_POINT('Origin',(-26.1725324076428,-9.02874994890399,13.8757984922725)) ;
#63450=CARTESIAN_POINT('Origin',(-27.2616627728748,-15.6195928533144,14.4532188673586)) ;
#63451=CARTESIAN_POINT('Origin',(-27.2616627728748,-15.6195928533144,14.4532188673586)) ;
#63452=CARTESIAN_POINT('Origin',(-28.638528093158,-15.3281150963394,15.183186660986)) ;
#63453=CARTESIAN_POINT('Origin',(-27.2616627728748,-15.6195928533144,14.4532188673586)) ;
#63454=CARTESIAN_POINT('Origin',(-27.2616627728748,-15.6195928533144,14.4532188673586)) ;
#63455=CARTESIAN_POINT('Origin',(-26.1725324076428,-9.02874994890399,13.8757984922725)) ;
#63456=CARTESIAN_POINT('Origin',(-28.5435196544557,-9.02874994890399,7.92506922133606)) ;
#63457=CARTESIAN_POINT('Origin',(-29.7313150692083,-15.6195928533144,8.25485899486984)) ;
#63458=CARTESIAN_POINT('Origin',(-29.7313150692083,-15.6195928533144,8.25485899486984)) ;
#63459=CARTESIAN_POINT('Origin',(-31.2329115413772,-15.3281150963394,8.67177520312011)) ;
#63460=CARTESIAN_POINT('Origin',(-29.7313150692083,-15.6195928533144,8.25485899486984)) ;
#63461=CARTESIAN_POINT('Origin',(-29.7313150692083,-15.6195928533144,8.25485899486984)) ;
#63462=CARTESIAN_POINT('Origin',(-28.5435196544557,-9.02874994890399,7.92506922133606)) ;
#63463=CARTESIAN_POINT('Origin',(-29.5798436460697,-9.02874994890399,1.60377252169177)) ;
#63464=CARTESIAN_POINT('Origin',(-30.810764116889,-15.6195928533144,1.67051109039783)) ;
#63465=CARTESIAN_POINT('Origin',(-30.810764116889,-15.6195928533144,1.67051109039783)) ;
#63466=CARTESIAN_POINT('Origin',(-32.3668787588096,-15.3281150963394,1.75488117474228)) ;
#63467=CARTESIAN_POINT('Origin',(-30.810764116889,-15.6195928533144,1.67051109039783)) ;
#63468=CARTESIAN_POINT('Origin',(-30.810764116889,-15.6195928533144,1.67051109039783)) ;
#63469=CARTESIAN_POINT('Origin',(-29.5798436460697,-9.02874994890399,1.60377252169177)) ;
#63470=CARTESIAN_POINT('Origin',(-29.2330470244285,-9.02874994890399,-4.79251479860169)) ;
#63471=CARTESIAN_POINT('Origin',(-30.4495360781687,-15.6195928533144,-4.99194805602145)) ;
#63472=CARTESIAN_POINT('Origin',(-30.4495360781687,-15.6195928533144,-4.99194805602145)) ;
#63473=CARTESIAN_POINT('Origin',(-31.987406698682,-15.3281150963394,-5.24406914695616)) ;
#63474=CARTESIAN_POINT('Origin',(-30.4495360781687,-15.6195928533144,-4.99194805602145)) ;
#63475=CARTESIAN_POINT('Origin',(-30.4495360781687,-15.6195928533144,-4.99194805602145)) ;
#63476=CARTESIAN_POINT('Origin',(-29.2330470244285,-9.02874994890399,-4.79251479860169)) ;
#63477=CARTESIAN_POINT('Origin',(-27.5193456141232,-9.02874994890399,-10.9647094534102)) ;
#63478=CARTESIAN_POINT('Origin',(-28.664521574662,-15.6195928533144,-11.4209892594929)) ;
#63479=CARTESIAN_POINT('Origin',(-28.664521574662,-15.6195928533144,-11.4209892594929)) ;
#63480=CARTESIAN_POINT('Origin',(-30.1122390527731,-15.3281150963394,-11.9978126237072)) ;
#63481=CARTESIAN_POINT('Origin',(-28.664521574662,-15.6195928533144,-11.4209892594929)) ;
#63482=CARTESIAN_POINT('Origin',(-28.664521574662,-15.6195928533144,-11.4209892594929)) ;
#63483=CARTESIAN_POINT('Origin',(-27.5193456141232,-9.02874994890399,-10.9647094534102)) ;
#63484=CARTESIAN_POINT('Origin',(-24.5188701884574,-9.028749948904,-16.6242064805765)) ;
#63485=CARTESIAN_POINT('Origin',(-25.5391859006516,-15.6195928533144,-17.3159976987084)) ;
#63486=CARTESIAN_POINT('Origin',(-25.5391859006516,-15.6195928533144,-17.3159976987084)) ;
#63487=CARTESIAN_POINT('Origin',(-26.8290565761066,-15.3281150963394,-18.1905517167846)) ;
#63488=CARTESIAN_POINT('Origin',(-25.5391859006516,-15.6195928533144,-17.3159976987084)) ;
#63489=CARTESIAN_POINT('Origin',(-25.5391859006516,-15.6195928533144,-17.3159976987084)) ;
#63490=CARTESIAN_POINT('Origin',(-24.5188701884574,-9.028749948904,-16.6242064805765)) ;
#63491=CARTESIAN_POINT('Origin',(-20.3719196435463,-9.028749948904,-21.5063740891895)) ;
#63492=CARTESIAN_POINT('Origin',(-21.2196662786931,-15.6195928533144,-22.4013293308814)) ;
#63493=CARTESIAN_POINT('Origin',(-21.2196662786931,-15.6195928533144,-22.4013293308814)) ;
#63494=CARTESIAN_POINT('Origin',(-22.2913772322959,-15.3281150963394,-23.5327208289314)) ;
#63495=CARTESIAN_POINT('Origin',(-21.2196662786931,-15.6195928533144,-22.4013293308814)) ;
#63496=CARTESIAN_POINT('Origin',(-21.2196662786931,-15.6195928533144,-22.4013293308814)) ;
#63497=CARTESIAN_POINT('Origin',(-20.3719196435463,-9.028749948904,-21.5063740891895)) ;
#63498=CARTESIAN_POINT('Origin',(-15.2724007778654,-9.028749948904,-25.38292754801)) ;
#63499=CARTESIAN_POINT('Origin',(-15.9079386455081,-15.6195928533144,-26.4391997008318)) ;
#63500=CARTESIAN_POINT('Origin',(-15.9079386455081,-15.6195928533144,-26.4391997008318)) ;
#63501=CARTESIAN_POINT('Origin',(-16.7113778641895,-15.3281150963394,-27.7745260698579)) ;
#63502=CARTESIAN_POINT('Origin',(-15.9079386455081,-15.6195928533144,-26.4391997008318)) ;
#63503=CARTESIAN_POINT('Origin',(-15.9079386455081,-15.6195928533144,-26.4391997008318)) ;
#63504=CARTESIAN_POINT('Origin',(-15.2724007778654,-9.028749948904,-25.38292754801)) ;
#63505=CARTESIAN_POINT('Origin',(-9.45876142586579,-9.028749948904,-28.0726035257833)) ;
#63506=CARTESIAN_POINT('Origin',(-9.85237348166313,-15.6195928533144,-29.2408024778311)) ;
#63507=CARTESIAN_POINT('Origin',(-9.85237348166313,-15.6195928533144,-29.2408024778311)) ;
#63508=CARTESIAN_POINT('Origin',(-10.3499730405161,-15.3281150963394,-30.7176253409266)) ;
#63509=CARTESIAN_POINT('Origin',(-9.85237348166313,-15.6195928533144,-29.2408024778311)) ;
#63510=CARTESIAN_POINT('Origin',(-9.85237348166313,-15.6195928533144,-29.2408024778311)) ;
#63511=CARTESIAN_POINT('Origin',(-9.45876142586579,-9.028749948904,-28.0726035257833)) ;
#63512=CARTESIAN_POINT('Origin',(-3.20284090225101,-9.028749948904,-29.4496357631488)) ;
#63513=CARTESIAN_POINT('Origin',(-3.33612228394221,-15.6195928533144,-30.6751378297849)) ;
#63514=CARTESIAN_POINT('Origin',(-3.33612228394221,-15.6195928533144,-30.6751378297849)) ;
#63515=CARTESIAN_POINT('Origin',(-3.50461498063695,-15.3281150963394,-32.2244025912419)) ;
#63516=CARTESIAN_POINT('Origin',(-3.33612228394221,-15.6195928533144,-30.6751378297849)) ;
#63517=CARTESIAN_POINT('Origin',(-3.33612228394221,-15.6195928533144,-30.6751378297849)) ;
#63518=CARTESIAN_POINT('Origin',(-3.20284090225101,-9.028749948904,-29.4496357631488)) ;
#63519=CARTESIAN_POINT('Origin',(3.20284090225105,-9.028749948904,-29.4496357631488)) ;
#63520=CARTESIAN_POINT('Origin',(3.33612228394225,-15.6195928533144,-30.6751378297849)) ;
#63521=CARTESIAN_POINT('Origin',(3.33612228394225,-15.6195928533144,-30.6751378297849)) ;
#63522=CARTESIAN_POINT('Origin',(3.50461498063699,-15.3281150963394,-32.2244025912419)) ;
#63523=CARTESIAN_POINT('Origin',(3.33612228394225,-15.6195928533144,-30.6751378297849)) ;
#63524=CARTESIAN_POINT('Origin',(3.33612228394225,-15.6195928533144,-30.6751378297849)) ;
#63525=CARTESIAN_POINT('Origin',(3.20284090225105,-9.028749948904,-29.4496357631488)) ;
#63526=CARTESIAN_POINT('Origin',(9.45876142586583,-9.028749948904,-28.0726035257833)) ;
#63527=CARTESIAN_POINT('Origin',(9.85237348166317,-15.6195928533144,-29.2408024778311)) ;
#63528=CARTESIAN_POINT('Origin',(9.85237348166317,-15.6195928533144,-29.2408024778311)) ;
#63529=CARTESIAN_POINT('Origin',(10.3499730405161,-15.3281150963394,-30.7176253409265)) ;
#63530=CARTESIAN_POINT('Origin',(9.85237348166317,-15.6195928533144,-29.2408024778311)) ;
#63531=CARTESIAN_POINT('Origin',(9.85237348166317,-15.6195928533144,-29.2408024778311)) ;
#63532=CARTESIAN_POINT('Origin',(9.45876142586583,-9.028749948904,-28.0726035257833)) ;
#63533=CARTESIAN_POINT('Origin',(15.2724007778654,-9.02874994890401,-25.3829275480099)) ;
#63534=CARTESIAN_POINT('Origin',(15.9079386455082,-15.6195928533144,-26.4391997008318)) ;
#63535=CARTESIAN_POINT('Origin',(15.9079386455082,-15.6195928533144,-26.4391997008318)) ;
#63536=CARTESIAN_POINT('Origin',(16.7113778641896,-15.3281150963394,-27.7745260698579)) ;
#63537=CARTESIAN_POINT('Origin',(15.9079386455082,-15.6195928533144,-26.4391997008318)) ;
#63538=CARTESIAN_POINT('Origin',(15.9079386455082,-15.6195928533144,-26.4391997008318)) ;
#63539=CARTESIAN_POINT('Origin',(15.2724007778654,-9.02874994890401,-25.3829275480099)) ;
#63540=CARTESIAN_POINT('Origin',(20.3719196435463,-9.02874994890401,-21.5063740891894)) ;
#63541=CARTESIAN_POINT('Origin',(21.2196662786931,-15.6195928533144,-22.4013293308814)) ;
#63542=CARTESIAN_POINT('Origin',(21.2196662786931,-15.6195928533144,-22.4013293308814)) ;
#63543=CARTESIAN_POINT('Origin',(22.291377232296,-15.3281150963394,-23.5327208289313)) ;
#63544=CARTESIAN_POINT('Origin',(21.2196662786931,-15.6195928533144,-22.4013293308814)) ;
#63545=CARTESIAN_POINT('Origin',(21.2196662786931,-15.6195928533144,-22.4013293308814)) ;
#63546=CARTESIAN_POINT('Origin',(20.3719196435463,-9.02874994890401,-21.5063740891894)) ;
#63547=CARTESIAN_POINT('Origin',(24.5188701884574,-9.02874994890401,-16.6242064805764)) ;
#63548=CARTESIAN_POINT('Origin',(25.5391859006516,-15.6195928533144,-17.3159976987084)) ;
#63549=CARTESIAN_POINT('Origin',(25.5391859006516,-15.6195928533144,-17.3159976987084)) ;
#63550=CARTESIAN_POINT('Origin',(26.8290565761066,-15.3281150963394,-18.1905517167846)) ;
#63551=CARTESIAN_POINT('Origin',(25.5391859006516,-15.6195928533144,-17.3159976987084)) ;
#63552=CARTESIAN_POINT('Origin',(25.5391859006516,-15.6195928533144,-17.3159976987084)) ;
#63553=CARTESIAN_POINT('Origin',(24.5188701884574,-9.02874994890401,-16.6242064805764)) ;
#63554=CARTESIAN_POINT('Origin',(27.5193456141232,-9.02874994890401,-10.9647094534101)) ;
#63555=CARTESIAN_POINT('Origin',(28.664521574662,-15.6195928533144,-11.4209892594929)) ;
#63556=CARTESIAN_POINT('Origin',(28.664521574662,-15.6195928533144,-11.4209892594929)) ;
#63557=CARTESIAN_POINT('Origin',(30.1122390527732,-15.3281150963394,-11.9978126237071)) ;
#63558=CARTESIAN_POINT('Origin',(28.664521574662,-15.6195928533144,-11.4209892594929)) ;
#63559=CARTESIAN_POINT('Origin',(28.664521574662,-15.6195928533144,-11.4209892594929)) ;
#63560=CARTESIAN_POINT('Origin',(27.5193456141232,-9.02874994890401,-10.9647094534101)) ;
#63561=CARTESIAN_POINT('Origin',(29.2330470244285,-9.02874994890401,-4.79251479860166)) ;
#63562=CARTESIAN_POINT('Origin',(30.4495360781687,-15.6195928533144,-4.99194805602142)) ;
#63563=CARTESIAN_POINT('Origin',(30.4495360781687,-15.6195928533144,-4.99194805602142)) ;
#63564=CARTESIAN_POINT('Origin',(31.987406698682,-15.3281150963394,-5.24406914695613)) ;
#63565=CARTESIAN_POINT('Origin',(30.4495360781687,-15.6195928533144,-4.99194805602142)) ;
#63566=CARTESIAN_POINT('Origin',(30.4495360781687,-15.6195928533144,-4.99194805602142)) ;
#63567=CARTESIAN_POINT('Origin',(29.2330470244285,-9.02874994890401,-4.79251479860166)) ;
#63568=CARTESIAN_POINT('Origin',(29.5798436460697,-9.02874994890401,1.6037725216918)) ;
#63569=CARTESIAN_POINT('Origin',(30.810764116889,-15.6195928533144,1.67051109039787)) ;
#63570=CARTESIAN_POINT('Origin',(30.810764116889,-15.6195928533144,1.67051109039787)) ;
#63571=CARTESIAN_POINT('Origin',(32.3668787588096,-15.3281150963394,1.75488117474232)) ;
#63572=CARTESIAN_POINT('Origin',(30.810764116889,-15.6195928533144,1.67051109039787)) ;
#63573=CARTESIAN_POINT('Origin',(30.810764116889,-15.6195928533144,1.67051109039787)) ;
#63574=CARTESIAN_POINT('Origin',(29.5798436460697,-9.02874994890401,1.6037725216918)) ;
#63575=CARTESIAN_POINT('Origin',(28.5435196544557,-9.02874994890401,7.92506922133609)) ;
#63576=CARTESIAN_POINT('Origin',(29.7313150692083,-15.6195928533144,8.25485899486987)) ;
#63577=CARTESIAN_POINT('Origin',(29.7313150692083,-15.6195928533144,8.25485899486987)) ;
#63578=CARTESIAN_POINT('Origin',(31.2329115413772,-15.3281150963394,8.67177520312015)) ;
#63579=CARTESIAN_POINT('Origin',(29.7313150692083,-15.6195928533144,8.25485899486987)) ;
#63580=CARTESIAN_POINT('Origin',(29.7313150692083,-15.6195928533144,8.25485899486987)) ;
#63581=CARTESIAN_POINT('Origin',(28.5435196544557,-9.02874994890401,7.92506922133609)) ;
#63582=CARTESIAN_POINT('Origin',(26.1725324076428,-9.02874994890401,13.8757984922725)) ;
#63583=CARTESIAN_POINT('Origin',(27.2616627728747,-15.6195928533144,14.4532188673586)) ;
#63584=CARTESIAN_POINT('Origin',(27.2616627728747,-15.6195928533144,14.4532188673586)) ;
#63585=CARTESIAN_POINT('Origin',(28.638528093158,-15.3281150963394,15.183186660986)) ;
#63586=CARTESIAN_POINT('Origin',(27.2616627728747,-15.6195928533144,14.4532188673586)) ;
#63587=CARTESIAN_POINT('Origin',(27.2616627728747,-15.6195928533144,14.4532188673586)) ;
#63588=CARTESIAN_POINT('Origin',(26.1725324076428,-9.02874994890401,13.8757984922725)) ;
#63589=CARTESIAN_POINT('Origin',(22.5777466341291,-9.028749948904,19.1777108475526)) ;
#63590=CARTESIAN_POINT('Origin',(23.5172854244436,-15.6195928533144,19.9757622892086)) ;
#63591=CARTESIAN_POINT('Origin',(23.5172854244436,-15.6195928533144,19.9757622892086)) ;
#63592=CARTESIAN_POINT('Origin',(24.7050389007406,-15.3281150963394,20.9846491854841)) ;
#63593=CARTESIAN_POINT('Origin',(23.5172854244436,-15.6195928533144,19.9757622892086)) ;
#63594=CARTESIAN_POINT('Origin',(23.5172854244436,-15.6195928533144,19.9757622892086)) ;
#63595=CARTESIAN_POINT('Origin',(22.5777466341291,-9.028749948904,19.1777108475526)) ;
#63596=CARTESIAN_POINT('Origin',(17.9272505213666,-9.028749948904,23.5828947580959)) ;
#63597=CARTESIAN_POINT('Origin',(18.6732659471508,-15.6195928533144,24.5642612678805)) ;
#63598=CARTESIAN_POINT('Origin',(18.6732659471508,-15.6195928533144,24.5642612678805)) ;
#63599=CARTESIAN_POINT('Origin',(19.6163695470032,-15.3281150963394,25.8048928368313)) ;
#63600=CARTESIAN_POINT('Origin',(18.6732659471508,-15.6195928533144,24.5642612678805)) ;
#63601=CARTESIAN_POINT('Origin',(18.6732659471508,-15.6195928533144,24.5642612678805)) ;
#63602=CARTESIAN_POINT('Origin',(17.9272505213666,-9.028749948904,23.5828947580959)) ;
#63603=CARTESIAN_POINT('Origin',(12.4384960989328,-9.028749948904,26.8853687202556)) ;
#63604=CARTESIAN_POINT('Origin',(12.9561053080138,-15.6195928533144,28.0041626908817)) ;
#63605=CARTESIAN_POINT('Origin',(12.9561053080138,-15.6195928533144,28.0041626908817)) ;
#63606=CARTESIAN_POINT('Origin',(13.6104605552767,-15.3281150963394,29.4185283792069)) ;
#63607=CARTESIAN_POINT('Origin',(12.9561053080138,-15.6195928533144,28.0041626908817)) ;
#63608=CARTESIAN_POINT('Origin',(12.9561053080138,-15.6195928533144,28.0041626908817)) ;
#63609=CARTESIAN_POINT('Origin',(12.4384960989328,-9.028749948904,26.8853687202556)) ;
#63610=CARTESIAN_POINT('Origin',(6.36813142330848,-9.028749948904,28.9307127219973)) ;
#63611=CARTESIAN_POINT('Origin',(6.63313158435088,-15.6195928533144,30.1346205908487)) ;
#63612=CARTESIAN_POINT('Origin',(6.63313158435088,-15.6195928533144,30.1346205908487)) ;
#63613=CARTESIAN_POINT('Origin',(6.96814155492595,-15.3281150963394,31.6565862309166)) ;
#63614=CARTESIAN_POINT('Origin',(6.63313158435088,-15.6195928533144,30.1346205908487)) ;
#63615=CARTESIAN_POINT('Origin',(6.63313158435088,-15.6195928533144,30.1346205908487)) ;
#63616=CARTESIAN_POINT('Origin',(6.36813142330848,-9.028749948904,28.9307127219973)) ;
#63803=UNCERTAINTY_MEASURE_WITH_UNIT(LENGTH_MEASURE(0.01),#63825,
'DISTANCE_ACCURACY_VALUE',
'Maximum model space distance between geometric entities at asserted c
onnectivities') ;
#63807=UNCERTAINTY_MEASURE_WITH_UNIT(LENGTH_MEASURE(0.01),#63825,
'DISTANCE_ACCURACY_VALUE',
'Maximum model space distance between geometric entities at asserted c
onnectivities') ;
#63820=(
GEOMETRIC_REPRESENTATION_CONTEXT(3)
GLOBAL_UNCERTAINTY_ASSIGNED_CONTEXT((#63803))
GLOBAL_UNIT_ASSIGNED_CONTEXT((#63825,#63827,#63828))
REPRESENTATION_CONTEXT('','3D')
) ;
#63824=(
GEOMETRIC_REPRESENTATION_CONTEXT(3)
GLOBAL_UNCERTAINTY_ASSIGNED_CONTEXT((#63807))
GLOBAL_UNIT_ASSIGNED_CONTEXT((#63825,#63827,#63828))
REPRESENTATION_CONTEXT('','3D')
) ;
#63825=(
LENGTH_UNIT()
NAMED_UNIT(*)
SI_UNIT(.MILLI.,.METRE.)
) ;
#63827=(
NAMED_UNIT(*)
PLANE_ANGLE_UNIT()
SI_UNIT($,.RADIAN.)
) ;
#63828=(
NAMED_UNIT(*)
SI_UNIT($,.STERADIAN.)
SOLID_ANGLE_UNIT()
) ;
#63841=SHAPE_DEFINITION_REPRESENTATION(#63857,#63890) ;
#63857=PRODUCT_DEFINITION_SHAPE('',$,#63907) ;
#63890=SHAPE_REPRESENTATION('',(#17272),#63820) ;
#63894=PRODUCT_DEFINITION_CONTEXT('part definition',#63944,'design') ;
#63907=PRODUCT_DEFINITION('Taper_Roller_Bearing','Taper_Roller_Bearing',
#63923,#63894) ;
#63923=PRODUCT_DEFINITION_FORMATION('',$,#63958) ;
#63944=APPLICATION_CONTEXT(
'Core Data for Automotive Mechanical Design Process') ;
#63945=PRODUCT_CONTEXT('part definition',#63944,'mechanical') ;
#63958=PRODUCT('Taper_Roller_Bearing','Taper_Roller_Bearing',$,(#63945)) ;
#63963=PRESENTATION_STYLE_ASSIGNMENT((#63968)) ;
#63968=SURFACE_STYLE_USAGE(.BOTH.,#63973) ;
#63973=SURFACE_SIDE_STYLE('',(#63978)) ;
#63978=SURFACE_STYLE_FILL_AREA(#63983) ;
#63983=FILL_AREA_STYLE('Opaque(160,160,160)',(#63988)) ;
#63988=FILL_AREA_STYLE_COLOUR('Opaque(160,160,160)',#63993) ;
#63993=COLOUR_RGB('Opaque(160,160,160)', 0.09019608, 0.27058824, 0.51372549) ;
ENDSEC;
END-ISO-10303-21;
